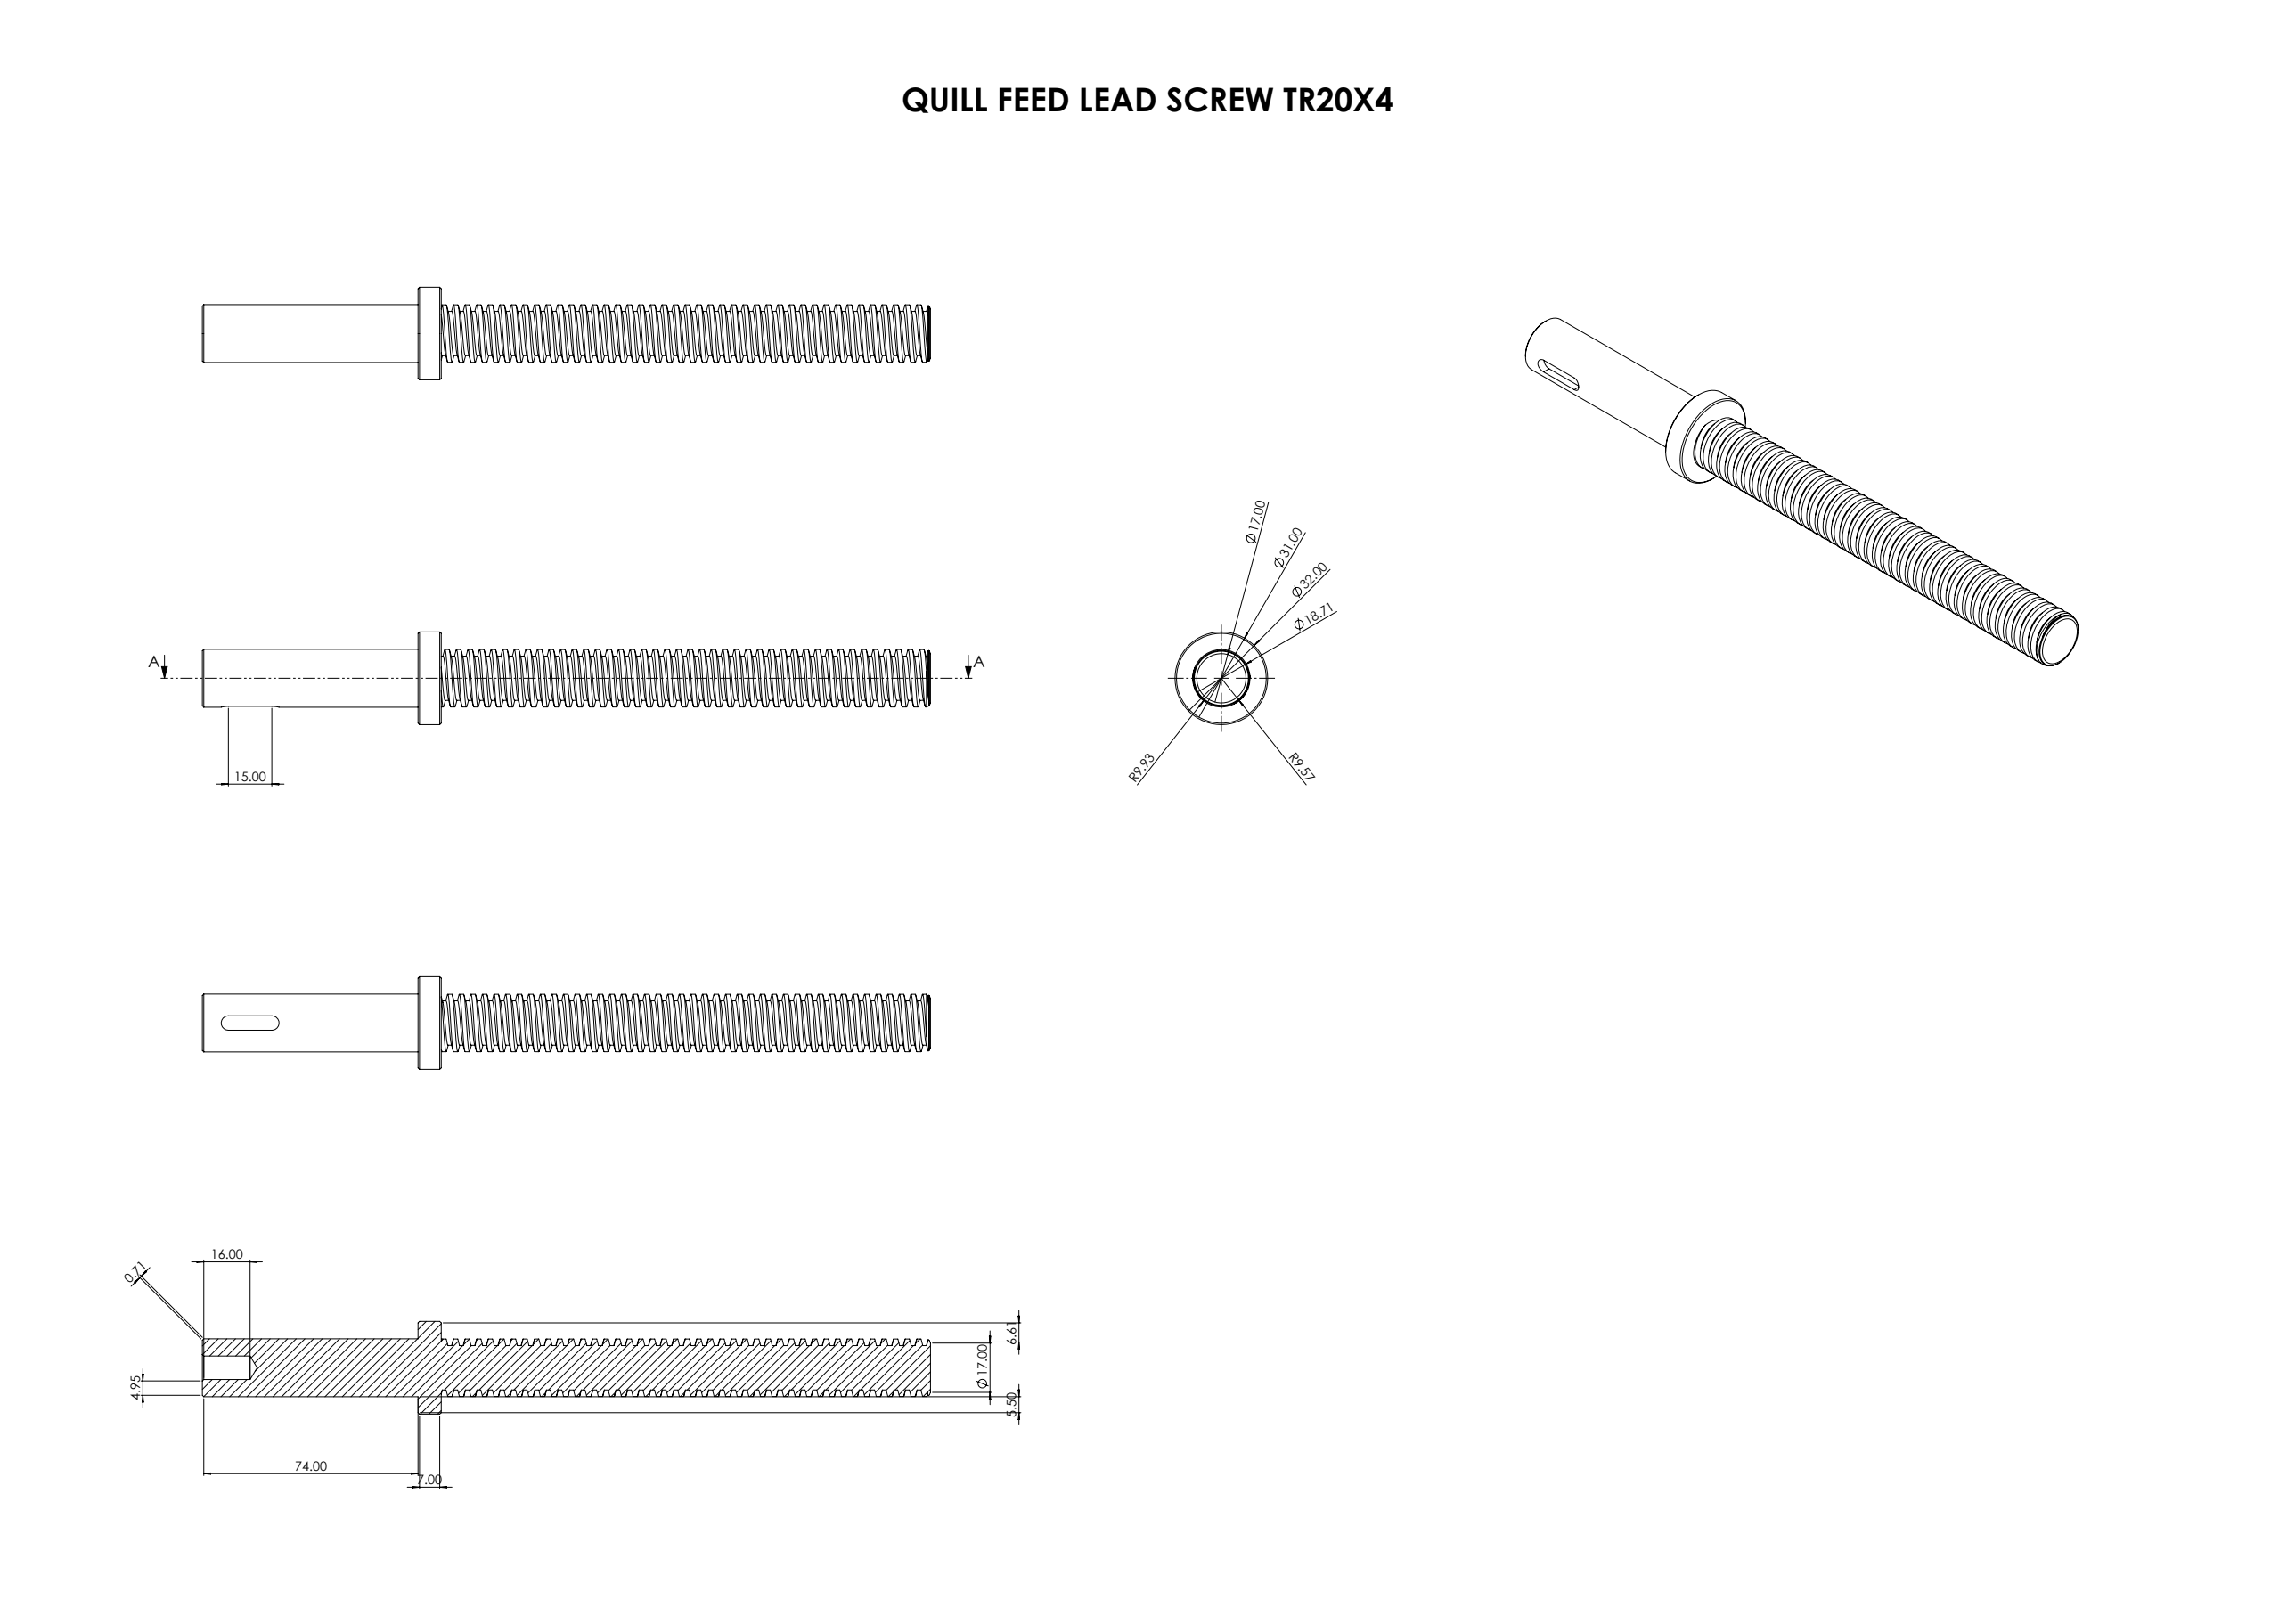
ISO-10303-21;
HEADER;
/* Generated by software containing ST-Developer
 * from STEP Tools, Inc. (www.steptools.com) 
 */

FILE_DESCRIPTION(
/* description */ (''),
/* implementation_level */ '2;1');

FILE_NAME(
/* name */ '05_Quill_Feed_Lead_Screw_Tr20x4.step',
/* time_stamp */ '2026-10-26T03:50:32-07:00',
/* author */ (''),
/* organization */ (''),
/* preprocessor_version */ 'ST-DEVELOPER v20.2',
/* originating_system */ 'Autodesk Translation Framework v15.15.0.0',
/* authorisation */ '');

FILE_SCHEMA (('AUTOMOTIVE_DESIGN { 1 0 10303 214 3 1 1 }'));
ENDSEC;

DATA;
#10=MECHANICAL_DESIGN_GEOMETRIC_PRESENTATION_REPRESENTATION('',(#1043),#76660);
#158=B_SPLINE_SURFACE_WITH_KNOTS('',3,3,((#45164,#45165,#45166,#45167,#45168,
#45169,#45170,#45171,#45172,#45173,#45174,#45175,#45176,#45177,#45178,#45179,
#45180,#45181,#45182,#45183,#45184,#45185,#45186,#45187,#45188,#45189,#45190,
#45191,#45192,#45193,#45194,#45195,#45196,#45197,#45198,#45199,#45200,#45201,
#45202,#45203,#45204,#45205,#45206,#45207,#45208,#45209,#45210,#45211,#45212,
#45213,#45214,#45215,#45216,#45217,#45218,#45219,#45220,#45221,#45222,#45223,
#45224,#45225,#45226,#45227,#45228,#45229,#45230,#45231,#45232,#45233,#45234,
#45235,#45236,#45237,#45238,#45239,#45240,#45241,#45242,#45243,#45244,#45245,
#45246,#45247,#45248,#45249,#45250,#45251,#45252,#45253,#45254,#45255,#45256,
#45257,#45258,#45259,#45260,#45261,#45262,#45263,#45264,#45265,#45266,#45267,
#45268,#45269,#45270,#45271,#45272,#45273,#45274,#45275,#45276,#45277,#45278,
#45279,#45280,#45281,#45282,#45283,#45284,#45285,#45286,#45287,#45288,#45289,
#45290,#45291,#45292,#45293,#45294,#45295,#45296,#45297,#45298,#45299,#45300,
#45301,#45302,#45303,#45304,#45305,#45306,#45307,#45308,#45309,#45310,#45311,
#45312,#45313,#45314,#45315,#45316,#45317,#45318,#45319,#45320,#45321,#45322,
#45323,#45324,#45325,#45326,#45327,#45328,#45329,#45330,#45331,#45332,#45333,
#45334,#45335,#45336,#45337,#45338,#45339,#45340,#45341,#45342,#45343,#45344,
#45345,#45346,#45347,#45348,#45349,#45350,#45351,#45352,#45353,#45354,#45355,
#45356,#45357,#45358,#45359,#45360,#45361,#45362,#45363,#45364,#45365,#45366,
#45367,#45368,#45369,#45370,#45371,#45372,#45373,#45374,#45375,#45376,#45377,
#45378,#45379,#45380,#45381,#45382,#45383,#45384,#45385,#45386,#45387,#45388,
#45389,#45390,#45391,#45392,#45393,#45394,#45395,#45396,#45397,#45398,#45399,
#45400,#45401,#45402,#45403,#45404,#45405,#45406,#45407,#45408,#45409,#45410,
#45411,#45412,#45413,#45414,#45415,#45416,#45417,#45418,#45419,#45420,#45421,
#45422,#45423,#45424,#45425,#45426,#45427,#45428,#45429,#45430,#45431,#45432,
#45433,#45434,#45435,#45436,#45437,#45438,#45439,#45440,#45441,#45442,#45443,
#45444,#45445,#45446,#45447,#45448,#45449,#45450,#45451,#45452,#45453,#45454,
#45455,#45456,#45457,#45458,#45459,#45460,#45461,#45462,#45463,#45464,#45465,
#45466,#45467,#45468,#45469,#45470,#45471,#45472,#45473,#45474,#45475,#45476,
#45477,#45478,#45479,#45480,#45481,#45482,#45483,#45484,#45485,#45486,#45487,
#45488,#45489,#45490,#45491,#45492,#45493,#45494,#45495,#45496,#45497,#45498,
#45499,#45500,#45501,#45502,#45503,#45504,#45505,#45506,#45507,#45508,#45509,
#45510,#45511,#45512,#45513,#45514,#45515,#45516,#45517,#45518,#45519,#45520,
#45521,#45522,#45523,#45524,#45525,#45526,#45527,#45528,#45529,#45530,#45531,
#45532,#45533,#45534,#45535,#45536,#45537,#45538,#45539,#45540,#45541,#45542,
#45543,#45544,#45545,#45546,#45547,#45548,#45549,#45550,#45551,#45552,#45553,
#45554,#45555,#45556,#45557,#45558,#45559,#45560,#45561,#45562,#45563,#45564,
#45565,#45566,#45567,#45568,#45569,#45570,#45571,#45572,#45573,#45574,#45575,
#45576,#45577,#45578,#45579,#45580,#45581,#45582,#45583,#45584,#45585,#45586,
#45587,#45588,#45589,#45590,#45591,#45592,#45593,#45594,#45595,#45596,#45597,
#45598,#45599,#45600,#45601,#45602,#45603,#45604,#45605,#45606,#45607,#45608,
#45609,#45610,#45611,#45612,#45613,#45614,#45615,#45616,#45617,#45618,#45619,
#45620,#45621,#45622,#45623,#45624,#45625,#45626,#45627,#45628,#45629,#45630,
#45631,#45632,#45633,#45634,#45635,#45636,#45637,#45638,#45639,#45640,#45641,
#45642,#45643,#45644,#45645,#45646,#45647,#45648,#45649,#45650,#45651,#45652,
#45653,#45654,#45655,#45656,#45657,#45658,#45659,#45660),(#45661,#45662,
#45663,#45664,#45665,#45666,#45667,#45668,#45669,#45670,#45671,#45672,#45673,
#45674,#45675,#45676,#45677,#45678,#45679,#45680,#45681,#45682,#45683,#45684,
#45685,#45686,#45687,#45688,#45689,#45690,#45691,#45692,#45693,#45694,#45695,
#45696,#45697,#45698,#45699,#45700,#45701,#45702,#45703,#45704,#45705,#45706,
#45707,#45708,#45709,#45710,#45711,#45712,#45713,#45714,#45715,#45716,#45717,
#45718,#45719,#45720,#45721,#45722,#45723,#45724,#45725,#45726,#45727,#45728,
#45729,#45730,#45731,#45732,#45733,#45734,#45735,#45736,#45737,#45738,#45739,
#45740,#45741,#45742,#45743,#45744,#45745,#45746,#45747,#45748,#45749,#45750,
#45751,#45752,#45753,#45754,#45755,#45756,#45757,#45758,#45759,#45760,#45761,
#45762,#45763,#45764,#45765,#45766,#45767,#45768,#45769,#45770,#45771,#45772,
#45773,#45774,#45775,#45776,#45777,#45778,#45779,#45780,#45781,#45782,#45783,
#45784,#45785,#45786,#45787,#45788,#45789,#45790,#45791,#45792,#45793,#45794,
#45795,#45796,#45797,#45798,#45799,#45800,#45801,#45802,#45803,#45804,#45805,
#45806,#45807,#45808,#45809,#45810,#45811,#45812,#45813,#45814,#45815,#45816,
#45817,#45818,#45819,#45820,#45821,#45822,#45823,#45824,#45825,#45826,#45827,
#45828,#45829,#45830,#45831,#45832,#45833,#45834,#45835,#45836,#45837,#45838,
#45839,#45840,#45841,#45842,#45843,#45844,#45845,#45846,#45847,#45848,#45849,
#45850,#45851,#45852,#45853,#45854,#45855,#45856,#45857,#45858,#45859,#45860,
#45861,#45862,#45863,#45864,#45865,#45866,#45867,#45868,#45869,#45870,#45871,
#45872,#45873,#45874,#45875,#45876,#45877,#45878,#45879,#45880,#45881,#45882,
#45883,#45884,#45885,#45886,#45887,#45888,#45889,#45890,#45891,#45892,#45893,
#45894,#45895,#45896,#45897,#45898,#45899,#45900,#45901,#45902,#45903,#45904,
#45905,#45906,#45907,#45908,#45909,#45910,#45911,#45912,#45913,#45914,#45915,
#45916,#45917,#45918,#45919,#45920,#45921,#45922,#45923,#45924,#45925,#45926,
#45927,#45928,#45929,#45930,#45931,#45932,#45933,#45934,#45935,#45936,#45937,
#45938,#45939,#45940,#45941,#45942,#45943,#45944,#45945,#45946,#45947,#45948,
#45949,#45950,#45951,#45952,#45953,#45954,#45955,#45956,#45957,#45958,#45959,
#45960,#45961,#45962,#45963,#45964,#45965,#45966,#45967,#45968,#45969,#45970,
#45971,#45972,#45973,#45974,#45975,#45976,#45977,#45978,#45979,#45980,#45981,
#45982,#45983,#45984,#45985,#45986,#45987,#45988,#45989,#45990,#45991,#45992,
#45993,#45994,#45995,#45996,#45997,#45998,#45999,#46000,#46001,#46002,#46003,
#46004,#46005,#46006,#46007,#46008,#46009,#46010,#46011,#46012,#46013,#46014,
#46015,#46016,#46017,#46018,#46019,#46020,#46021,#46022,#46023,#46024,#46025,
#46026,#46027,#46028,#46029,#46030,#46031,#46032,#46033,#46034,#46035,#46036,
#46037,#46038,#46039,#46040,#46041,#46042,#46043,#46044,#46045,#46046,#46047,
#46048,#46049,#46050,#46051,#46052,#46053,#46054,#46055,#46056,#46057,#46058,
#46059,#46060,#46061,#46062,#46063,#46064,#46065,#46066,#46067,#46068,#46069,
#46070,#46071,#46072,#46073,#46074,#46075,#46076,#46077,#46078,#46079,#46080,
#46081,#46082,#46083,#46084,#46085,#46086,#46087,#46088,#46089,#46090,#46091,
#46092,#46093,#46094,#46095,#46096,#46097,#46098,#46099,#46100,#46101,#46102,
#46103,#46104,#46105,#46106,#46107,#46108,#46109,#46110,#46111,#46112,#46113,
#46114,#46115,#46116,#46117,#46118,#46119,#46120,#46121,#46122,#46123,#46124,
#46125,#46126,#46127,#46128,#46129,#46130,#46131,#46132,#46133,#46134,#46135,
#46136,#46137,#46138,#46139,#46140,#46141,#46142,#46143,#46144,#46145,#46146,
#46147,#46148,#46149,#46150,#46151,#46152,#46153,#46154,#46155,#46156,#46157),
(#46158,#46159,#46160,#46161,#46162,#46163,#46164,#46165,#46166,#46167,
#46168,#46169,#46170,#46171,#46172,#46173,#46174,#46175,#46176,#46177,#46178,
#46179,#46180,#46181,#46182,#46183,#46184,#46185,#46186,#46187,#46188,#46189,
#46190,#46191,#46192,#46193,#46194,#46195,#46196,#46197,#46198,#46199,#46200,
#46201,#46202,#46203,#46204,#46205,#46206,#46207,#46208,#46209,#46210,#46211,
#46212,#46213,#46214,#46215,#46216,#46217,#46218,#46219,#46220,#46221,#46222,
#46223,#46224,#46225,#46226,#46227,#46228,#46229,#46230,#46231,#46232,#46233,
#46234,#46235,#46236,#46237,#46238,#46239,#46240,#46241,#46242,#46243,#46244,
#46245,#46246,#46247,#46248,#46249,#46250,#46251,#46252,#46253,#46254,#46255,
#46256,#46257,#46258,#46259,#46260,#46261,#46262,#46263,#46264,#46265,#46266,
#46267,#46268,#46269,#46270,#46271,#46272,#46273,#46274,#46275,#46276,#46277,
#46278,#46279,#46280,#46281,#46282,#46283,#46284,#46285,#46286,#46287,#46288,
#46289,#46290,#46291,#46292,#46293,#46294,#46295,#46296,#46297,#46298,#46299,
#46300,#46301,#46302,#46303,#46304,#46305,#46306,#46307,#46308,#46309,#46310,
#46311,#46312,#46313,#46314,#46315,#46316,#46317,#46318,#46319,#46320,#46321,
#46322,#46323,#46324,#46325,#46326,#46327,#46328,#46329,#46330,#46331,#46332,
#46333,#46334,#46335,#46336,#46337,#46338,#46339,#46340,#46341,#46342,#46343,
#46344,#46345,#46346,#46347,#46348,#46349,#46350,#46351,#46352,#46353,#46354,
#46355,#46356,#46357,#46358,#46359,#46360,#46361,#46362,#46363,#46364,#46365,
#46366,#46367,#46368,#46369,#46370,#46371,#46372,#46373,#46374,#46375,#46376,
#46377,#46378,#46379,#46380,#46381,#46382,#46383,#46384,#46385,#46386,#46387,
#46388,#46389,#46390,#46391,#46392,#46393,#46394,#46395,#46396,#46397,#46398,
#46399,#46400,#46401,#46402,#46403,#46404,#46405,#46406,#46407,#46408,#46409,
#46410,#46411,#46412,#46413,#46414,#46415,#46416,#46417,#46418,#46419,#46420,
#46421,#46422,#46423,#46424,#46425,#46426,#46427,#46428,#46429,#46430,#46431,
#46432,#46433,#46434,#46435,#46436,#46437,#46438,#46439,#46440,#46441,#46442,
#46443,#46444,#46445,#46446,#46447,#46448,#46449,#46450,#46451,#46452,#46453,
#46454,#46455,#46456,#46457,#46458,#46459,#46460,#46461,#46462,#46463,#46464,
#46465,#46466,#46467,#46468,#46469,#46470,#46471,#46472,#46473,#46474,#46475,
#46476,#46477,#46478,#46479,#46480,#46481,#46482,#46483,#46484,#46485,#46486,
#46487,#46488,#46489,#46490,#46491,#46492,#46493,#46494,#46495,#46496,#46497,
#46498,#46499,#46500,#46501,#46502,#46503,#46504,#46505,#46506,#46507,#46508,
#46509,#46510,#46511,#46512,#46513,#46514,#46515,#46516,#46517,#46518,#46519,
#46520,#46521,#46522,#46523,#46524,#46525,#46526,#46527,#46528,#46529,#46530,
#46531,#46532,#46533,#46534,#46535,#46536,#46537,#46538,#46539,#46540,#46541,
#46542,#46543,#46544,#46545,#46546,#46547,#46548,#46549,#46550,#46551,#46552,
#46553,#46554,#46555,#46556,#46557,#46558,#46559,#46560,#46561,#46562,#46563,
#46564,#46565,#46566,#46567,#46568,#46569,#46570,#46571,#46572,#46573,#46574,
#46575,#46576,#46577,#46578,#46579,#46580,#46581,#46582,#46583,#46584,#46585,
#46586,#46587,#46588,#46589,#46590,#46591,#46592,#46593,#46594,#46595,#46596,
#46597,#46598,#46599,#46600,#46601,#46602,#46603,#46604,#46605,#46606,#46607,
#46608,#46609,#46610,#46611,#46612,#46613,#46614,#46615,#46616,#46617,#46618,
#46619,#46620,#46621,#46622,#46623,#46624,#46625,#46626,#46627,#46628,#46629,
#46630,#46631,#46632,#46633,#46634,#46635,#46636,#46637,#46638,#46639,#46640,
#46641,#46642,#46643,#46644,#46645,#46646,#46647,#46648,#46649,#46650,#46651,
#46652,#46653,#46654),(#46655,#46656,#46657,#46658,#46659,#46660,#46661,
#46662,#46663,#46664,#46665,#46666,#46667,#46668,#46669,#46670,#46671,#46672,
#46673,#46674,#46675,#46676,#46677,#46678,#46679,#46680,#46681,#46682,#46683,
#46684,#46685,#46686,#46687,#46688,#46689,#46690,#46691,#46692,#46693,#46694,
#46695,#46696,#46697,#46698,#46699,#46700,#46701,#46702,#46703,#46704,#46705,
#46706,#46707,#46708,#46709,#46710,#46711,#46712,#46713,#46714,#46715,#46716,
#46717,#46718,#46719,#46720,#46721,#46722,#46723,#46724,#46725,#46726,#46727,
#46728,#46729,#46730,#46731,#46732,#46733,#46734,#46735,#46736,#46737,#46738,
#46739,#46740,#46741,#46742,#46743,#46744,#46745,#46746,#46747,#46748,#46749,
#46750,#46751,#46752,#46753,#46754,#46755,#46756,#46757,#46758,#46759,#46760,
#46761,#46762,#46763,#46764,#46765,#46766,#46767,#46768,#46769,#46770,#46771,
#46772,#46773,#46774,#46775,#46776,#46777,#46778,#46779,#46780,#46781,#46782,
#46783,#46784,#46785,#46786,#46787,#46788,#46789,#46790,#46791,#46792,#46793,
#46794,#46795,#46796,#46797,#46798,#46799,#46800,#46801,#46802,#46803,#46804,
#46805,#46806,#46807,#46808,#46809,#46810,#46811,#46812,#46813,#46814,#46815,
#46816,#46817,#46818,#46819,#46820,#46821,#46822,#46823,#46824,#46825,#46826,
#46827,#46828,#46829,#46830,#46831,#46832,#46833,#46834,#46835,#46836,#46837,
#46838,#46839,#46840,#46841,#46842,#46843,#46844,#46845,#46846,#46847,#46848,
#46849,#46850,#46851,#46852,#46853,#46854,#46855,#46856,#46857,#46858,#46859,
#46860,#46861,#46862,#46863,#46864,#46865,#46866,#46867,#46868,#46869,#46870,
#46871,#46872,#46873,#46874,#46875,#46876,#46877,#46878,#46879,#46880,#46881,
#46882,#46883,#46884,#46885,#46886,#46887,#46888,#46889,#46890,#46891,#46892,
#46893,#46894,#46895,#46896,#46897,#46898,#46899,#46900,#46901,#46902,#46903,
#46904,#46905,#46906,#46907,#46908,#46909,#46910,#46911,#46912,#46913,#46914,
#46915,#46916,#46917,#46918,#46919,#46920,#46921,#46922,#46923,#46924,#46925,
#46926,#46927,#46928,#46929,#46930,#46931,#46932,#46933,#46934,#46935,#46936,
#46937,#46938,#46939,#46940,#46941,#46942,#46943,#46944,#46945,#46946,#46947,
#46948,#46949,#46950,#46951,#46952,#46953,#46954,#46955,#46956,#46957,#46958,
#46959,#46960,#46961,#46962,#46963,#46964,#46965,#46966,#46967,#46968,#46969,
#46970,#46971,#46972,#46973,#46974,#46975,#46976,#46977,#46978,#46979,#46980,
#46981,#46982,#46983,#46984,#46985,#46986,#46987,#46988,#46989,#46990,#46991,
#46992,#46993,#46994,#46995,#46996,#46997,#46998,#46999,#47000,#47001,#47002,
#47003,#47004,#47005,#47006,#47007,#47008,#47009,#47010,#47011,#47012,#47013,
#47014,#47015,#47016,#47017,#47018,#47019,#47020,#47021,#47022,#47023,#47024,
#47025,#47026,#47027,#47028,#47029,#47030,#47031,#47032,#47033,#47034,#47035,
#47036,#47037,#47038,#47039,#47040,#47041,#47042,#47043,#47044,#47045,#47046,
#47047,#47048,#47049,#47050,#47051,#47052,#47053,#47054,#47055,#47056,#47057,
#47058,#47059,#47060,#47061,#47062,#47063,#47064,#47065,#47066,#47067,#47068,
#47069,#47070,#47071,#47072,#47073,#47074,#47075,#47076,#47077,#47078,#47079,
#47080,#47081,#47082,#47083,#47084,#47085,#47086,#47087,#47088,#47089,#47090,
#47091,#47092,#47093,#47094,#47095,#47096,#47097,#47098,#47099,#47100,#47101,
#47102,#47103,#47104,#47105,#47106,#47107,#47108,#47109,#47110,#47111,#47112,
#47113,#47114,#47115,#47116,#47117,#47118,#47119,#47120,#47121,#47122,#47123,
#47124,#47125,#47126,#47127,#47128,#47129,#47130,#47131,#47132,#47133,#47134,
#47135,#47136,#47137,#47138,#47139,#47140,#47141,#47142,#47143,#47144,#47145,
#47146,#47147,#47148,#47149,#47150,#47151)),.UNSPECIFIED.,.F.,.F.,.F.,(4,
4),(4,1,1,1,1,1,1,1,1,1,1,1,1,1,1,1,1,1,1,1,1,1,1,1,1,1,1,1,1,1,1,1,1,1,
1,1,1,1,1,1,1,1,1,1,1,1,1,1,1,1,1,1,1,1,1,1,1,1,1,1,1,1,1,1,1,1,1,1,1,1,
1,1,1,1,1,1,1,1,1,1,1,1,1,1,1,1,1,1,1,1,1,1,1,1,1,1,1,1,1,1,1,1,1,1,1,1,
1,1,1,1,1,1,1,1,1,1,1,1,1,1,1,1,1,1,1,1,1,1,1,1,1,1,1,1,1,1,1,1,1,1,1,1,
1,1,1,1,1,1,1,1,1,1,1,1,1,1,1,1,1,1,1,1,1,1,1,1,1,1,1,1,1,1,1,1,1,1,1,1,
1,1,1,1,1,1,1,1,1,1,1,1,1,1,1,1,1,1,1,1,1,1,1,1,1,1,1,1,1,1,1,1,1,1,1,1,
1,1,1,1,1,1,1,1,1,1,1,1,1,1,1,1,1,1,1,1,1,1,1,1,1,1,1,1,1,1,1,1,1,1,1,1,
1,1,1,1,1,1,1,1,1,1,1,1,1,1,1,1,1,1,1,1,1,1,1,1,1,1,1,1,1,1,1,1,1,1,1,1,
1,1,1,1,1,1,1,1,1,1,1,1,1,1,1,1,1,1,1,1,1,1,1,1,1,1,1,1,1,1,1,1,1,1,1,1,
1,1,1,1,1,1,1,1,1,1,1,1,1,1,1,1,1,1,1,1,1,1,1,1,1,1,1,1,1,1,1,1,1,1,1,1,
1,1,1,1,1,1,1,1,1,1,1,1,1,1,1,1,1,1,1,1,1,1,1,1,1,1,1,1,1,1,1,1,1,1,1,1,
1,1,1,1,1,1,1,1,1,1,1,1,1,1,1,1,1,1,1,1,1,1,1,1,1,1,1,1,1,1,1,1,1,1,1,1,
1,1,1,1,1,1,1,1,1,1,1,1,1,1,1,1,1,1,1,1,1,1,1,1,1,1,1,1,1,1,1,1,1,1,1,1,
1,1,1,1,1,1,1,1,1,1,1,1,1,1,1,1,1,1,1,1,1,1,1,1,1,1,1,1,4),(-1.54457385216123E-14,
0.236198260560645),(12.043305083964,12.5421366924057,13.0409683008475,13.5397999092893,
14.0386315177311,14.5374631261729,15.0362947346147,15.5351263430564,16.0339579514982,
17.0316211683818,17.5304527768236,18.0292843852654,18.5281159937072,19.0269476021489,
19.5257792105907,20.0246108190325,20.5234424274743,21.0222740359161,21.5211056443579,
22.0199372527997,22.5187688612414,23.0176004696832,24.0152636865668,24.5140952950086,
25.0129269034504,25.5117585118921,26.0105901203339,26.5094217287757,27.0082533372175,
27.5070849456593,28.0059165541011,28.5047481625429,29.0035797709846,29.5024113794264,
30.0012429878682,30.9989062047518,31.4977378131936,31.9965694216353,32.4954010300771,
32.9942326385189,33.4930642469607,33.9918958554025,34.4907274638443,34.9895590722861,
35.4883906807278,35.9872222891696,36.4860538976114,36.9848855060532,37.9825487229368,
38.4813803313785,38.9802119398203,39.4790435482621,39.9778751567039,40.4767067651457,
40.9755383735875,41.4743699820293,41.973201590471,42.4720331989128,42.9708648073546,
43.4696964157964,43.9685280242382,44.9661912411217,45.4650228495635,45.9638544580053,
46.4626860664471,46.9615176748889,47.4603492833307,47.9591808917725,48.4580125002142,
48.956844108656,49.4556757170978,49.9545073255396,50.4533389339814,50.9521705424232,
51.9498337593067,52.4486653677485,52.9474969761903,53.4463285846321,53.9451601930739,
54.4439918015157,54.9428234099574,55.4416550183992,55.940486626841,56.4393182352828,
56.9381498437246,57.4369814521664,57.9358130606082,58.9334762774917,59.4323078859335,
59.9311394943753,60.4299711028171,60.9288027112589,61.4276343197006,61.9264659281424,
62.4252975365842,62.924129145026,63.4229607534678,63.9217923619096,64.4206239703514,
64.9194555787931,65.9171187956767,66.4159504041185,66.9147820125603,67.4136136210021,
67.9124452294438,68.4112768378856,68.9101084463274,69.4089400547692,69.907771663211,
70.4066032716528,70.9054348800946,71.4042664885363,71.9030980969781,72.9007613138617,
73.3995929223035,73.8984245307453,74.397256139187,74.8960877476288,75.3949193560706,
75.8937509645124,76.3925825729542,76.891414181396,77.3902457898378,77.8890773982795,
78.3879090067213,78.8867406151631,79.8844038320467,80.3832354404885,80.8820670489303,
81.380898657372,81.8797302658138,82.3785618742556,82.8773934826974,83.3762250911392,
83.875056699581,84.3738883080227,84.8727199164645,85.3715515249063,85.8703831333481,
86.8680463502317,87.3668779586735,87.8657095671152,88.364541175557,88.8633727839988,
89.3622043924406,89.8610360008824,90.3598676093242,90.8586992177659,91.3575308262077,
91.8563624346495,92.3551940430913,92.8540256515331,93.8516888684167,94.3505204768584,
94.8493520853002,95.348183693742,95.8470153021838,96.3458469106256,96.8446785190674,
97.3435101275091,97.8423417359509,98.3411733443927,98.8400049528345,99.3388365612763,
99.8376681697181,100.835331386602,101.334162995043,101.832994603485,102.331826211927,
102.830657820369,103.329489428811,103.828321037252,104.327152645694,104.825984254136,
105.324815862578,105.823647471019,106.322479079461,106.821310687903,107.818973904787,
108.317805513228,108.81663712167,109.315468730112,109.814300338554,110.313131946996,
110.811963555437,111.310795163879,111.809626772321,112.308458380763,112.807289989204,
113.306121597646,113.804953206088,114.802616422972,115.301448031413,115.800279639855,
116.299111248297,116.797942856739,117.296774465181,117.795606073622,118.294437682064,
118.793269290506,119.292100898948,119.790932507389,120.289764115831,120.788595724273,
121.786258941157,122.285090549598,122.78392215804,123.282753766482,123.781585374924,
124.280416983366,124.779248591807,125.278080200249,125.776911808691,126.275743417133,
126.774575025574,127.273406634016,127.772238242458,128.769901459342,129.268733067783,
129.767564676225,130.266396284667,130.765227893109,131.26405950155,131.762891109992,
132.261722718434,132.760554326876,133.259385935318,133.758217543759,134.257049152201,
134.755880760643,135.753543977527,136.252375585968,136.75120719441,137.250038802852,
137.748870411294,138.247702019735,138.746533628177,139.245365236619,139.744196845061,
140.243028453503,140.741860061944,141.240691670386,141.739523278828,142.737186495712,
143.236018104153,143.734849712595,144.233681321037,144.732512929479,145.231344537921,
145.730176146362,146.229007754804,146.727839363246,147.725502580129,148.224334188571,
148.723165797013,149.221997405455,149.720829013897,150.219660622338,150.71849223078,
151.217323839222,151.716155447664,152.214987056105,152.713818664547,153.212650272989,
153.711481881431,154.709145098314,155.207976706756,155.706808315198,156.20563992364,
156.704471532082,157.203303140523,157.702134748965,158.200966357407,158.699797965849,
159.19862957429,159.697461182732,160.196292791174,160.695124399616,161.692787616499,
162.191619224941,162.690450833383,163.189282441825,163.688114050267,164.186945658708,
164.68577726715,165.184608875592,165.683440484034,166.182272092475,166.681103700917,
167.179935309359,167.678766917801,168.676430134684,169.175261743126,169.674093351568,
170.17292496001,170.671756568452,171.170588176893,171.669419785335,172.168251393777,
172.667083002219,173.16591461066,173.664746219102,174.163577827544,174.662409435986,
175.660072652869,176.158904261311,176.657735869753,177.156567478195,177.655399086636,
178.154230695078,178.65306230352,179.151893911962,179.650725520404,180.149557128845,
180.648388737287,181.147220345729,181.646051954171,182.643715171054,183.142546779496,
183.641378387938,184.14020999638,184.639041604821,185.137873213263,185.636704821705,
186.135536430147,186.634368038589,187.13319964703,187.632031255472,188.130862863914,
188.629694472356,189.627357689239,190.126189297681,190.625020906123,191.123852514565,
191.622684123006,192.121515731448,192.62034733989,193.119178948332,193.618010556774,
194.116842165215,194.615673773657,195.114505382099,195.613336990541,196.611000207424,
197.109831815866,197.608663424308,198.10749503275,198.606326641191,199.105158249633,
199.603989858075,200.102821466517,200.601653074959,201.1004846834,201.599316291842,
202.098147900284,202.596979508726,203.594642725609,204.093474334051,204.592305942493,
205.091137550935,205.589969159376,206.088800767818,206.58763237626,207.086463984702,
207.585295593144,208.084127201585,208.582958810027,209.081790418469,209.580622026911,
210.578285243794,211.077116852236,211.575948460678,212.07478006912,212.573611677561,
213.072443286003,213.571274894445,214.070106502887,214.568938111329,215.06776971977,
215.566601328212,216.065432936654,216.564264545096,217.561927761979,218.060759370421,
218.559590978863,219.058422587305,219.557254195746,220.056085804188,220.55491741263,
221.053749021072,221.552580629514,222.051412237955,222.550243846397,223.049075454839,
223.547907063281,224.545570280164,225.044401888606,225.543233497048,226.04206510549,
226.540896713931,227.039728322373,227.538559930815,228.037391539257,228.536223147699,
229.03505475614,229.533886364582,230.032717973024,230.531549581466,231.529212798349,
232.028044406791,232.526876015233,233.025707623675,233.524539232116,234.023370840558,
234.522202449,235.021034057442,235.519865665884,236.018697274325,236.517528882767,
237.016360491209,237.515192099651,238.512855316534,239.011686924976,239.510518533418,
240.00935014186,240.508181750301,241.007013358743,241.505844967185,242.004676575627,
242.503508184069,243.00233979251,243.501171400952,244.000003009394,244.498834617836,
245.496497834719,245.995329443161,246.494161051603,246.992992660045,247.491824268486,
247.990655876928,248.48948748537,248.988319093812,249.487150702254,249.985982310695,
250.484813919137,250.983645527579,251.482477136021,252.480140352904,252.978971961346,
253.477803569788,253.97663517823,254.475466786671,254.974298395113,255.473130003555,
255.971961611997,256.470793220438,256.96962482888,257.468456437322,257.967288045764,
258.466119654206,259.463782871089,259.962614479531,260.461446087973,260.960277696415,
261.459109304856,261.957940913298,262.45677252174,262.955604130182,263.454435738623,
263.953267347065,264.452098955507,264.950930563949,265.449762172391,266.447425389274,
266.946256997716,267.445088606158,267.9439202146,268.442751823041,268.941583431483,
269.440415039925,269.939246648367,270.438078256808,270.93690986525,271.435741473692,
271.934573082134,272.433404690576,273.431067907459,273.929899515901,274.428731124343,
274.927562732785,275.426394341226,275.925225949668,276.42405755811,276.922889166552,
277.421720774993),.UNSPECIFIED.);
#159=B_SPLINE_SURFACE_WITH_KNOTS('',3,3,((#47328,#47329,#47330,#47331,#47332,
#47333,#47334,#47335,#47336,#47337,#47338,#47339,#47340,#47341,#47342,#47343,
#47344,#47345,#47346,#47347,#47348,#47349,#47350,#47351,#47352,#47353,#47354,
#47355,#47356,#47357,#47358,#47359,#47360,#47361,#47362,#47363,#47364,#47365,
#47366,#47367,#47368,#47369,#47370,#47371,#47372,#47373,#47374,#47375,#47376,
#47377,#47378,#47379,#47380,#47381,#47382,#47383,#47384,#47385,#47386,#47387,
#47388,#47389,#47390,#47391,#47392,#47393,#47394,#47395,#47396,#47397,#47398,
#47399,#47400,#47401,#47402,#47403,#47404,#47405,#47406,#47407,#47408,#47409,
#47410,#47411,#47412,#47413,#47414,#47415,#47416,#47417,#47418,#47419,#47420,
#47421,#47422,#47423,#47424,#47425,#47426,#47427,#47428,#47429,#47430,#47431,
#47432,#47433,#47434,#47435,#47436,#47437,#47438,#47439,#47440,#47441,#47442,
#47443,#47444,#47445,#47446,#47447,#47448,#47449,#47450,#47451,#47452,#47453,
#47454,#47455,#47456,#47457,#47458,#47459,#47460,#47461,#47462,#47463,#47464,
#47465,#47466,#47467,#47468,#47469,#47470,#47471,#47472,#47473,#47474,#47475,
#47476,#47477,#47478,#47479,#47480,#47481,#47482,#47483,#47484,#47485,#47486,
#47487,#47488,#47489,#47490,#47491,#47492,#47493,#47494,#47495,#47496,#47497,
#47498,#47499,#47500,#47501,#47502,#47503,#47504,#47505,#47506,#47507,#47508,
#47509,#47510,#47511,#47512,#47513,#47514,#47515,#47516,#47517,#47518,#47519,
#47520,#47521,#47522,#47523,#47524,#47525,#47526,#47527,#47528,#47529,#47530,
#47531,#47532,#47533,#47534,#47535,#47536,#47537,#47538,#47539,#47540,#47541,
#47542,#47543,#47544,#47545,#47546,#47547,#47548,#47549,#47550,#47551,#47552,
#47553,#47554,#47555,#47556,#47557,#47558,#47559,#47560,#47561,#47562,#47563,
#47564,#47565,#47566,#47567,#47568,#47569,#47570,#47571,#47572,#47573,#47574,
#47575,#47576,#47577,#47578,#47579,#47580,#47581,#47582,#47583,#47584,#47585,
#47586,#47587,#47588,#47589,#47590,#47591,#47592,#47593,#47594,#47595,#47596,
#47597,#47598,#47599,#47600,#47601,#47602,#47603,#47604,#47605,#47606,#47607,
#47608,#47609,#47610,#47611,#47612,#47613,#47614,#47615,#47616,#47617,#47618,
#47619,#47620,#47621,#47622,#47623,#47624,#47625,#47626,#47627,#47628,#47629,
#47630,#47631,#47632,#47633,#47634,#47635,#47636,#47637,#47638,#47639,#47640,
#47641,#47642,#47643,#47644,#47645,#47646,#47647,#47648,#47649,#47650,#47651,
#47652,#47653,#47654,#47655,#47656,#47657,#47658,#47659,#47660,#47661,#47662,
#47663,#47664,#47665,#47666,#47667,#47668,#47669,#47670,#47671,#47672,#47673,
#47674,#47675,#47676,#47677,#47678,#47679,#47680,#47681,#47682,#47683,#47684,
#47685,#47686,#47687,#47688,#47689,#47690,#47691,#47692,#47693,#47694,#47695,
#47696,#47697,#47698,#47699,#47700,#47701,#47702,#47703,#47704,#47705,#47706,
#47707,#47708,#47709,#47710,#47711,#47712,#47713,#47714,#47715,#47716,#47717,
#47718,#47719,#47720,#47721,#47722,#47723,#47724,#47725,#47726,#47727,#47728,
#47729,#47730,#47731,#47732,#47733,#47734,#47735,#47736,#47737,#47738,#47739,
#47740,#47741,#47742,#47743,#47744,#47745,#47746,#47747,#47748,#47749,#47750,
#47751,#47752,#47753,#47754,#47755,#47756,#47757,#47758,#47759,#47760,#47761,
#47762,#47763,#47764,#47765,#47766,#47767,#47768,#47769,#47770,#47771,#47772,
#47773,#47774,#47775,#47776,#47777,#47778,#47779,#47780,#47781,#47782,#47783,
#47784,#47785,#47786,#47787,#47788,#47789,#47790,#47791,#47792,#47793,#47794,
#47795,#47796,#47797,#47798,#47799,#47800,#47801,#47802,#47803,#47804,#47805,
#47806,#47807,#47808,#47809,#47810,#47811,#47812,#47813,#47814,#47815,#47816,
#47817,#47818,#47819,#47820,#47821,#47822,#47823,#47824,#47825,#47826,#47827,
#47828,#47829,#47830,#47831,#47832,#47833,#47834,#47835,#47836,#47837,#47838,
#47839,#47840,#47841,#47842,#47843,#47844,#47845,#47846,#47847,#47848,#47849,
#47850,#47851,#47852,#47853,#47854,#47855,#47856,#47857,#47858),(#47859,
#47860,#47861,#47862,#47863,#47864,#47865,#47866,#47867,#47868,#47869,#47870,
#47871,#47872,#47873,#47874,#47875,#47876,#47877,#47878,#47879,#47880,#47881,
#47882,#47883,#47884,#47885,#47886,#47887,#47888,#47889,#47890,#47891,#47892,
#47893,#47894,#47895,#47896,#47897,#47898,#47899,#47900,#47901,#47902,#47903,
#47904,#47905,#47906,#47907,#47908,#47909,#47910,#47911,#47912,#47913,#47914,
#47915,#47916,#47917,#47918,#47919,#47920,#47921,#47922,#47923,#47924,#47925,
#47926,#47927,#47928,#47929,#47930,#47931,#47932,#47933,#47934,#47935,#47936,
#47937,#47938,#47939,#47940,#47941,#47942,#47943,#47944,#47945,#47946,#47947,
#47948,#47949,#47950,#47951,#47952,#47953,#47954,#47955,#47956,#47957,#47958,
#47959,#47960,#47961,#47962,#47963,#47964,#47965,#47966,#47967,#47968,#47969,
#47970,#47971,#47972,#47973,#47974,#47975,#47976,#47977,#47978,#47979,#47980,
#47981,#47982,#47983,#47984,#47985,#47986,#47987,#47988,#47989,#47990,#47991,
#47992,#47993,#47994,#47995,#47996,#47997,#47998,#47999,#48000,#48001,#48002,
#48003,#48004,#48005,#48006,#48007,#48008,#48009,#48010,#48011,#48012,#48013,
#48014,#48015,#48016,#48017,#48018,#48019,#48020,#48021,#48022,#48023,#48024,
#48025,#48026,#48027,#48028,#48029,#48030,#48031,#48032,#48033,#48034,#48035,
#48036,#48037,#48038,#48039,#48040,#48041,#48042,#48043,#48044,#48045,#48046,
#48047,#48048,#48049,#48050,#48051,#48052,#48053,#48054,#48055,#48056,#48057,
#48058,#48059,#48060,#48061,#48062,#48063,#48064,#48065,#48066,#48067,#48068,
#48069,#48070,#48071,#48072,#48073,#48074,#48075,#48076,#48077,#48078,#48079,
#48080,#48081,#48082,#48083,#48084,#48085,#48086,#48087,#48088,#48089,#48090,
#48091,#48092,#48093,#48094,#48095,#48096,#48097,#48098,#48099,#48100,#48101,
#48102,#48103,#48104,#48105,#48106,#48107,#48108,#48109,#48110,#48111,#48112,
#48113,#48114,#48115,#48116,#48117,#48118,#48119,#48120,#48121,#48122,#48123,
#48124,#48125,#48126,#48127,#48128,#48129,#48130,#48131,#48132,#48133,#48134,
#48135,#48136,#48137,#48138,#48139,#48140,#48141,#48142,#48143,#48144,#48145,
#48146,#48147,#48148,#48149,#48150,#48151,#48152,#48153,#48154,#48155,#48156,
#48157,#48158,#48159,#48160,#48161,#48162,#48163,#48164,#48165,#48166,#48167,
#48168,#48169,#48170,#48171,#48172,#48173,#48174,#48175,#48176,#48177,#48178,
#48179,#48180,#48181,#48182,#48183,#48184,#48185,#48186,#48187,#48188,#48189,
#48190,#48191,#48192,#48193,#48194,#48195,#48196,#48197,#48198,#48199,#48200,
#48201,#48202,#48203,#48204,#48205,#48206,#48207,#48208,#48209,#48210,#48211,
#48212,#48213,#48214,#48215,#48216,#48217,#48218,#48219,#48220,#48221,#48222,
#48223,#48224,#48225,#48226,#48227,#48228,#48229,#48230,#48231,#48232,#48233,
#48234,#48235,#48236,#48237,#48238,#48239,#48240,#48241,#48242,#48243,#48244,
#48245,#48246,#48247,#48248,#48249,#48250,#48251,#48252,#48253,#48254,#48255,
#48256,#48257,#48258,#48259,#48260,#48261,#48262,#48263,#48264,#48265,#48266,
#48267,#48268,#48269,#48270,#48271,#48272,#48273,#48274,#48275,#48276,#48277,
#48278,#48279,#48280,#48281,#48282,#48283,#48284,#48285,#48286,#48287,#48288,
#48289,#48290,#48291,#48292,#48293,#48294,#48295,#48296,#48297,#48298,#48299,
#48300,#48301,#48302,#48303,#48304,#48305,#48306,#48307,#48308,#48309,#48310,
#48311,#48312,#48313,#48314,#48315,#48316,#48317,#48318,#48319,#48320,#48321,
#48322,#48323,#48324,#48325,#48326,#48327,#48328,#48329,#48330,#48331,#48332,
#48333,#48334,#48335,#48336,#48337,#48338,#48339,#48340,#48341,#48342,#48343,
#48344,#48345,#48346,#48347,#48348,#48349,#48350,#48351,#48352,#48353,#48354,
#48355,#48356,#48357,#48358,#48359,#48360,#48361,#48362,#48363,#48364,#48365,
#48366,#48367,#48368,#48369,#48370,#48371,#48372,#48373,#48374,#48375,#48376,
#48377,#48378,#48379,#48380,#48381,#48382,#48383,#48384,#48385,#48386,#48387,
#48388,#48389),(#48390,#48391,#48392,#48393,#48394,#48395,#48396,#48397,
#48398,#48399,#48400,#48401,#48402,#48403,#48404,#48405,#48406,#48407,#48408,
#48409,#48410,#48411,#48412,#48413,#48414,#48415,#48416,#48417,#48418,#48419,
#48420,#48421,#48422,#48423,#48424,#48425,#48426,#48427,#48428,#48429,#48430,
#48431,#48432,#48433,#48434,#48435,#48436,#48437,#48438,#48439,#48440,#48441,
#48442,#48443,#48444,#48445,#48446,#48447,#48448,#48449,#48450,#48451,#48452,
#48453,#48454,#48455,#48456,#48457,#48458,#48459,#48460,#48461,#48462,#48463,
#48464,#48465,#48466,#48467,#48468,#48469,#48470,#48471,#48472,#48473,#48474,
#48475,#48476,#48477,#48478,#48479,#48480,#48481,#48482,#48483,#48484,#48485,
#48486,#48487,#48488,#48489,#48490,#48491,#48492,#48493,#48494,#48495,#48496,
#48497,#48498,#48499,#48500,#48501,#48502,#48503,#48504,#48505,#48506,#48507,
#48508,#48509,#48510,#48511,#48512,#48513,#48514,#48515,#48516,#48517,#48518,
#48519,#48520,#48521,#48522,#48523,#48524,#48525,#48526,#48527,#48528,#48529,
#48530,#48531,#48532,#48533,#48534,#48535,#48536,#48537,#48538,#48539,#48540,
#48541,#48542,#48543,#48544,#48545,#48546,#48547,#48548,#48549,#48550,#48551,
#48552,#48553,#48554,#48555,#48556,#48557,#48558,#48559,#48560,#48561,#48562,
#48563,#48564,#48565,#48566,#48567,#48568,#48569,#48570,#48571,#48572,#48573,
#48574,#48575,#48576,#48577,#48578,#48579,#48580,#48581,#48582,#48583,#48584,
#48585,#48586,#48587,#48588,#48589,#48590,#48591,#48592,#48593,#48594,#48595,
#48596,#48597,#48598,#48599,#48600,#48601,#48602,#48603,#48604,#48605,#48606,
#48607,#48608,#48609,#48610,#48611,#48612,#48613,#48614,#48615,#48616,#48617,
#48618,#48619,#48620,#48621,#48622,#48623,#48624,#48625,#48626,#48627,#48628,
#48629,#48630,#48631,#48632,#48633,#48634,#48635,#48636,#48637,#48638,#48639,
#48640,#48641,#48642,#48643,#48644,#48645,#48646,#48647,#48648,#48649,#48650,
#48651,#48652,#48653,#48654,#48655,#48656,#48657,#48658,#48659,#48660,#48661,
#48662,#48663,#48664,#48665,#48666,#48667,#48668,#48669,#48670,#48671,#48672,
#48673,#48674,#48675,#48676,#48677,#48678,#48679,#48680,#48681,#48682,#48683,
#48684,#48685,#48686,#48687,#48688,#48689,#48690,#48691,#48692,#48693,#48694,
#48695,#48696,#48697,#48698,#48699,#48700,#48701,#48702,#48703,#48704,#48705,
#48706,#48707,#48708,#48709,#48710,#48711,#48712,#48713,#48714,#48715,#48716,
#48717,#48718,#48719,#48720,#48721,#48722,#48723,#48724,#48725,#48726,#48727,
#48728,#48729,#48730,#48731,#48732,#48733,#48734,#48735,#48736,#48737,#48738,
#48739,#48740,#48741,#48742,#48743,#48744,#48745,#48746,#48747,#48748,#48749,
#48750,#48751,#48752,#48753,#48754,#48755,#48756,#48757,#48758,#48759,#48760,
#48761,#48762,#48763,#48764,#48765,#48766,#48767,#48768,#48769,#48770,#48771,
#48772,#48773,#48774,#48775,#48776,#48777,#48778,#48779,#48780,#48781,#48782,
#48783,#48784,#48785,#48786,#48787,#48788,#48789,#48790,#48791,#48792,#48793,
#48794,#48795,#48796,#48797,#48798,#48799,#48800,#48801,#48802,#48803,#48804,
#48805,#48806,#48807,#48808,#48809,#48810,#48811,#48812,#48813,#48814,#48815,
#48816,#48817,#48818,#48819,#48820,#48821,#48822,#48823,#48824,#48825,#48826,
#48827,#48828,#48829,#48830,#48831,#48832,#48833,#48834,#48835,#48836,#48837,
#48838,#48839,#48840,#48841,#48842,#48843,#48844,#48845,#48846,#48847,#48848,
#48849,#48850,#48851,#48852,#48853,#48854,#48855,#48856,#48857,#48858,#48859,
#48860,#48861,#48862,#48863,#48864,#48865,#48866,#48867,#48868,#48869,#48870,
#48871,#48872,#48873,#48874,#48875,#48876,#48877,#48878,#48879,#48880,#48881,
#48882,#48883,#48884,#48885,#48886,#48887,#48888,#48889,#48890,#48891,#48892,
#48893,#48894,#48895,#48896,#48897,#48898,#48899,#48900,#48901,#48902,#48903,
#48904,#48905,#48906,#48907,#48908,#48909,#48910,#48911,#48912,#48913,#48914,
#48915,#48916,#48917,#48918,#48919,#48920),(#48921,#48922,#48923,#48924,
#48925,#48926,#48927,#48928,#48929,#48930,#48931,#48932,#48933,#48934,#48935,
#48936,#48937,#48938,#48939,#48940,#48941,#48942,#48943,#48944,#48945,#48946,
#48947,#48948,#48949,#48950,#48951,#48952,#48953,#48954,#48955,#48956,#48957,
#48958,#48959,#48960,#48961,#48962,#48963,#48964,#48965,#48966,#48967,#48968,
#48969,#48970,#48971,#48972,#48973,#48974,#48975,#48976,#48977,#48978,#48979,
#48980,#48981,#48982,#48983,#48984,#48985,#48986,#48987,#48988,#48989,#48990,
#48991,#48992,#48993,#48994,#48995,#48996,#48997,#48998,#48999,#49000,#49001,
#49002,#49003,#49004,#49005,#49006,#49007,#49008,#49009,#49010,#49011,#49012,
#49013,#49014,#49015,#49016,#49017,#49018,#49019,#49020,#49021,#49022,#49023,
#49024,#49025,#49026,#49027,#49028,#49029,#49030,#49031,#49032,#49033,#49034,
#49035,#49036,#49037,#49038,#49039,#49040,#49041,#49042,#49043,#49044,#49045,
#49046,#49047,#49048,#49049,#49050,#49051,#49052,#49053,#49054,#49055,#49056,
#49057,#49058,#49059,#49060,#49061,#49062,#49063,#49064,#49065,#49066,#49067,
#49068,#49069,#49070,#49071,#49072,#49073,#49074,#49075,#49076,#49077,#49078,
#49079,#49080,#49081,#49082,#49083,#49084,#49085,#49086,#49087,#49088,#49089,
#49090,#49091,#49092,#49093,#49094,#49095,#49096,#49097,#49098,#49099,#49100,
#49101,#49102,#49103,#49104,#49105,#49106,#49107,#49108,#49109,#49110,#49111,
#49112,#49113,#49114,#49115,#49116,#49117,#49118,#49119,#49120,#49121,#49122,
#49123,#49124,#49125,#49126,#49127,#49128,#49129,#49130,#49131,#49132,#49133,
#49134,#49135,#49136,#49137,#49138,#49139,#49140,#49141,#49142,#49143,#49144,
#49145,#49146,#49147,#49148,#49149,#49150,#49151,#49152,#49153,#49154,#49155,
#49156,#49157,#49158,#49159,#49160,#49161,#49162,#49163,#49164,#49165,#49166,
#49167,#49168,#49169,#49170,#49171,#49172,#49173,#49174,#49175,#49176,#49177,
#49178,#49179,#49180,#49181,#49182,#49183,#49184,#49185,#49186,#49187,#49188,
#49189,#49190,#49191,#49192,#49193,#49194,#49195,#49196,#49197,#49198,#49199,
#49200,#49201,#49202,#49203,#49204,#49205,#49206,#49207,#49208,#49209,#49210,
#49211,#49212,#49213,#49214,#49215,#49216,#49217,#49218,#49219,#49220,#49221,
#49222,#49223,#49224,#49225,#49226,#49227,#49228,#49229,#49230,#49231,#49232,
#49233,#49234,#49235,#49236,#49237,#49238,#49239,#49240,#49241,#49242,#49243,
#49244,#49245,#49246,#49247,#49248,#49249,#49250,#49251,#49252,#49253,#49254,
#49255,#49256,#49257,#49258,#49259,#49260,#49261,#49262,#49263,#49264,#49265,
#49266,#49267,#49268,#49269,#49270,#49271,#49272,#49273,#49274,#49275,#49276,
#49277,#49278,#49279,#49280,#49281,#49282,#49283,#49284,#49285,#49286,#49287,
#49288,#49289,#49290,#49291,#49292,#49293,#49294,#49295,#49296,#49297,#49298,
#49299,#49300,#49301,#49302,#49303,#49304,#49305,#49306,#49307,#49308,#49309,
#49310,#49311,#49312,#49313,#49314,#49315,#49316,#49317,#49318,#49319,#49320,
#49321,#49322,#49323,#49324,#49325,#49326,#49327,#49328,#49329,#49330,#49331,
#49332,#49333,#49334,#49335,#49336,#49337,#49338,#49339,#49340,#49341,#49342,
#49343,#49344,#49345,#49346,#49347,#49348,#49349,#49350,#49351,#49352,#49353,
#49354,#49355,#49356,#49357,#49358,#49359,#49360,#49361,#49362,#49363,#49364,
#49365,#49366,#49367,#49368,#49369,#49370,#49371,#49372,#49373,#49374,#49375,
#49376,#49377,#49378,#49379,#49380,#49381,#49382,#49383,#49384,#49385,#49386,
#49387,#49388,#49389,#49390,#49391,#49392,#49393,#49394,#49395,#49396,#49397,
#49398,#49399,#49400,#49401,#49402,#49403,#49404,#49405,#49406,#49407,#49408,
#49409,#49410,#49411,#49412,#49413,#49414,#49415,#49416,#49417,#49418,#49419,
#49420,#49421,#49422,#49423,#49424,#49425,#49426,#49427,#49428,#49429,#49430,
#49431,#49432,#49433,#49434,#49435,#49436,#49437,#49438,#49439,#49440,#49441,
#49442,#49443,#49444,#49445,#49446,#49447,#49448,#49449,#49450,#49451)),
 .UNSPECIFIED.,.F.,.F.,.F.,(4,4),(4,1,1,1,1,1,1,1,1,1,1,1,1,1,1,1,1,1,1,
1,1,1,1,1,1,1,1,1,1,1,1,1,1,1,1,1,1,1,1,1,1,1,1,1,1,1,1,1,1,1,1,1,1,1,1,
1,1,1,1,1,1,1,1,1,1,1,1,1,1,1,1,1,1,1,1,1,1,1,1,1,1,1,1,1,1,1,1,1,1,1,1,
1,1,1,1,1,1,1,1,1,1,1,1,1,1,1,1,1,1,1,1,1,1,1,1,1,1,1,1,1,1,1,1,1,1,1,1,
1,1,1,1,1,1,1,1,1,1,1,1,1,1,1,1,1,1,1,1,1,1,1,1,1,1,1,1,1,1,1,1,1,1,1,1,
1,1,1,1,1,1,1,1,1,1,1,1,1,1,1,1,1,1,1,1,1,1,1,1,1,1,1,1,1,1,1,1,1,1,1,1,
1,1,1,1,1,1,1,1,1,1,1,1,1,1,1,1,1,1,1,1,1,1,1,1,1,1,1,1,1,1,1,1,1,1,1,1,
1,1,1,1,1,1,1,1,1,1,1,1,1,1,1,1,1,1,1,1,1,1,1,1,1,1,1,1,1,1,1,1,1,1,1,1,
1,1,1,1,1,1,1,1,1,1,1,1,1,1,1,1,1,1,1,1,1,1,1,1,1,1,1,1,1,1,1,1,1,1,1,1,
1,1,1,1,1,1,1,1,1,1,1,1,1,1,1,1,1,1,1,1,1,1,1,1,1,1,1,1,1,1,1,1,1,1,1,1,
1,1,1,1,1,1,1,1,1,1,1,1,1,1,1,1,1,1,1,1,1,1,1,1,1,1,1,1,1,1,1,1,1,1,1,1,
1,1,1,1,1,1,1,1,1,1,1,1,1,1,1,1,1,1,1,1,1,1,1,1,1,1,1,1,1,1,1,1,1,1,1,1,
1,1,1,1,1,1,1,1,1,1,1,1,1,1,1,1,1,1,1,1,1,1,1,1,1,1,1,1,1,1,1,1,1,1,1,1,
1,1,1,1,1,1,1,1,1,1,1,1,1,1,1,1,1,1,1,1,1,1,1,1,1,1,1,1,1,1,1,1,1,1,1,1,
1,1,1,1,1,1,1,1,1,1,1,1,1,1,1,1,1,1,1,1,1,1,1,1,1,1,1,1,1,1,1,1,1,1,1,1,
1,1,1,1,1,4),(-1.81545167298606E-13,0.23619887080812),(8.98757472625061,
9.48752163453545,9.98746854282029,10.4874154511051,10.98736235939,11.4873092676748,
11.9872561759597,12.4872030842445,12.9871499925294,13.4870969008142,13.987043809099,
14.4869907173839,14.9869376256687,15.4868845339536,15.9868314422384,16.4867783505233,
16.9867252588081,17.4866721670929,17.9866190753778,18.4865659836626,18.9865128919475,
19.4864598002323,19.9864067085172,20.486353616802,20.9863005250869,21.4862474333717,
21.9861943416565,22.4861412499414,22.9860881582262,23.4860350665111,23.9859819747959,
24.4859288830808,24.9858757913656,25.4858226996504,25.9857696079353,26.4857165162201,
26.985663424505,27.4856103327898,27.9855572410747,28.4855041493595,28.9854510576443,
29.4853979659292,29.985344874214,30.4852917824989,30.9852386907837,31.4851855990686,
31.9851325073534,32.4850794156383,32.9850263239231,33.4849732322079,33.9849201404928,
34.4848670487776,34.9848139570625,35.4847608653473,35.9847077736322,36.484654681917,
36.9846015902018,37.4845484984867,37.9844954067715,38.4844423150564,38.9843892233412,
39.4843361316261,39.9842830399109,40.4842299481957,40.9841768564806,41.4841237647654,
41.9840706730503,42.4840175813351,42.98396448962,43.4839113979048,43.9838583061896,
44.4838052144745,44.9837521227593,45.4836990310442,45.983645939329,46.4835928476139,
46.9835397558987,47.4834866641836,47.9834335724684,48.4833804807532,48.9833273890381,
49.4832742973229,49.9832212056078,50.4831681138926,50.9831150221775,51.4830619304623,
51.9830088387471,52.482955747032,52.9829026553168,53.4828495636017,53.9827964718865,
54.4827433801714,54.9826902884562,55.4826371967411,55.9825841050259,56.4825310133107,
56.9824779215956,57.4824248298804,57.9823717381653,58.4823186464501,58.982265554735,
59.4822124630198,59.9821593713046,60.4821062795895,60.9820531878743,61.4820000961592,
61.981947004444,62.4818939127289,62.9818408210137,63.4817877292985,63.9817346375834,
64.4816815458682,64.9816284541531,65.4815753624379,65.9815222707228,66.4814691790076,
66.9814160872924,67.4813629955773,67.9813099038621,68.481256812147,68.9812037204318,
69.4811506287167,69.9810975370015,70.4810444452864,70.9809913535712,71.480938261856,
71.9808851701409,72.4808320784257,72.9807789867106,73.4807258949954,73.9806728032802,
74.4806197115651,74.98056661985,75.4805135281348,75.9804604364196,76.4804073447045,
76.9803542529893,77.4803011612742,77.980248069559,78.4801949778438,78.9801418861287,
79.4800887944135,79.9800357026984,80.4799826109832,80.9799295192681,81.4798764275529,
81.9798233358378,82.4797702441226,82.9797171524074,83.4796640606923,83.9796109689771,
84.479557877262,84.9795047855468,85.4794516938317,85.9793986021165,86.4793455104013,
86.9792924186862,87.479239326971,87.9791862352559,88.4791331435407,88.9790800518255,
89.4790269601104,89.9789738683953,90.4789207766801,90.9788676849649,91.4788145932498,
91.9787615015346,92.4787084098195,92.9786553181043,93.4786022263891,93.978549134674,
94.4784960429588,94.9784429512437,95.4783898595285,95.9783367678134,96.4782836760982,
96.9782305843831,97.4781774926679,97.9781244009527,98.4780713092376,98.9780182175224,
99.4779651258073,99.9779120340921,100.477858942377,100.977805850662,101.477752758947,
101.977699667231,102.477646575516,102.977593483801,103.477540392086,103.977487300371,
104.477434208656,104.977381116941,105.477328025225,105.97727493351,106.477221841795,
106.97716875008,107.477115658365,107.97706256665,108.477009474934,108.976956383219,
109.476903291504,109.976850199789,110.476797108074,110.976744016359,111.476690924644,
111.976637832928,112.476584741213,112.976531649498,113.476478557783,113.976425466068,
114.476372374353,114.976319282637,115.476266190922,115.976213099207,116.476160007492,
116.976106915777,117.476053824062,117.976000732346,118.475947640631,118.975894548916,
119.475841457201,119.975788365486,120.475735273771,120.975682182056,121.47562909034,
121.975575998625,122.47552290691,122.975469815195,123.47541672348,123.975363631765,
124.475310540049,124.975257448334,125.475204356619,125.975151264904,126.475098173189,
126.975045081474,127.474991989759,127.974938898043,128.474885806328,128.974832714613,
129.474779622898,129.974726531183,130.474673439468,130.974620347752,131.474567256037,
131.974514164322,132.474461072607,132.974407980892,133.474354889177,133.974301797461,
134.474248705746,134.974195614031,135.474142522316,135.974089430601,136.474036338886,
136.973983247171,137.473930155455,137.97387706374,138.473823972025,138.97377088031,
139.97366469688,140.973558513449,141.473505421734,141.973452330019,142.473399238304,
142.973346146589,143.473293054873,143.973239963158,144.473186871443,144.973133779728,
145.473080688013,145.973027596298,146.472974504583,146.972921412867,147.472868321152,
147.972815229437,148.472762137722,148.972709046007,149.472655954292,149.972602862576,
150.472549770861,150.972496679146,151.472443587431,151.972390495716,152.472337404001,
152.972284312286,153.47223122057,153.972178128855,154.47212503714,154.972071945425,
155.47201885371,155.971965761995,156.471912670279,156.971859578564,157.471806486849,
157.971753395134,158.471700303419,158.971647211704,159.471594119988,159.971541028273,
160.471487936558,160.971434844843,161.471381753128,161.971328661413,162.471275569698,
162.971222477982,163.471169386267,163.971116294552,164.471063202837,164.971010111122,
165.470957019407,165.970903927691,166.470850835976,166.970797744261,167.470744652546,
167.970691560831,168.470638469116,168.970585377401,169.470532285685,169.97047919397,
170.470426102255,170.97037301054,171.470319918825,171.97026682711,172.470213735394,
172.970160643679,173.470107551964,173.970054460249,174.470001368534,174.969948276819,
175.469895185103,175.969842093388,176.469789001673,176.969735909958,177.469682818243,
177.969629726528,178.469576634813,178.969523543097,179.469470451382,179.969417359667,
180.469364267952,180.969311176237,181.469258084522,181.969204992806,182.469151901091,
182.969098809376,183.469045717661,183.968992625946,184.468939534231,184.968886442515,
185.4688333508,185.968780259085,186.46872716737,186.968674075655,187.46862098394,
187.968567892225,188.468514800509,188.968461708794,189.468408617079,189.968355525364,
190.468302433649,190.968249341934,191.468196250218,191.968143158503,192.468090066788,
192.968036975073,193.467983883358,193.967930791643,194.467877699928,194.967824608212,
195.467771516497,195.967718424782,196.467665333067,196.967612241352,197.467559149637,
197.967506057921,198.467452966206,198.967399874491,199.467346782776,199.967293691061,
200.467240599346,200.967187507631,201.467134415915,201.9670813242,202.467028232485,
202.96697514077,203.466922049055,203.96686895734,204.466815865624,204.966762773909,
205.466709682194,205.966656590479,206.466603498764,206.966550407049,207.466497315333,
207.966444223618,208.466391131903,208.966338040188,209.466284948473,209.966231856758,
210.466178765043,210.966125673327,211.466072581612,211.966019489897,212.465966398182,
212.965913306467,213.465860214752,213.965807123036,214.465754031321,214.965700939606,
215.465647847891,215.965594756176,216.465541664461,216.965488572745,217.46543548103,
217.965382389315,218.4653292976,218.965276205885,219.46522311417,219.965170022455,
220.465116930739,220.965063839024,221.465010747309,221.964957655594,222.464904563879,
222.964851472164,223.464798380448,223.964745288733,224.464692197018,224.964639105303,
225.464586013588,225.964532921873,226.464479830158,226.964426738442,227.464373646727,
227.964320555012,228.464267463297,228.964214371582,229.464161279867,229.964108188151,
230.464055096436,230.964002004721,231.463948913006,231.963895821291,232.463842729576,
232.96378963786,233.463736546145,233.96368345443,234.463630362715,234.963577271,
235.463524179285,235.96347108757,236.463417995854,236.963364904139,237.463311812424,
237.963258720709,238.463205628994,238.963152537279,239.463099445563,239.963046353848,
240.462993262133,240.962940170418,241.462887078703,241.962833986988,242.462780895273,
242.962727803557,243.462674711842,243.962621620127,244.462568528412,244.962515436697,
245.462462344982,245.962409253266,246.462356161551,246.962303069836,247.462249978121,
247.962196886406,248.462143794691,248.962090702975,249.46203761126,249.961984519545,
250.46193142783,250.961878336115,251.4618252444,251.961772152685,252.461719060969,
252.961665969254,253.461612877539,253.961559785824,254.461506694109,254.961453602394,
255.461400510678,255.961347418963,256.461294327248,256.961241235533,257.461188143818,
257.961135052103,258.461081960387,258.961028868672,259.460975776957,259.960922685242,
260.460869593527,260.960816501812,261.460763410097,261.960710318381,262.460657226666,
262.960604134951,263.460551043236,263.960497951521,264.460444859806,264.96039176809,
265.460338676375,265.96028558466,266.460232492945,266.96017940123,267.460126309515,
267.9600732178,268.460020126084,268.959967034369,269.459913942654,269.959860850939,
270.459807759224,270.959754667509,271.459701575793,271.959648484078,272.459595392363,
272.959542300648,273.459489208933,273.959436117218),.UNSPECIFIED.);
#239=B_SPLINE_CURVE_WITH_KNOTS('',3,(#40100,#40101,#40102,#40103,#40104,
#40105,#40106,#40107,#40108,#40109,#40110,#40111,#40112,#40113,#40114,#40115,
#40116,#40117,#40118,#40119,#40120,#40121),.UNSPECIFIED.,.F.,.F.,(4,3,3,
3,3,3,3,4),(-3.6646581839854,-3.4918212590925,-2.99298965065071,-2.49415804220892,
-1.99532643376714,-1.49649482532536,-0.99766321688357,-0.960268764914586),
 .UNSPECIFIED.);
#240=B_SPLINE_CURVE_WITH_KNOTS('',3,(#40124,#40125,#40126,#40127),
 .UNSPECIFIED.,.F.,.F.,(4,4),(0.,0.437203234519499),.UNSPECIFIED.);
#241=B_SPLINE_CURVE_WITH_KNOTS('',3,(#40132,#40133,#40134,#40135,#40136,
#40137,#40138,#40139,#40140,#40141,#40142,#40143,#40144,#40145,#40146,#40147,
#40148,#40149,#40150,#40151,#40152,#40153,#40154,#40155,#40156,#40157,#40158,
#40159,#40160,#40161,#40162,#40163,#40164,#40165,#40166,#40167,#40168),
 .UNSPECIFIED.,.F.,.F.,(4,3,3,3,3,3,3,3,3,3,3,3,4),(-9.94784349116496,-9.47780056039391,
-8.97896895195213,-8.48013734351034,-7.98130573506856,-7.48247412662677,
-6.98364251818499,-6.48481090974321,-5.98597930130142,-5.48714769285963,
-4.98831608441785,-3.99065286753428,-3.6646581839854),.UNSPECIFIED.);
#242=B_SPLINE_CURVE_WITH_KNOTS('',3,(#40169,#40170,#40171,#40172,#40173,
#40174,#40175,#40176,#40177,#40178,#40179,#40180,#40181,#40182,#40183,#40184,
#40185,#40186,#40187,#40188,#40189,#40190,#40191,#40192,#40193,#40194,#40195,
#40196,#40197,#40198,#40199,#40200,#40201,#40202,#40203,#40204,#40205,#40206,
#40207,#40208,#40209,#40210,#40211),.UNSPECIFIED.,.F.,.F.,(4,3,3,3,3,3,
3,3,3,3,3,3,3,3,4),(0.437203234519499,0.499946908284749,0.999893816569588,
1.49984072485443,1.99978763313927,2.49973454142411,2.99968144970895,3.49962835799379,
3.99957526627863,4.49952217456346,4.99946908284831,5.49941599113315,5.99936289941799,
6.49930980770282,6.72038854169909),.UNSPECIFIED.);
#243=B_SPLINE_CURVE_WITH_KNOTS('',3,(#40216,#40217,#40218,#40219,#40220,
#40221,#40222,#40223,#40224,#40225,#40226,#40227,#40228,#40229,#40230,#40231,
#40232,#40233,#40234,#40235,#40236,#40237,#40238,#40239,#40240,#40241,#40242,
#40243,#40244,#40245,#40246,#40247,#40248,#40249,#40250,#40251,#40252,#40253,
#40254,#40255),.UNSPECIFIED.,.F.,.F.,(4,3,3,3,3,3,3,3,3,3,3,3,3,4),(-16.2310287983446,
-15.9626114701371,-15.4637798616953,-14.9649482532535,-14.4661166448118,
-13.96728503637,-13.4684534279282,-12.9696218194864,-12.4707902110446,-11.9719586026028,
-10.9742953857193,-10.4754637772775,-9.9766321688357,-9.94784349116496),
 .UNSPECIFIED.);
#244=B_SPLINE_CURVE_WITH_KNOTS('',3,(#40256,#40257,#40258,#40259,#40260,
#40261,#40262,#40263,#40264,#40265,#40266,#40267,#40268,#40269,#40270,#40271,
#40272,#40273,#40274,#40275,#40276,#40277,#40278,#40279,#40280,#40281,#40282,
#40283,#40284,#40285,#40286,#40287,#40288,#40289,#40290,#40291,#40292,#40293,
#40294,#40295,#40296,#40297,#40298),.UNSPECIFIED.,.F.,.F.,(4,3,3,3,3,3,
3,3,3,3,3,3,3,3,4),(6.72038854169909,6.99925671598767,7.49920362427252,
7.99915053255736,8.49909744084221,8.99904434912705,9.4989912574119,9.99893816569675,
10.4988850739816,10.9988319822664,11.4987788905513,11.9987257988361,12.498672707121,
12.9986196154058,13.0035738488787),.UNSPECIFIED.);
#245=B_SPLINE_CURVE_WITH_KNOTS('',3,(#40303,#40304,#40305,#40306,#40307,
#40308,#40309,#40310,#40311,#40312,#40313,#40314,#40315,#40316,#40317,#40318,
#40319,#40320,#40321,#40322,#40323,#40324,#40325,#40326,#40327,#40328,#40329,
#40330,#40331,#40332,#40333,#40334,#40335,#40336,#40337,#40338,#40339,#40340,
#40341,#40342),.UNSPECIFIED.,.F.,.F.,(4,3,3,3,3,3,3,3,3,3,3,3,3,4),(-22.5142141055241,
-22.4474223798803,-21.9485907714385,-21.4497591629967,-20.950927554555,
-20.4520959461132,-19.9532643376714,-19.4544327292296,-18.9556011207878,
-17.9579379039043,-17.4591062954625,-16.9602746870207,-16.4614430785789,
-16.2310287983446),.UNSPECIFIED.);
#246=B_SPLINE_CURVE_WITH_KNOTS('',3,(#40343,#40344,#40345,#40346,#40347,
#40348,#40349,#40350,#40351,#40352,#40353,#40354,#40355,#40356,#40357,#40358,
#40359,#40360,#40361,#40362,#40363,#40364,#40365,#40366,#40367,#40368,#40369,
#40370,#40371,#40372,#40373,#40374,#40375,#40376,#40377,#40378,#40379,#40380,
#40381,#40382),.UNSPECIFIED.,.F.,.F.,(4,3,3,3,3,3,3,3,3,3,3,3,3,4),(13.0035738488787,
13.4985665236907,13.9985134319755,14.4984603402604,14.9984072485452,15.49835415683,
15.9983010651149,16.4982479733997,16.9981948816846,17.4981417899694,17.9980886982543,
18.4980356065391,18.9979825148239,19.2867591560582),.UNSPECIFIED.);
#247=B_SPLINE_CURVE_WITH_KNOTS('',3,(#40387,#40388,#40389,#40390,#40391,
#40392,#40393,#40394,#40395,#40396,#40397,#40398,#40399,#40400,#40401,#40402,
#40403,#40404,#40405,#40406,#40407,#40408,#40409,#40410,#40411),
 .UNSPECIFIED.,.F.,.F.,(4,3,3,3,3,3,3,3,4),(-28.7973994127037,-28.008505735355,
-27.2196120580062,-26.4307183806574,-25.6418247033086,-24.8529310259599,
-24.0640373486111,-23.2751436712623,-22.5142141055241),.UNSPECIFIED.);
#248=B_SPLINE_CURVE_WITH_KNOTS('',3,(#40412,#40413,#40414,#40415,#40416,
#40417,#40418,#40419,#40420,#40421,#40422,#40423,#40424,#40425,#40426,#40427,
#40428,#40429,#40430,#40431,#40432,#40433,#40434,#40435,#40436,#40437,#40438,
#40439,#40440,#40441,#40442,#40443,#40444,#40445,#40446,#40447,#40448,#40449,
#40450,#40451,#40452,#40453,#40454),.UNSPECIFIED.,.F.,.F.,(4,3,3,3,3,3,
3,3,3,3,3,3,3,3,4),(19.2867591560582,19.4979294231088,19.9978763313936,
20.4978232396785,20.9977701479633,21.4977170562482,21.997663964533,22.4976108728179,
22.9975577811027,23.4975046893875,23.9974515976724,24.4973985059572,24.9973454142421,
25.4972923225269,25.5699444632378),.UNSPECIFIED.);
#249=B_SPLINE_CURVE_WITH_KNOTS('',3,(#40459,#40460,#40461,#40462,#40463,
#40464,#40465,#40466,#40467,#40468,#40469,#40470,#40471,#40472,#40473,#40474,
#40475,#40476,#40477,#40478,#40479,#40480,#40481,#40482,#40483),
 .UNSPECIFIED.,.F.,.F.,(4,3,3,3,3,3,3,3,4),(-35.0805847198833,-34.2916910425345,
-33.5027973651858,-32.713903687837,-31.9250100104882,-31.1361163331394,
-30.3472226557907,-29.5583289784419,-28.7973994127037),.UNSPECIFIED.);
#250=B_SPLINE_CURVE_WITH_KNOTS('',3,(#40484,#40485,#40486,#40487,#40488,
#40489,#40490,#40491,#40492,#40493,#40494,#40495,#40496,#40497,#40498,#40499,
#40500,#40501,#40502,#40503,#40504,#40505,#40506,#40507,#40508,#40509,#40510,
#40511,#40512,#40513,#40514,#40515,#40516,#40517,#40518,#40519,#40520,#40521,
#40522,#40523),.UNSPECIFIED.,.F.,.F.,(4,3,3,3,3,3,3,3,3,3,3,3,3,4),(25.5699444632378,
25.9972392308118,26.4971861390966,26.9971330473814,27.4970799556663,27.9970268639511,
28.496973772236,28.9969206805208,29.4968675888057,29.9968144970905,30.4967614053753,
30.9967083136602,31.496655221945,31.8531297704174),.UNSPECIFIED.);
#251=B_SPLINE_CURVE_WITH_KNOTS('',3,(#40528,#40529,#40530,#40531,#40532,
#40533,#40534,#40535,#40536,#40537,#40538,#40539,#40540,#40541,#40542,#40543,
#40544,#40545,#40546,#40547,#40548,#40549,#40550,#40551,#40552,#40553,#40554,
#40555,#40556,#40557,#40558,#40559,#40560,#40561,#40562,#40563,#40564),
 .UNSPECIFIED.,.F.,.F.,(4,3,3,3,3,3,3,3,3,3,3,3,4),(-41.3637700270629,-40.9041918922264,
-40.4053602837846,-39.9065286753428,-38.9088654584592,-38.4100338500174,
-37.9112022415756,-37.4123706331339,-36.9135390246921,-36.4147074162503,
-35.9158758078085,-35.4170441993667,-35.0805847198833),.UNSPECIFIED.);
#252=B_SPLINE_CURVE_WITH_KNOTS('',3,(#40565,#40566,#40567,#40568,#40569,
#40570,#40571,#40572,#40573,#40574,#40575,#40576,#40577,#40578,#40579,#40580,
#40581,#40582,#40583,#40584,#40585,#40586,#40587,#40588,#40589,#40590,#40591,
#40592,#40593,#40594,#40595,#40596,#40597,#40598,#40599,#40600,#40601,#40602,
#40603,#40604,#40605,#40606,#40607),.UNSPECIFIED.,.F.,.F.,(4,3,3,3,3,3,
3,3,3,3,3,3,3,3,4),(31.8531297704174,31.9966021302299,32.4965490385147,
32.9964959467996,33.4964428550844,33.9963897633693,34.4963366716541,34.9962835799389,
35.4962304882238,35.9961773965086,36.4961243047935,36.9960712130783,37.4960181213632,
37.995965029648,38.136315077597),.UNSPECIFIED.);
#253=B_SPLINE_CURVE_WITH_KNOTS('',3,(#40612,#40613,#40614,#40615,#40616,
#40617,#40618,#40619,#40620,#40621,#40622,#40623,#40624,#40625,#40626,#40627,
#40628,#40629,#40630,#40631,#40632,#40633,#40634,#40635,#40636,#40637,#40638,
#40639,#40640,#40641,#40642,#40643,#40644,#40645,#40646,#40647,#40648,#40649,
#40650,#40651),.UNSPECIFIED.,.F.,.F.,(4,3,3,3,3,3,3,3,3,3,3,3,3,4),(-47.6469553342425,
-47.3890028019696,-46.8901711935278,-45.8925079766442,-45.3936763682024,
-44.8948447597606,-44.3960131513188,-43.8971815428771,-43.3983499344353,
-42.8995183259935,-42.4006867175517,-41.9018551091099,-41.4030235006681,
-41.3637700270629),.UNSPECIFIED.);
#254=B_SPLINE_CURVE_WITH_KNOTS('',3,(#40652,#40653,#40654,#40655,#40656,
#40657,#40658,#40659,#40660,#40661,#40662,#40663,#40664,#40665,#40666,#40667,
#40668,#40669,#40670,#40671,#40672,#40673,#40674,#40675,#40676,#40677,#40678,
#40679,#40680,#40681,#40682,#40683,#40684,#40685,#40686,#40687,#40688,#40689,
#40690,#40691),.UNSPECIFIED.,.F.,.F.,(4,3,3,3,3,3,3,3,3,3,3,3,3,4),(38.136315077597,
38.4959119379328,38.9958588462177,39.4958057545025,39.9957526627874,40.4956995710722,
40.9956464793571,41.4955933876419,41.9955402959268,42.4954872042116,42.9954341124965,
43.4953810207813,43.9953279290661,44.4195003847766),.UNSPECIFIED.);
#255=B_SPLINE_CURVE_WITH_KNOTS('',3,(#40696,#40697,#40698,#40699,#40700,
#40701,#40702,#40703,#40704,#40705,#40706,#40707,#40708,#40709,#40710,#40711,
#40712,#40713,#40714,#40715,#40716,#40717,#40718,#40719,#40720,#40721,#40722,
#40723,#40724,#40725,#40726,#40727,#40728,#40729,#40730,#40731,#40732,#40733,
#40734,#40735),.UNSPECIFIED.,.F.,.F.,(4,3,3,3,3,3,3,3,3,3,3,3,3,4),(-53.9301406414221,
-53.8738137117128,-52.8761504948292,-52.3773188863874,-51.8784872779456,
-51.3796556695038,-50.8808240610621,-50.3819924526203,-49.8831608441785,
-49.3843292357367,-48.8854976272949,-48.3866660188531,-47.8878344104113,
-47.6469553342425),.UNSPECIFIED.);
#256=B_SPLINE_CURVE_WITH_KNOTS('',3,(#40736,#40737,#40738,#40739,#40740,
#40741,#40742,#40743,#40744,#40745,#40746,#40747,#40748,#40749,#40750,#40751,
#40752,#40753,#40754,#40755,#40756,#40757,#40758,#40759,#40760,#40761,#40762,
#40763,#40764,#40765,#40766,#40767,#40768,#40769,#40770,#40771,#40772,#40773,
#40774,#40775,#40776,#40777,#40778),.UNSPECIFIED.,.F.,.F.,(4,3,3,3,3,3,
3,3,3,3,3,3,3,3,4),(44.4195003847766,44.495274837351,44.9952217456358,45.4951686539207,
45.9951155622055,46.4950624704904,46.9950093787752,47.49495628706,47.9949031953449,
48.4948501036297,48.9947970119145,49.4947439201994,49.9946908284842,50.4946377367691,
50.7026856919562),.UNSPECIFIED.);
#257=B_SPLINE_CURVE_WITH_KNOTS('',3,(#40783,#40784,#40785,#40786,#40787,
#40788,#40789,#40790,#40791,#40792,#40793,#40794,#40795,#40796,#40797,#40798,
#40799,#40800,#40801,#40802,#40803,#40804,#40805,#40806,#40807,#40808,#40809,
#40810,#40811,#40812,#40813,#40814,#40815,#40816,#40817,#40818,#40819,#40820,
#40821,#40822),.UNSPECIFIED.,.F.,.F.,(4,3,3,3,3,3,3,3,3,3,3,3,3,4),(-60.2133259486017,
-59.8597930130142,-59.3609614045724,-58.8621297961306,-58.3632981876888,
-57.864466579247,-57.3656349708053,-56.8668033623635,-56.3679717539217,
-55.8691401454799,-55.3703085370381,-54.8714769285963,-54.3726453201545,
-53.9301406414221),.UNSPECIFIED.);
#258=B_SPLINE_CURVE_WITH_KNOTS('',3,(#40823,#40824,#40825,#40826,#40827,
#40828,#40829,#40830,#40831,#40832,#40833,#40834,#40835,#40836,#40837,#40838,
#40839,#40840,#40841,#40842,#40843,#40844,#40845,#40846,#40847,#40848,#40849,
#40850,#40851,#40852,#40853,#40854,#40855,#40856,#40857,#40858,#40859,#40860,
#40861,#40862),.UNSPECIFIED.,.F.,.F.,(4,3,3,3,3,3,3,3,3,3,3,3,3,4),(50.7026856919562,
50.9945846450539,51.4945315533388,51.9944784616236,52.4944253699085,52.9943722781933,
53.4943191864781,53.994266094763,54.4942130030478,54.9941599113327,55.4941068196175,
55.9940537279024,56.4940006361872,56.9858709991358),.UNSPECIFIED.);
#259=B_SPLINE_CURVE_WITH_KNOTS('',3,(#40867,#40868,#40869,#40870,#40871,
#40872,#40873,#40874,#40875,#40876,#40877,#40878,#40879,#40880,#40881,#40882,
#40883,#40884,#40885,#40886,#40887,#40888,#40889,#40890,#40891,#40892,#40893,
#40894,#40895,#40896,#40897,#40898,#40899,#40900,#40901,#40902,#40903,#40904,
#40905,#40906),.UNSPECIFIED.,.F.,.F.,(4,3,3,3,3,3,3,3,3,3,3,3,3,4),(-66.4965112557813,
-66.3446039227574,-65.8457723143156,-65.3469407058738,-64.848109097432,
-64.3492774889902,-63.8504458805484,-63.3516142721067,-62.8527826636649,
-62.3539510552231,-61.8551194467813,-61.3562878383395,-60.8574562298977,
-60.2133259486017),.UNSPECIFIED.);
#260=B_SPLINE_CURVE_WITH_KNOTS('',3,(#40907,#40908,#40909,#40910,#40911,
#40912,#40913,#40914,#40915,#40916,#40917,#40918,#40919,#40920,#40921,#40922,
#40923,#40924,#40925,#40926,#40927,#40928,#40929,#40930,#40931,#40932,#40933,
#40934,#40935,#40936,#40937,#40938,#40939,#40940,#40941,#40942,#40943,#40944,
#40945,#40946,#40947,#40948,#40949),.UNSPECIFIED.,.F.,.F.,(4,3,3,3,3,3,
3,3,3,3,3,3,3,3,4),(56.9858709991358,56.9939475444721,57.4938944527569,
57.9938413610417,58.4937882693266,58.9937351776114,59.4936820858963,59.9936289941811,
60.493575902466,60.9935228107508,61.4934697190356,61.9934166273205,62.4933635356053,
62.9933104438902,63.2690563063154),.UNSPECIFIED.);
#261=B_SPLINE_CURVE_WITH_KNOTS('',3,(#40954,#40955,#40956,#40957,#40958,
#40959,#40960,#40961,#40962,#40963,#40964,#40965,#40966,#40967,#40968,#40969,
#40970,#40971,#40972,#40973,#40974,#40975,#40976,#40977,#40978,#40979,#40980,
#40981,#40982,#40983,#40984,#40985,#40986,#40987,#40988,#40989,#40990),
 .UNSPECIFIED.,.F.,.F.,(4,3,3,3,3,3,3,3,3,3,3,3,4),(-72.7796965629609,-72.3305832240588,
-71.831751615617,-71.3329200071752,-70.8340883987335,-70.3352567902917,
-69.8364251818499,-69.3375935734081,-68.8387619649663,-68.3399303565245,
-67.8410987480827,-66.8434355311992,-66.4965112557813),.UNSPECIFIED.);
#262=B_SPLINE_CURVE_WITH_KNOTS('',3,(#40991,#40992,#40993,#40994,#40995,
#40996,#40997,#40998,#40999,#41000,#41001,#41002,#41003,#41004,#41005,#41006,
#41007,#41008,#41009,#41010,#41011,#41012,#41013,#41014,#41015,#41016,#41017,
#41018,#41019,#41020,#41021,#41022,#41023,#41024,#41025,#41026,#41027,#41028,
#41029,#41030,#41031,#41032,#41033),.UNSPECIFIED.,.F.,.F.,(4,3,3,3,3,3,
3,3,3,3,3,3,3,3,4),(63.2690563063154,63.493257352175,63.9932042604598,64.4931511687447,
64.9930980770295,65.4930449853144,65.9929918935992,66.4929388018841,66.9928857101689,
67.4928326184538,67.9927795267386,68.4927264350235,68.9926733433083,69.4926202515931,
69.552241613495),.UNSPECIFIED.);
#263=B_SPLINE_CURVE_WITH_KNOTS('',3,(#41038,#41039,#41040,#41041,#41042,
#41043,#41044,#41045,#41046,#41047,#41048,#41049,#41050,#41051,#41052,#41053,
#41054,#41055,#41056,#41057,#41058,#41059,#41060,#41061,#41062,#41063,#41064,
#41065,#41066,#41067,#41068,#41069,#41070,#41071,#41072,#41073,#41074,#41075,
#41076,#41077),.UNSPECIFIED.,.F.,.F.,(4,3,3,3,3,3,3,3,3,3,3,3,3,4),(-79.0628818701405,
-78.815394133802,-78.3165625253602,-77.8177309169184,-77.3188993084766,
-76.8200677000349,-76.3212360915931,-75.8224044831513,-75.3235728747095,
-74.8247412662677,-73.8270780493842,-73.3282464409424,-72.8294148325006,
-72.7796965629609),.UNSPECIFIED.);
#264=B_SPLINE_CURVE_WITH_KNOTS('',3,(#41078,#41079,#41080,#41081,#41082,
#41083,#41084,#41085,#41086,#41087,#41088,#41089,#41090,#41091,#41092,#41093,
#41094,#41095,#41096,#41097,#41098,#41099,#41100,#41101,#41102,#41103,#41104,
#41105,#41106,#41107,#41108,#41109,#41110,#41111,#41112,#41113,#41114,#41115,
#41116,#41117),.UNSPECIFIED.,.F.,.F.,(4,3,3,3,3,3,3,3,3,3,3,3,3,4),(69.552241613495,
69.992567159878,70.4925140681628,70.9924609764477,71.4924078847325,71.9923547930174,
72.4923017013022,72.9922486095871,73.4921955178719,73.9921424261567,74.4920893344416,
74.9920362427264,75.4919831510113,75.8354269206746),.UNSPECIFIED.);
#265=B_SPLINE_CURVE_WITH_KNOTS('',3,(#41122,#41123,#41124,#41125,#41126,
#41127,#41128,#41129,#41130,#41131,#41132,#41133,#41134,#41135,#41136,#41137,
#41138,#41139,#41140,#41141,#41142,#41143,#41144,#41145,#41146,#41147,#41148,
#41149,#41150,#41151,#41152,#41153,#41154,#41155,#41156,#41157,#41158,#41159,
#41160,#41161),.UNSPECIFIED.,.F.,.F.,(4,3,3,3,3,3,3,3,3,3,3,3,3,4),(-85.3460671773201,
-85.3002050435452,-84.8013734351034,-84.3025418266616,-83.8037102182198,
-83.3048786097781,-82.8060470013363,-82.3072153928945,-81.8083837844527,
-80.8107205675691,-80.3118889591274,-79.8130573506856,-79.3142257422438,
-79.0628818701405),.UNSPECIFIED.);
#266=B_SPLINE_CURVE_WITH_KNOTS('',3,(#41162,#41163,#41164,#41165,#41166,
#41167,#41168,#41169,#41170,#41171,#41172,#41173,#41174,#41175,#41176,#41177,
#41178,#41179,#41180,#41181,#41182,#41183,#41184,#41185,#41186,#41187,#41188,
#41189,#41190,#41191,#41192,#41193,#41194,#41195,#41196,#41197,#41198,#41199,
#41200,#41201,#41202,#41203,#41204),.UNSPECIFIED.,.F.,.F.,(4,3,3,3,3,3,
3,3,3,3,3,3,3,3,4),(75.8354269206746,75.9919300592961,76.491876967581,76.9918238758658,
77.4917707841506,77.9917176924355,78.4916646007203,78.9916115090052,79.49155841729,
79.9915053255748,80.4914522338597,80.9913991421445,81.4913460504294,81.9912929587142,
82.1186122278542),.UNSPECIFIED.);
#267=B_SPLINE_CURVE_WITH_KNOTS('',3,(#41209,#41210,#41211,#41212,#41213,
#41214,#41215,#41216,#41217,#41218,#41219,#41220,#41221,#41222,#41223,#41224,
#41225,#41226,#41227,#41228,#41229,#41230,#41231,#41232,#41233),
 .UNSPECIFIED.,.F.,.F.,(4,3,3,3,3,3,3,3,4),(-91.6292524844997,-90.8403588071509,
-90.0514651298022,-89.2625714524534,-88.4736777751046,-87.6847840977559,
-86.8958904204071,-86.1069967430584,-85.3460671773201),.UNSPECIFIED.);
#268=B_SPLINE_CURVE_WITH_KNOTS('',3,(#41234,#41235,#41236,#41237,#41238,
#41239,#41240,#41241,#41242,#41243,#41244,#41245,#41246,#41247,#41248,#41249,
#41250,#41251,#41252,#41253,#41254,#41255,#41256,#41257,#41258,#41259,#41260,
#41261,#41262,#41263,#41264,#41265,#41266,#41267,#41268,#41269,#41270,#41271,
#41272,#41273),.UNSPECIFIED.,.F.,.F.,(4,3,3,3,3,3,3,3,3,3,3,3,3,4),(82.1186122278542,
82.4912398669991,82.9911867752839,83.4911336835687,83.9910805918536,84.4910275001384,
84.9909744084233,85.4909213167081,85.990868224993,86.4908151332778,86.9907620415627,
87.4907089498475,87.9906558581323,88.4017975350338),.UNSPECIFIED.);
#269=B_SPLINE_CURVE_WITH_KNOTS('',3,(#41278,#41279,#41280,#41281,#41282,
#41283,#41284,#41285,#41286,#41287,#41288,#41289,#41290,#41291,#41292,#41293,
#41294,#41295,#41296,#41297,#41298,#41299,#41300,#41301,#41302),
 .UNSPECIFIED.,.F.,.F.,(4,3,3,3,3,3,3,3,4),(-97.9124377916793,-97.1235441143305,
-96.3346504369817,-95.545756759633,-94.7568630822842,-93.9679694049355,
-93.1790757275867,-92.390182050238,-91.6292524844997),.UNSPECIFIED.);
#270=B_SPLINE_CURVE_WITH_KNOTS('',3,(#41303,#41304,#41305,#41306,#41307,
#41308,#41309,#41310,#41311,#41312,#41313,#41314,#41315,#41316,#41317,#41318,
#41319,#41320,#41321,#41322,#41323,#41324,#41325,#41326,#41327,#41328,#41329,
#41330,#41331,#41332,#41333,#41334,#41335,#41336,#41337,#41338,#41339,#41340,
#41341,#41342,#41343,#41344,#41345),.UNSPECIFIED.,.F.,.F.,(4,3,3,3,3,3,
3,3,3,3,3,3,3,3,4),(88.4017975350338,88.4906027664172,88.990549674702,89.4904965829869,
89.9904434912717,90.4903903995565,90.9903373078414,91.4902842161263,91.9902311244111,
92.4901780326959,92.9901249409808,93.4900718492656,93.9900187575504,94.4899656658353,
94.6849828422133),.UNSPECIFIED.);
#271=B_SPLINE_CURVE_WITH_KNOTS('',3,(#41350,#41351,#41352,#41353,#41354,
#41355,#41356,#41357,#41358,#41359,#41360,#41361,#41362,#41363,#41364,#41365,
#41366,#41367,#41368,#41369,#41370,#41371,#41372,#41373,#41374,#41375,#41376,
#41377,#41378,#41379,#41380,#41381,#41382,#41383,#41384,#41385,#41386),
 .UNSPECIFIED.,.F.,.F.,(4,3,3,3,3,3,3,3,3,3,3,3,4),(-104.195623098859,-103.756974555891,
-103.258142947449,-102.759311339008,-101.761648122124,-101.262816513682,
-100.763984905241,-100.265153296799,-99.766321688357,-99.2674900799152,
-98.7686584714734,-98.2698268630316,-97.9124377916793),.UNSPECIFIED.);
#272=B_SPLINE_CURVE_WITH_KNOTS('',3,(#41387,#41388,#41389,#41390,#41391,
#41392,#41393,#41394,#41395,#41396,#41397,#41398,#41399,#41400,#41401,#41402,
#41403,#41404,#41405,#41406,#41407,#41408,#41409,#41410,#41411,#41412,#41413,
#41414,#41415,#41416,#41417,#41418,#41419,#41420,#41421,#41422,#41423,#41424,
#41425,#41426),.UNSPECIFIED.,.F.,.F.,(4,3,3,3,3,3,3,3,3,3,3,3,3,4),(94.6849828422133,
94.9899125741201,95.489859482405,95.9898063906898,96.4897532989747,96.9897002072595,
97.4896471155444,97.9895940238292,98.4895409321141,98.9894878403989,99.4894347486837,
99.9893816569686,100.489328565253,100.968168149393),.UNSPECIFIED.);
#273=B_SPLINE_CURVE_WITH_KNOTS('',3,(#41431,#41432,#41433,#41434,#41435,
#41436,#41437,#41438,#41439,#41440,#41441,#41442,#41443,#41444,#41445,#41446,
#41447,#41448,#41449,#41450,#41451,#41452,#41453,#41454,#41455,#41456,#41457,
#41458,#41459,#41460,#41461,#41462,#41463,#41464,#41465,#41466,#41467,#41468,
#41469,#41470),.UNSPECIFIED.,.F.,.F.,(4,3,3,3,3,3,3,3,3,3,3,3,3,4),(-110.478808406038,
-110.241785465634,-109.742953857193,-108.745290640309,-108.246459031867,
-107.747627423426,-107.248795814984,-106.749964206542,-106.2511325981,-105.752300989658,
-105.253469381217,-104.754637772775,-104.255806164333,-104.195623098859),
 .UNSPECIFIED.);
#274=B_SPLINE_CURVE_WITH_KNOTS('',3,(#41471,#41472,#41473,#41474,#41475,
#41476,#41477,#41478,#41479,#41480,#41481,#41482,#41483,#41484,#41485,#41486,
#41487,#41488,#41489,#41490,#41491,#41492,#41493,#41494,#41495,#41496,#41497,
#41498,#41499,#41500,#41501,#41502,#41503,#41504,#41505,#41506,#41507,#41508,
#41509,#41510,#41511,#41512,#41513),.UNSPECIFIED.,.F.,.F.,(4,3,3,3,3,3,
3,3,3,3,3,3,3,3,4),(100.968168149393,100.989275473538,101.489222381823,
101.989169290108,102.489116198393,102.989063106678,103.489010014963,103.988956923247,
104.488903831532,104.988850739817,105.488797648102,105.988744556387,106.488691464672,
106.988638372956,107.251353456573),.UNSPECIFIED.);
#275=B_SPLINE_CURVE_WITH_KNOTS('',3,(#41518,#41519,#41520,#41521,#41522,
#41523,#41524,#41525,#41526,#41527,#41528,#41529,#41530,#41531,#41532,#41533,
#41534,#41535,#41536,#41537,#41538,#41539,#41540,#41541,#41542,#41543,#41544,
#41545,#41546,#41547,#41548,#41549,#41550,#41551,#41552,#41553,#41554,#41555,
#41556,#41557),.UNSPECIFIED.,.F.,.F.,(4,3,3,3,3,3,3,3,3,3,3,3,3,4),(-116.761993713218,
-116.726596375378,-115.728933158494,-115.230101550052,-114.731269941611,
-114.232438333169,-113.733606724727,-113.234775116285,-112.735943507843,
-112.237111899402,-111.73828029096,-111.239448682518,-110.740617074076,
-110.478808406038),.UNSPECIFIED.);
#276=B_SPLINE_CURVE_WITH_KNOTS('',3,(#41558,#41559,#41560,#41561,#41562,
#41563,#41564,#41565,#41566,#41567,#41568,#41569,#41570,#41571,#41572,#41573,
#41574,#41575,#41576,#41577,#41578,#41579,#41580,#41581,#41582,#41583,#41584,
#41585,#41586,#41587,#41588,#41589,#41590,#41591,#41592,#41593,#41594,#41595,
#41596,#41597,#41598,#41599,#41600),.UNSPECIFIED.,.F.,.F.,(4,3,3,3,3,3,
3,3,3,3,3,3,3,3,4),(107.251353456573,107.488585281241,107.988532189526,
108.488479097811,108.988426006096,109.488372914381,109.988319822665,110.48826673095,
110.988213639235,111.48816054752,111.988107455805,112.48805436409,112.988001272375,
113.487948180659,113.534538763752),.UNSPECIFIED.);
#277=B_SPLINE_CURVE_WITH_KNOTS('',3,(#41605,#41606,#41607,#41608,#41609,
#41610,#41611,#41612,#41613,#41614,#41615,#41616,#41617,#41618,#41619,#41620,
#41621,#41622,#41623,#41624,#41625,#41626,#41627,#41628,#41629,#41630,#41631,
#41632,#41633,#41634,#41635,#41636,#41637,#41638,#41639,#41640,#41641,#41642,
#41643,#41644),.UNSPECIFIED.,.F.,.F.,(4,3,3,3,3,3,3,3,3,3,3,3,3,4),(-123.045179020398,
-122.712575676679,-122.213744068237,-121.714912459795,-121.216080851354,
-120.717249242912,-120.21841763447,-119.719586026028,-119.220754417587,
-118.721922809145,-118.223091200703,-117.724259592261,-117.225427983819,
-116.761993713218),.UNSPECIFIED.);
#278=B_SPLINE_CURVE_WITH_KNOTS('',3,(#41645,#41646,#41647,#41648,#41649,
#41650,#41651,#41652,#41653,#41654,#41655,#41656,#41657,#41658,#41659,#41660,
#41661,#41662,#41663,#41664,#41665,#41666,#41667,#41668,#41669,#41670,#41671,
#41672,#41673,#41674,#41675,#41676,#41677,#41678,#41679,#41680,#41681,#41682,
#41683,#41684),.UNSPECIFIED.,.F.,.F.,(4,3,3,3,3,3,3,3,3,3,3,3,3,4),(113.534538763752,
113.987895088944,114.487841997229,114.987788905514,115.487735813799,115.987682722084,
116.487629630368,116.987576538653,117.487523446938,117.987470355223,118.487417263508,
118.987364171793,119.487311080077,119.817724070932),.UNSPECIFIED.);
#279=B_SPLINE_CURVE_WITH_KNOTS('',3,(#41689,#41690,#41691,#41692,#41693,
#41694,#41695,#41696,#41697,#41698,#41699,#41700,#41701,#41702,#41703,#41704,
#41705,#41706,#41707,#41708,#41709,#41710,#41711,#41712,#41713,#41714,#41715,
#41716,#41717,#41718,#41719,#41720,#41721,#41722,#41723,#41724,#41725,#41726,
#41727,#41728),.UNSPECIFIED.,.F.,.F.,(4,3,3,3,3,3,3,3,3,3,3,3,3,4),(-129.328364327577,
-129.197386586422,-128.698554977981,-128.199723369539,-127.700891761097,
-127.202060152655,-126.703228544213,-126.204396935772,-125.70556532733,
-125.206733718888,-124.707902110446,-124.209070502004,-123.710238893563,
-123.045179020398),.UNSPECIFIED.);
#280=B_SPLINE_CURVE_WITH_KNOTS('',3,(#41729,#41730,#41731,#41732,#41733,
#41734,#41735,#41736,#41737,#41738,#41739,#41740,#41741,#41742,#41743,#41744,
#41745,#41746,#41747,#41748,#41749,#41750,#41751,#41752,#41753,#41754,#41755,
#41756,#41757,#41758,#41759,#41760,#41761,#41762,#41763,#41764,#41765,#41766,
#41767,#41768,#41769,#41770,#41771),.UNSPECIFIED.,.F.,.F.,(4,3,3,3,3,3,
3,3,3,3,3,3,3,3,4),(119.817724070932,119.987257988362,120.487204896647,
120.987151804932,121.487098713217,121.987045621502,122.486992529787,122.986939438071,
123.486886346356,123.986833254641,124.486780162926,124.986727071211,125.486673979496,
125.98662088778,126.100909378111),.UNSPECIFIED.);
#281=B_SPLINE_CURVE_WITH_KNOTS('',3,(#41776,#41777,#41778,#41779,#41780,
#41781,#41782,#41783,#41784,#41785,#41786,#41787,#41788,#41789,#41790,#41791,
#41792,#41793,#41794,#41795,#41796,#41797,#41798,#41799,#41800,#41801,#41802,
#41803,#41804,#41805,#41806,#41807,#41808,#41809),.UNSPECIFIED.,.F.,.F.,
(4,3,3,3,3,3,3,3,3,3,3,4),(-135.611549634757,-134.684534279282,-134.18570267084,
-133.686871062398,-133.188039453957,-132.689207845515,-132.190376237073,
-131.691544628631,-131.192713020189,-130.693881411748,-129.696218194864,
-129.328364327577),.UNSPECIFIED.);
#282=B_SPLINE_CURVE_WITH_KNOTS('',3,(#41810,#41811,#41812,#41813,#41814,
#41815,#41816,#41817,#41818,#41819,#41820,#41821,#41822,#41823,#41824,#41825,
#41826,#41827,#41828,#41829,#41830,#41831,#41832,#41833,#41834,#41835,#41836,
#41837,#41838,#41839,#41840,#41841,#41842,#41843),.UNSPECIFIED.,.F.,.F.,
(4,3,3,3,3,3,3,3,3,3,3,4),(126.100909378111,126.486567796065,126.98651470435,
127.486461612635,127.98640852092,128.486355429205,128.98630233749,129.486249245774,
129.986196154059,130.986089970629,131.985983787199,132.384094685291),
 .UNSPECIFIED.);
#283=B_SPLINE_CURVE_WITH_KNOTS('',3,(#41848,#41849,#41850,#41851,#41852,
#41853,#41854,#41855,#41856,#41857,#41858,#41859,#41860,#41861,#41862,#41863,
#41864,#41865,#41866,#41867,#41868,#41869,#41870,#41871,#41872,#41873,#41874,
#41875,#41876,#41877,#41878,#41879,#41880,#41881,#41882,#41883,#41884,#41885,
#41886,#41887,#41888,#41889,#41890),.UNSPECIFIED.,.F.,.F.,(4,3,3,3,3,3,
3,3,3,3,3,3,3,3,4),(-141.894734941936,-141.668176797467,-141.169345189025,
-140.670513580583,-140.171681972142,-139.6728503637,-139.174018755258,-138.675187146816,
-138.176355538374,-137.677523929933,-137.178692321491,-136.679860713049,
-136.181029104607,-135.682197496165,-135.611549634757),.UNSPECIFIED.);
#284=B_SPLINE_CURVE_WITH_KNOTS('',3,(#41891,#41892,#41893,#41894,#41895,
#41896,#41897,#41898,#41899,#41900,#41901,#41902,#41903,#41904,#41905,#41906,
#41907,#41908,#41909,#41910,#41911,#41912,#41913,#41914,#41915,#41916,#41917,
#41918,#41919,#41920,#41921,#41922,#41923,#41924,#41925,#41926,#41927,#41928,
#41929,#41930,#41931,#41932,#41933),.UNSPECIFIED.,.F.,.F.,(4,3,3,3,3,3,
3,3,3,3,3,3,3,3,4),(132.384094685291,132.485930695483,132.985877603768,
133.485824512053,133.985771420338,134.485718328623,134.985665236908,135.485612145193,
135.985559053477,136.485505961762,136.985452870047,137.485399778332,137.985346686617,
138.485293594902,138.66727999247),.UNSPECIFIED.);
#285=B_SPLINE_CURVE_WITH_KNOTS('',3,(#41938,#41939,#41940,#41941,#41942,
#41943,#41944,#41945,#41946,#41947,#41948,#41949,#41950,#41951,#41952,#41953,
#41954,#41955,#41956,#41957,#41958,#41959,#41960,#41961,#41962,#41963,#41964,
#41965,#41966,#41967,#41968,#41969,#41970,#41971,#41972,#41973,#41974,#41975,
#41976,#41977),.UNSPECIFIED.,.F.,.F.,(4,3,3,3,3,3,3,3,3,3,3,3,3,4),(-148.177920249116,
-148.15298770721,-147.654156098768,-147.155324490327,-146.656492881885,
-146.157661273443,-145.658829665001,-145.159998056559,-144.661166448118,
-144.162334839676,-143.663503231234,-143.164671622792,-142.66584001435,
-141.894734941936),.UNSPECIFIED.);
#286=B_SPLINE_CURVE_WITH_KNOTS('',3,(#41978,#41979,#41980,#41981,#41982,
#41983,#41984,#41985,#41986,#41987,#41988,#41989,#41990,#41991,#41992,#41993,
#41994,#41995,#41996,#41997,#41998,#41999,#42000,#42001,#42002,#42003,#42004,
#42005,#42006,#42007,#42008,#42009,#42010,#42011,#42012,#42013,#42014,#42015,
#42016,#42017),.UNSPECIFIED.,.F.,.F.,(4,3,3,3,3,3,3,3,3,3,3,3,3,4),(138.66727999247,
138.985240503186,139.485187411471,139.985134319756,140.485081228041,140.985028136326,
141.484975044611,141.984921952895,142.48486886118,142.984815769465,143.48476267775,
143.984709586035,144.48465649432,144.95046529965),.UNSPECIFIED.);
#287=B_SPLINE_CURVE_WITH_KNOTS('',3,(#42022,#42023,#42024,#42025,#42026,
#42027,#42028,#42029,#42030,#42031,#42032,#42033,#42034,#42035,#42036,#42037,
#42038,#42039,#42040,#42041,#42042,#42043,#42044,#42045,#42046,#42047,#42048,
#42049,#42050,#42051,#42052,#42053,#42054,#42055,#42056,#42057,#42058),
 .UNSPECIFIED.,.F.,.F.,(4,3,3,3,3,3,3,3,3,3,3,3,4),(-154.461105556295,-154.138967008512,
-153.64013540007,-153.141303791628,-152.642472183186,-152.143640574744,
-151.644808966303,-151.145977357861,-150.647145749419,-150.148314140977,
-149.649482532535,-148.651819315652,-148.177920249116),.UNSPECIFIED.);
#288=B_SPLINE_CURVE_WITH_KNOTS('',3,(#42059,#42060,#42061,#42062,#42063,
#42064,#42065,#42066,#42067,#42068,#42069,#42070,#42071,#42072,#42073,#42074,
#42075,#42076,#42077,#42078,#42079,#42080,#42081,#42082,#42083,#42084,#42085,
#42086,#42087,#42088,#42089,#42090,#42091,#42092,#42093,#42094,#42095,#42096,
#42097,#42098,#42099,#42100,#42101),.UNSPECIFIED.,.F.,.F.,(4,3,3,3,3,3,
3,3,3,3,3,3,3,3,4),(144.95046529965,144.984603402604,145.484550310889,145.984497219174,
146.484444127459,146.984391035744,147.484337944029,147.984284852314,148.484231760598,
148.984178668883,149.484125577168,149.984072485453,150.484019393738,150.983966302023,
151.23365060683),.UNSPECIFIED.);
#289=B_SPLINE_CURVE_WITH_KNOTS('',3,(#42106,#42107,#42108,#42109,#42110,
#42111,#42112,#42113,#42114,#42115,#42116,#42117,#42118,#42119,#42120,#42121,
#42122,#42123,#42124,#42125,#42126,#42127,#42128,#42129,#42130,#42131,#42132,
#42133,#42134,#42135,#42136,#42137,#42138,#42139,#42140,#42141,#42142,#42143,
#42144,#42145),.UNSPECIFIED.,.F.,.F.,(4,3,3,3,3,3,3,3,3,3,3,3,3,4),(-160.744290863475,
-160.623777918255,-160.124946309813,-159.626114701371,-159.127283092929,
-158.628451484488,-158.129619876046,-157.630788267604,-157.131956659162,
-156.63312505072,-155.635461833837,-155.136630225395,-154.637798616953,
-154.461105556295),.UNSPECIFIED.);
#290=B_SPLINE_CURVE_WITH_KNOTS('',3,(#42146,#42147,#42148,#42149,#42150,
#42151,#42152,#42153,#42154,#42155,#42156,#42157,#42158,#42159,#42160,#42161,
#42162,#42163,#42164,#42165,#42166,#42167,#42168,#42169,#42170,#42171,#42172,
#42173,#42174,#42175,#42176,#42177,#42178,#42179,#42180,#42181,#42182,#42183,
#42184,#42185,#42186,#42187,#42188),.UNSPECIFIED.,.F.,.F.,(4,3,3,3,3,3,
3,3,3,3,3,3,3,3,4),(151.23365060683,151.483913210307,151.983860118592,152.483807026877,
152.983753935162,153.483700843447,153.983647751732,154.483594660017,154.983541568301,
155.483488476586,155.983435384871,156.483382293156,156.983329201441,157.483276109726,
157.516835914009),.UNSPECIFIED.);
#291=B_SPLINE_CURVE_WITH_KNOTS('',3,(#42193,#42194,#42195,#42196,#42197,
#42198,#42199,#42200,#42201,#42202,#42203,#42204,#42205,#42206,#42207,#42208,
#42209,#42210,#42211,#42212,#42213,#42214,#42215,#42216,#42217,#42218,#42219,
#42220,#42221,#42222,#42223,#42224,#42225,#42226,#42227,#42228,#42229),
 .UNSPECIFIED.,.F.,.F.,(4,3,3,3,3,3,3,3,3,3,3,3,4),(-167.027476170655,-166.609757219556,
-166.110925611114,-165.612094002673,-165.113262394231,-164.614430785789,
-164.115599177347,-163.616767568905,-162.619104352022,-162.12027274358,
-161.621441135138,-161.122609526696,-160.744290863475),.UNSPECIFIED.);
#292=B_SPLINE_CURVE_WITH_KNOTS('',3,(#42230,#42231,#42232,#42233,#42234,
#42235,#42236,#42237,#42238,#42239,#42240,#42241,#42242,#42243,#42244,#42245,
#42246,#42247,#42248,#42249,#42250,#42251,#42252,#42253,#42254,#42255,#42256,
#42257,#42258,#42259,#42260,#42261,#42262,#42263,#42264,#42265,#42266,#42267,
#42268,#42269),.UNSPECIFIED.,.F.,.F.,(4,3,3,3,3,3,3,3,3,3,3,3,3,4),(157.516835914009,
157.98322301801,158.483169926295,158.98311683458,159.483063742865,159.98301065115,
160.482957559435,160.98290446772,161.482851376004,161.982798284289,162.482745192574,
162.982692100859,163.482639009144,163.800021221189),.UNSPECIFIED.);
#293=B_SPLINE_CURVE_WITH_KNOTS('',3,(#42274,#42275,#42276,#42277,#42278,
#42279,#42280,#42281,#42282,#42283,#42284,#42285,#42286,#42287,#42288,#42289,
#42290,#42291,#42292,#42293,#42294,#42295,#42296,#42297,#42298),
 .UNSPECIFIED.,.F.,.F.,(4,3,3,3,3,3,3,3,4),(-173.310661477834,-172.521767800485,
-171.732874123137,-170.943980445788,-170.155086768439,-169.36619309109,
-168.577299413742,-167.788405736393,-167.027476170655),.UNSPECIFIED.);
#294=B_SPLINE_CURVE_WITH_KNOTS('',3,(#42299,#42300,#42301,#42302,#42303,
#42304,#42305,#42306,#42307,#42308,#42309,#42310,#42311,#42312,#42313,#42314,
#42315,#42316,#42317,#42318,#42319,#42320,#42321,#42322,#42323,#42324,#42325,
#42326,#42327,#42328,#42329,#42330,#42331,#42332,#42333,#42334,#42335,#42336,
#42337,#42338,#42339,#42340,#42341),.UNSPECIFIED.,.F.,.F.,(4,3,3,3,3,3,
3,3,3,3,3,3,3,3,4),(163.800021221189,163.982585917429,164.482532825713,
164.982479733998,165.482426642283,165.982373550568,166.482320458853,166.982267367138,
167.482214275422,167.982161183707,168.482108091992,168.982055000277,169.482001908562,
169.981948816847,170.083206528368),.UNSPECIFIED.);
#295=B_SPLINE_CURVE_WITH_KNOTS('',3,(#42346,#42347,#42348,#42349,#42350,
#42351,#42352,#42353,#42354,#42355,#42356,#42357,#42358,#42359,#42360,#42361,
#42362,#42363,#42364,#42365,#42366,#42367,#42368,#42369,#42370),
 .UNSPECIFIED.,.F.,.F.,(4,3,3,3,3,3,3,3,4),(-179.593846785014,-178.804953107665,
-178.016059430316,-177.227165752967,-176.438272075619,-175.64937839827,
-174.860484720921,-174.071591043572,-173.310661477834),.UNSPECIFIED.);
#296=B_SPLINE_CURVE_WITH_KNOTS('',3,(#42371,#42372,#42373,#42374,#42375,
#42376,#42377,#42378,#42379,#42380,#42381,#42382,#42383,#42384,#42385,#42386,
#42387,#42388,#42389,#42390,#42391,#42392,#42393,#42394,#42395,#42396,#42397,
#42398,#42399,#42400,#42401,#42402,#42403,#42404,#42405,#42406,#42407,#42408,
#42409,#42410),.UNSPECIFIED.,.F.,.F.,(4,3,3,3,3,3,3,3,3,3,3,3,3,4),(170.083206528368,
170.481895725131,170.981842633416,171.481789541701,171.981736449986,172.481683358271,
172.981630266556,173.481577174841,173.981524083125,174.48147099141,174.981417899695,
175.48136480798,175.981311716265,176.366391835548),.UNSPECIFIED.);
#297=B_SPLINE_CURVE_WITH_KNOTS('',3,(#42415,#42416,#42417,#42418,#42419,
#42420,#42421,#42422,#42423,#42424,#42425,#42426,#42427,#42428,#42429,#42430,
#42431,#42432,#42433,#42434,#42435,#42436,#42437,#42438,#42439,#42440,#42441,
#42442,#42443,#42444,#42445,#42446,#42447,#42448,#42449,#42450,#42451),
 .UNSPECIFIED.,.F.,.F.,(4,3,3,3,3,3,3,3,3,3,3,3,4),(-185.877032092193,-185.565358340344,
-185.066526731902,-184.56769512346,-183.570031906577,-183.071200298135,
-182.572368689693,-182.073537081251,-181.57470547281,-181.075873864368,
-180.577042255926,-180.078210647484,-179.593846785014),.UNSPECIFIED.);
#298=B_SPLINE_CURVE_WITH_KNOTS('',3,(#42452,#42453,#42454,#42455,#42456,
#42457,#42458,#42459,#42460,#42461,#42462,#42463,#42464,#42465,#42466,#42467,
#42468,#42469,#42470,#42471,#42472,#42473,#42474,#42475,#42476,#42477,#42478,
#42479,#42480,#42481,#42482,#42483,#42484,#42485,#42486,#42487,#42488,#42489,
#42490,#42491,#42492,#42493,#42494),.UNSPECIFIED.,.F.,.F.,(4,3,3,3,3,3,
3,3,3,3,3,3,3,3,4),(176.366391835548,176.48125862455,176.981205532834,177.481152441119,
177.981099349404,178.481046257689,178.980993165974,179.480940074259,179.980886982544,
180.480833890828,180.980780799113,181.480727707398,181.980674615683,182.480621523968,
182.649577142727),.UNSPECIFIED.);
#299=B_SPLINE_CURVE_WITH_KNOTS('',3,(#42499,#42500,#42501,#42502,#42503,
#42504,#42505,#42506,#42507,#42508,#42509,#42510,#42511,#42512,#42513,#42514,
#42515,#42516,#42517,#42518,#42519,#42520,#42521,#42522,#42523,#42524,#42525,
#42526,#42527,#42528,#42529,#42530,#42531,#42532,#42533,#42534,#42535,#42536,
#42537,#42538),.UNSPECIFIED.,.F.,.F.,(4,3,3,3,3,3,3,3,3,3,3,3,3,4),(-192.160217399373,
-192.050169250087,-191.551337641645,-190.553674424762,-190.05484281632,
-189.556011207878,-189.057179599436,-188.558347990995,-188.059516382553,
-187.560684774111,-187.061853165669,-186.563021557228,-186.064189948786,
-185.877032092193),.UNSPECIFIED.);
#300=B_SPLINE_CURVE_WITH_KNOTS('',3,(#42539,#42540,#42541,#42542,#42543,
#42544,#42545,#42546,#42547,#42548,#42549,#42550,#42551,#42552,#42553,#42554,
#42555,#42556,#42557,#42558,#42559,#42560,#42561,#42562,#42563,#42564,#42565,
#42566,#42567,#42568,#42569,#42570,#42571,#42572,#42573,#42574,#42575,#42576,
#42577,#42578),.UNSPECIFIED.,.F.,.F.,(4,3,3,3,3,3,3,3,3,3,3,3,3,4),(182.649577142727,
182.980568432253,183.480515340537,183.980462248822,184.480409157107,184.980356065392,
185.480302973677,185.980249881962,186.480196790247,186.980143698531,187.480090606816,
187.980037515101,188.479984423386,188.932762449907),.UNSPECIFIED.);
#301=B_SPLINE_CURVE_WITH_KNOTS('',3,(#42583,#42584,#42585,#42586,#42587,
#42588,#42589,#42590,#42591,#42592,#42593,#42594,#42595,#42596,#42597,#42598,
#42599,#42600,#42601,#42602,#42603,#42604,#42605,#42606,#42607,#42608,#42609,
#42610,#42611,#42612,#42613,#42614,#42615,#42616,#42617,#42618,#42619),
 .UNSPECIFIED.,.F.,.F.,(4,3,3,3,3,3,3,3,3,3,3,3,4),(-198.443402706552,-197.537316942947,
-197.038485334505,-196.539653726063,-196.040822117621,-195.54199050918,
-195.043158900738,-194.544327292296,-194.045495683854,-193.546664075412,
-193.047832466971,-192.549000858529,-192.160217399373),.UNSPECIFIED.);
#302=B_SPLINE_CURVE_WITH_KNOTS('',3,(#42620,#42621,#42622,#42623,#42624,
#42625,#42626,#42627,#42628,#42629,#42630,#42631,#42632,#42633,#42634,#42635,
#42636,#42637,#42638,#42639,#42640,#42641,#42642,#42643,#42644,#42645,#42646,
#42647,#42648,#42649,#42650,#42651,#42652,#42653,#42654,#42655,#42656,#42657,
#42658,#42659,#42660,#42661,#42662),.UNSPECIFIED.,.F.,.F.,(4,3,3,3,3,3,
3,3,3,3,3,3,3,3,4),(188.932762449907,188.979931331671,189.479878239956,
189.97982514824,190.479772056525,190.97971896481,191.479665873095,191.97961278138,
192.479559689665,192.979506597949,193.479453506234,193.979400414519,194.479347322804,
194.979294231089,195.215947757087),.UNSPECIFIED.);
#303=B_SPLINE_CURVE_WITH_KNOTS('',3,(#42667,#42668,#42669,#42670,#42671,
#42672,#42673,#42674,#42675,#42676,#42677,#42678,#42679,#42680,#42681,#42682,
#42683,#42684,#42685,#42686,#42687,#42688,#42689,#42690,#42691,#42692,#42693,
#42694,#42695,#42696,#42697,#42698,#42699,#42700,#42701,#42702,#42703,#42704,
#42705,#42706,#42707,#42708,#42709),.UNSPECIFIED.,.F.,.F.,(4,3,3,3,3,3,
3,3,3,3,3,3,3,3,4),(-204.726588013732,-204.520959461132,-204.02212785269,
-203.523296244248,-203.024464635806,-202.525633027365,-202.026801418923,
-201.527969810481,-201.029138202039,-200.530306593597,-200.031474985156,
-199.532643376714,-199.033811768272,-198.53498015983,-198.443402706552),
 .UNSPECIFIED.);
#304=B_SPLINE_CURVE_WITH_KNOTS('',3,(#42710,#42711,#42712,#42713,#42714,
#42715,#42716,#42717,#42718,#42719,#42720,#42721,#42722,#42723,#42724,#42725,
#42726,#42727,#42728,#42729,#42730,#42731,#42732,#42733,#42734,#42735,#42736,
#42737,#42738,#42739,#42740,#42741,#42742,#42743,#42744,#42745,#42746,#42747,
#42748,#42749,#42750,#42751,#42752),.UNSPECIFIED.,.F.,.F.,(4,3,3,3,3,3,
3,3,3,3,3,3,3,3,4),(195.215947757087,195.479241139374,195.979188047659,
196.479134955943,196.979081864228,197.479028772513,197.978975680798,198.478922589083,
198.978869497368,199.478816405652,199.978763313937,200.478710222222,200.978657130507,
201.478604038792,201.499133064266),.UNSPECIFIED.);
#305=B_SPLINE_CURVE_WITH_KNOTS('',3,(#42757,#42758,#42759,#42760,#42761,
#42762,#42763,#42764,#42765,#42766,#42767,#42768,#42769,#42770,#42771,#42772,
#42773,#42774,#42775,#42776,#42777,#42778,#42779,#42780,#42781,#42782,#42783,
#42784,#42785,#42786,#42787,#42788,#42789,#42790,#42791,#42792,#42793,#42794,
#42795,#42796),.UNSPECIFIED.,.F.,.F.,(4,3,3,3,3,3,3,3,3,3,3,3,3,4),(-211.009773320912,
-211.005770370875,-210.506938762433,-210.008107153991,-209.50927554555,
-209.010443937108,-208.511612328666,-208.012780720224,-207.513949111782,
-207.015117503341,-206.516285894899,-206.017454286457,-205.518622678015,
-204.726588013732),.UNSPECIFIED.);
#306=B_SPLINE_CURVE_WITH_KNOTS('',3,(#42797,#42798,#42799,#42800,#42801,
#42802,#42803,#42804,#42805,#42806,#42807,#42808,#42809,#42810,#42811,#42812,
#42813,#42814,#42815,#42816,#42817,#42818,#42819,#42820,#42821,#42822,#42823,
#42824,#42825,#42826,#42827,#42828,#42829,#42830,#42831,#42832,#42833,#42834,
#42835,#42836),.UNSPECIFIED.,.F.,.F.,(4,3,3,3,3,3,3,3,3,3,3,3,3,4),(201.499133064266,
201.978550947077,202.478497855361,202.978444763646,203.478391671931,203.978338580216,
204.478285488501,204.978232396786,205.478179305071,205.978126213355,206.47807312164,
206.978020029925,207.47796693821,207.782318371446),.UNSPECIFIED.);
#307=B_SPLINE_CURVE_WITH_KNOTS('',3,(#42841,#42842,#42843,#42844,#42845,
#42846,#42847,#42848,#42849,#42850,#42851,#42852,#42853,#42854,#42855,#42856,
#42857,#42858,#42859,#42860,#42861,#42862,#42863,#42864,#42865,#42866,#42867,
#42868,#42869,#42870,#42871,#42872,#42873,#42874,#42875,#42876,#42877),
 .UNSPECIFIED.,.F.,.F.,(4,3,3,3,3,3,3,3,3,3,3,3,4),(-217.292958628091,-216.991749672176,
-216.492918063735,-215.994086455293,-215.495254846851,-214.996423238409,
-214.497591629967,-213.998760021526,-213.499928413084,-213.001096804642,
-212.5022651962,-211.504601979317,-211.009773320912),.UNSPECIFIED.);
#308=B_SPLINE_CURVE_WITH_KNOTS('',3,(#42878,#42879,#42880,#42881,#42882,
#42883,#42884,#42885,#42886,#42887,#42888,#42889,#42890,#42891,#42892,#42893,
#42894,#42895,#42896,#42897,#42898,#42899,#42900,#42901,#42902,#42903,#42904,
#42905,#42906,#42907,#42908,#42909,#42910,#42911,#42912,#42913,#42914,#42915,
#42916,#42917,#42918,#42919,#42920),.UNSPECIFIED.,.F.,.F.,(4,3,3,3,3,3,
3,3,3,3,3,3,3,3,4),(207.782318371446,207.977913846495,208.47786075478,208.977807663065,
209.477754571349,209.977701479634,210.477648387919,210.977595296204,211.477542204489,
211.977489112774,212.477436021058,212.977382929343,213.477329837628,213.977276745913,
214.065503678625),.UNSPECIFIED.);
#309=B_SPLINE_CURVE_WITH_KNOTS('',3,(#42925,#42926,#42927,#42928,#42929,
#42930,#42931,#42932,#42933,#42934,#42935,#42936,#42937,#42938,#42939,#42940,
#42941,#42942,#42943,#42944,#42945,#42946,#42947,#42948,#42949,#42950,#42951,
#42952,#42953,#42954,#42955,#42956,#42957,#42958,#42959,#42960,#42961,#42962,
#42963,#42964),.UNSPECIFIED.,.F.,.F.,(4,3,3,3,3,3,3,3,3,3,3,3,3,4),(-223.576143935271,
-223.47656058192,-222.977728973478,-222.478897365036,-221.980065756594,
-221.481234148152,-220.982402539711,-220.483570931269,-219.984739322827,
-219.485907714385,-218.488244497502,-217.98941288906,-217.490581280618,
-217.292958628091),.UNSPECIFIED.);
#310=B_SPLINE_CURVE_WITH_KNOTS('',3,(#42965,#42966,#42967,#42968,#42969,
#42970,#42971,#42972,#42973,#42974,#42975,#42976,#42977,#42978,#42979,#42980,
#42981,#42982,#42983,#42984,#42985,#42986,#42987,#42988,#42989,#42990,#42991,
#42992,#42993,#42994,#42995,#42996,#42997,#42998,#42999,#43000,#43001,#43002,
#43003,#43004),.UNSPECIFIED.,.F.,.F.,(4,3,3,3,3,3,3,3,3,3,3,3,3,4),(214.065503678625,
214.477223654198,214.977170562483,215.477117470767,215.977064379052,216.477011287337,
216.976958195622,217.476905103907,217.976852012192,218.476798920477,218.976745828761,
219.476692737046,219.976639645331,220.348688985805),.UNSPECIFIED.);
#311=B_SPLINE_CURVE_WITH_KNOTS('',3,(#43009,#43010,#43011,#43012,#43013,
#43014,#43015,#43016,#43017,#43018,#43019,#43020,#43021,#43022,#43023,#43024,
#43025,#43026,#43027,#43028,#43029,#43030,#43031,#43032,#43033,#43034,#43035,
#43036,#43037,#43038,#43039,#43040,#43041,#43042,#43043,#43044,#43045),
 .UNSPECIFIED.,.F.,.F.,(4,3,3,3,3,3,3,3,3,3,3,3,4),(-229.85932924245,-229.462539883221,
-228.963708274779,-228.464876666337,-227.966045057896,-227.467213449454,
-226.968381841012,-226.46955023257,-225.471887015687,-224.973055407245,
-224.474223798803,-223.975392190361,-223.576143935271),.UNSPECIFIED.);
#312=B_SPLINE_CURVE_WITH_KNOTS('',3,(#43046,#43047,#43048,#43049,#43050,
#43051,#43052,#43053,#43054,#43055,#43056,#43057,#43058,#43059,#43060,#43061,
#43062,#43063,#43064,#43065,#43066,#43067,#43068,#43069,#43070,#43071,#43072,
#43073,#43074,#43075,#43076,#43077,#43078,#43079,#43080,#43081,#43082,#43083,
#43084,#43085,#43086,#43087,#43088),.UNSPECIFIED.,.F.,.F.,(4,3,3,3,3,3,
3,3,3,3,3,3,3,3,4),(220.348688985805,220.476586553616,220.976533461901,
221.476480370186,221.97642727847,222.476374186755,222.97632109504,223.476268003325,
223.97621491161,224.476161819895,224.976108728179,225.476055636464,225.976002544749,
226.475949453034,226.631874292984),.UNSPECIFIED.);
#313=B_SPLINE_CURVE_WITH_KNOTS('',3,(#43093,#43094,#43095,#43096,#43097,
#43098,#43099,#43100,#43101,#43102,#43103,#43104,#43105,#43106,#43107,#43108,
#43109,#43110,#43111,#43112,#43113,#43114,#43115,#43116,#43117),
 .UNSPECIFIED.,.F.,.F.,(4,3,3,3,3,3,3,3,4),(-236.14251454963,-235.353620872281,
-234.564727194932,-233.775833517583,-232.986939840235,-232.198046162886,
-231.409152485537,-230.620258808188,-229.85932924245),.UNSPECIFIED.);
#314=B_SPLINE_CURVE_WITH_KNOTS('',3,(#43118,#43119,#43120,#43121,#43122,
#43123,#43124,#43125,#43126,#43127,#43128,#43129,#43130,#43131,#43132,#43133,
#43134,#43135,#43136,#43137,#43138,#43139,#43140,#43141,#43142,#43143,#43144,
#43145,#43146,#43147,#43148,#43149,#43150,#43151,#43152,#43153,#43154,#43155,
#43156,#43157),.UNSPECIFIED.,.F.,.F.,(4,3,3,3,3,3,3,3,3,3,3,3,3,4),(226.631874292984,
226.975896361319,227.475843269604,227.975790177889,228.475737086173,228.975683994458,
229.475630902743,229.975577811028,230.475524719313,230.975471627598,231.475418535882,
231.975365444167,232.475312352452,232.915059600164),.UNSPECIFIED.);
#315=B_SPLINE_CURVE_WITH_KNOTS('',3,(#43162,#43163,#43164,#43165,#43166,
#43167,#43168,#43169,#43170,#43171,#43172,#43173,#43174,#43175,#43176,#43177,
#43178,#43179,#43180,#43181,#43182,#43183,#43184,#43185,#43186,#43187,#43188,
#43189,#43190,#43191,#43192,#43193,#43194,#43195,#43196,#43197,#43198),
 .UNSPECIFIED.,.F.,.F.,(4,3,3,3,3,3,3,3,3,3,3,3,4),(-242.425699856809,-241.933330094266,
-241.434498485824,-240.935666877382,-240.43683526894,-239.439172052057,
-238.940340443615,-238.441508835173,-237.942677226731,-237.44384561829,
-236.945014009848,-236.446182401406,-236.14251454963),.UNSPECIFIED.);
#316=B_SPLINE_CURVE_WITH_KNOTS('',3,(#43199,#43200,#43201,#43202,#43203,
#43204,#43205,#43206,#43207,#43208,#43209,#43210,#43211,#43212,#43213,#43214,
#43215,#43216,#43217,#43218,#43219,#43220,#43221,#43222,#43223,#43224,#43225,
#43226,#43227,#43228,#43229,#43230,#43231,#43232,#43233,#43234,#43235,#43236,
#43237,#43238,#43239,#43240,#43241),.UNSPECIFIED.,.F.,.F.,(4,3,3,3,3,3,
3,3,3,3,3,3,3,3,4),(232.915059600164,232.975259260737,233.475206169022,
233.975153077307,234.475099985591,234.975046893876,235.474993802161,235.974940710446,
236.474887618731,236.974834527016,237.474781435301,237.974728343585,238.47467525187,
238.974622160155,239.198244907343),.UNSPECIFIED.);
#317=B_SPLINE_CURVE_WITH_KNOTS('',3,(#43246,#43247,#43248,#43249,#43250,
#43251,#43252,#43253,#43254,#43255,#43256,#43257,#43258,#43259,#43260,#43261,
#43262,#43263,#43264,#43265,#43266,#43267,#43268,#43269,#43270,#43271,#43272,
#43273,#43274,#43275,#43276,#43277,#43278,#43279,#43280,#43281,#43282,#43283,
#43284,#43285),.UNSPECIFIED.,.F.,.F.,(4,3,3,3,3,3,3,3,3,3,3,3,3,4),(-248.708885163989,
-248.418141004009,-247.919309395567,-247.420477787125,-246.422814570242,
-245.9239829618,-245.425151353358,-244.926319744916,-244.427488136475,-243.928656528033,
-243.429824919591,-242.930993311149,-242.432161702707,-242.425699856809),
 .UNSPECIFIED.);
#318=B_SPLINE_CURVE_WITH_KNOTS('',3,(#43286,#43287,#43288,#43289,#43290,
#43291,#43292,#43293,#43294,#43295,#43296,#43297,#43298,#43299,#43300,#43301,
#43302,#43303,#43304,#43305,#43306,#43307,#43308,#43309,#43310,#43311,#43312,
#43313,#43314,#43315,#43316,#43317,#43318,#43319,#43320,#43321,#43322,#43323,
#43324,#43325,#43326,#43327,#43328),.UNSPECIFIED.,.F.,.F.,(4,3,3,3,3,3,
3,3,3,3,3,3,3,3,4),(239.198244907343,239.47456906844,239.974515976725,240.47446288501,
240.974409793294,241.474356701579,241.974303609864,242.474250518149,242.974197426434,
243.474144334719,243.974091243004,244.474038151288,244.973985059573,245.473931967858,
245.481430214523),.UNSPECIFIED.);
#319=B_SPLINE_CURVE_WITH_KNOTS('',3,(#43333,#43334,#43335,#43336,#43337,
#43338,#43339,#43340,#43341,#43342,#43343,#43344,#43345,#43346,#43347,#43348,
#43349,#43350,#43351,#43352,#43353,#43354,#43355,#43356,#43357,#43358,#43359,
#43360,#43361,#43362,#43363,#43364,#43365,#43366,#43367,#43368,#43369,#43370,
#43371,#43372),.UNSPECIFIED.,.F.,.F.,(4,3,3,3,3,3,3,3,3,3,3,3,3,4),(-254.992070471168,
-254.902951913752,-254.40412030531,-253.406457088427,-252.907625479985,
-252.408793871543,-251.909962263101,-251.41113065466,-250.912299046218,
-250.413467437776,-249.914635829334,-249.415804220892,-248.916972612451,
-248.708885163989),.UNSPECIFIED.);
#320=B_SPLINE_CURVE_WITH_KNOTS('',3,(#43373,#43374,#43375,#43376,#43377,
#43378,#43379,#43380,#43381,#43382,#43383,#43384,#43385,#43386,#43387,#43388,
#43389,#43390,#43391,#43392,#43393,#43394,#43395,#43396,#43397,#43398,#43399,
#43400,#43401,#43402,#43403,#43404,#43405,#43406,#43407,#43408,#43409,#43410,
#43411,#43412),.UNSPECIFIED.,.F.,.F.,(4,3,3,3,3,3,3,3,3,3,3,3,3,4),(245.481430214523,
245.973878876143,246.473825784428,246.973772692713,247.473719600997,247.973666509282,
248.473613417567,248.973560325852,249.473507234137,249.973454142422,250.473401050706,
250.973347958991,251.473294867276,251.764615521703),.UNSPECIFIED.);
#321=B_SPLINE_CURVE_WITH_KNOTS('',3,(#43417,#43418,#43419,#43420,#43421,
#43422,#43423,#43424,#43425,#43426,#43427,#43428,#43429,#43430,#43431,#43432,
#43433,#43434,#43435,#43436,#43437,#43438,#43439,#43440,#43441,#43442,#43443,
#43444,#43445,#43446,#43447,#43448,#43449,#43450,#43451,#43452,#43453),
 .UNSPECIFIED.,.F.,.F.,(4,3,3,3,3,3,3,3,3,3,3,3,4),(-261.275255778348,-260.390099606612,
-259.89126799817,-259.392436389728,-258.893604781286,-258.394773172845,
-257.895941564403,-257.397109955961,-256.898278347519,-256.399446739077,
-255.900615130636,-255.401783522194,-254.992070471168),.UNSPECIFIED.);
#322=B_SPLINE_CURVE_WITH_KNOTS('',3,(#43454,#43455,#43456,#43457,#43458,
#43459,#43460,#43461,#43462,#43463,#43464,#43465,#43466,#43467,#43468,#43469,
#43470,#43471,#43472,#43473,#43474,#43475,#43476,#43477,#43478,#43479,#43480,
#43481,#43482,#43483,#43484,#43485,#43486,#43487,#43488,#43489,#43490,#43491,
#43492,#43493,#43494,#43495,#43496),.UNSPECIFIED.,.F.,.F.,(4,3,3,3,3,3,
3,3,3,3,3,3,3,3,4),(251.764615521703,251.973241775561,252.473188683846,
252.973135592131,253.473082500416,253.9730294087,254.472976316985,254.97292322527,
255.472870133555,255.97281704184,256.472763950125,256.972710858409,257.472657766694,
257.972604674979,258.047800828882),.UNSPECIFIED.);
#323=B_SPLINE_CURVE_WITH_KNOTS('',3,(#43502,#43503,#43504,#43505,#43506,
#43507,#43508,#43509,#43510,#43511),.UNSPECIFIED.,.F.,.F.,(4,1,1,1,1,1,
1,4),(273.318560862312,273.431067907459,273.929899515901,274.428731124343,
274.927562732785,275.426394341226,275.925225949668,276.054897710016),
 .UNSPECIFIED.);
#324=B_SPLINE_CURVE_WITH_KNOTS('',3,(#43514,#43515,#43516,#43517,#43518),
 .UNSPECIFIED.,.F.,.F.,(4,1,4),(273.318560862312,273.459489208933,273.959436117218),
 .UNSPECIFIED.);
#325=B_SPLINE_CURVE_WITH_KNOTS('',3,(#43523,#43524,#43525,#43526,#43527,
#43528,#43529,#43530,#43531,#43532,#43533,#43534,#43535,#43536,#43537),
 .UNSPECIFIED.,.F.,.F.,(4,1,1,1,1,1,1,1,1,1,1,1,4),(267.035375555132,267.445088606158,
267.9439202146,268.442751823041,268.941583431483,269.440415039925,269.939246648367,
270.438078256808,270.93690986525,271.435741473692,271.934573082134,272.433404690576,
273.318560862312),.UNSPECIFIED.);
#326=B_SPLINE_CURVE_WITH_KNOTS('',3,(#43538,#43539,#43540,#43541,#43542,
#43543,#43544,#43545,#43546,#43547,#43548,#43549,#43550,#43551,#43552,#43553),
 .UNSPECIFIED.,.F.,.F.,(4,1,1,1,1,1,1,1,1,1,1,1,1,4),(267.035375555132,
267.460126309515,267.9600732178,268.460020126084,268.959967034369,269.459913942654,
269.959860850939,270.459807759224,270.959754667509,271.459701575793,271.959648484078,
272.459595392363,272.959542300648,273.318560862312),.UNSPECIFIED.);
#327=B_SPLINE_CURVE_WITH_KNOTS('',3,(#43558,#43559,#43560,#43561,#43562,
#43563,#43564,#43565,#43566,#43567,#43568,#43569,#43570,#43571,#43572,#43573),
 .UNSPECIFIED.,.F.,.F.,(4,1,1,1,1,1,1,1,1,1,1,1,1,4),(260.752190247953,
260.960277696415,261.459109304856,261.957940913298,262.45677252174,262.955604130182,
263.454435738623,263.953267347065,264.452098955507,264.950930563949,265.449762172391,
266.447425389274,266.946256997716,267.035375555132),.UNSPECIFIED.);
#328=B_SPLINE_CURVE_WITH_KNOTS('',3,(#43574,#43575,#43576,#43577,#43578,
#43579,#43580,#43581,#43582,#43583,#43584,#43585,#43586,#43587,#43588,#43589,
#43590),.UNSPECIFIED.,.F.,.F.,(4,1,1,1,1,1,1,1,1,1,1,1,1,1,4),(260.752190247953,
260.960816501812,261.460763410097,261.960710318381,262.460657226666,262.960604134951,
263.460551043236,263.960497951521,264.460444859806,264.96039176809,265.460338676375,
265.96028558466,266.460232492945,266.96017940123,267.035375555132),
 .UNSPECIFIED.);
#329=B_SPLINE_CURVE_WITH_KNOTS('',3,(#43595,#43596,#43597,#43598,#43599,
#43600,#43601,#43602,#43603,#43604,#43605,#43606,#43607,#43608,#43609,#43610),
 .UNSPECIFIED.,.F.,.F.,(4,1,1,1,1,1,1,1,1,1,1,1,1,4),(254.469004940773,
254.475466786671,254.974298395113,255.473130003555,255.971961611997,256.470793220438,
256.96962482888,257.468456437322,257.967288045764,258.466119654206,259.463782871089,
259.962614479531,260.461446087973,260.752190247953),.UNSPECIFIED.);
#330=B_SPLINE_CURVE_WITH_KNOTS('',3,(#43611,#43612,#43613,#43614,#43615,
#43616,#43617,#43618,#43619,#43620,#43621,#43622,#43623,#43624,#43625,#43626),
 .UNSPECIFIED.,.F.,.F.,(4,1,1,1,1,1,1,1,1,1,1,1,1,4),(254.469004940773,
254.961453602394,255.461400510678,255.961347418963,256.461294327248,256.961241235533,
257.461188143818,257.961135052103,258.461081960387,258.961028868672,259.460975776957,
259.960922685242,260.460869593527,260.752190247953),.UNSPECIFIED.);
#331=B_SPLINE_CURVE_WITH_KNOTS('',3,(#43631,#43632,#43633,#43634,#43635,
#43636,#43637,#43638,#43639,#43640,#43641,#43642,#43643,#43644,#43645),
 .UNSPECIFIED.,.F.,.F.,(4,1,1,1,1,1,1,1,1,1,1,1,4),(248.185819633594,248.48948748537,
248.988319093812,249.487150702254,249.985982310695,250.484813919137,250.983645527579,
251.482477136021,252.480140352904,252.978971961346,253.477803569788,253.97663517823,
254.469004940773),.UNSPECIFIED.);
#332=B_SPLINE_CURVE_WITH_KNOTS('',3,(#43646,#43647,#43648,#43649,#43650,
#43651,#43652,#43653,#43654,#43655,#43656,#43657,#43658,#43659,#43660,#43661,
#43662),.UNSPECIFIED.,.F.,.F.,(4,1,1,1,1,1,1,1,1,1,1,1,1,1,4),(248.185819633594,
248.462143794691,248.962090702975,249.46203761126,249.961984519545,250.46193142783,
250.961878336115,251.4618252444,251.961772152685,252.461719060969,252.961665969254,
253.461612877539,253.961559785824,254.461506694109,254.469004940773),
 .UNSPECIFIED.);
#333=B_SPLINE_CURVE_WITH_KNOTS('',3,(#43667,#43668,#43669,#43670,#43671,
#43672,#43673,#43674,#43675,#43676,#43677,#43678,#43679,#43680,#43681,#43682,
#43683,#43684,#43685,#43686,#43687,#43688,#43689,#43690,#43691),
 .UNSPECIFIED.,.F.,.F.,(4,3,3,3,3,3,3,3,4),(241.902634326414,242.744762189266,
243.586890052118,244.42901791497,245.271145777822,246.113273640674,246.955401503526,
247.797529366378,248.185819633594),.UNSPECIFIED.);
#334=B_SPLINE_CURVE_WITH_KNOTS('',3,(#43692,#43693,#43694,#43695,#43696,
#43697,#43698,#43699,#43700,#43701,#43702,#43703,#43704,#43705,#43706,#43707,
#43708),.UNSPECIFIED.,.F.,.F.,(4,1,1,1,1,1,1,1,1,1,1,1,1,1,4),(241.902634326414,
241.962833986988,242.462780895273,242.962727803557,243.462674711842,243.962621620127,
244.462568528412,244.962515436697,245.462462344982,245.962409253266,246.462356161551,
246.962303069836,247.462249978121,247.962196886406,248.185819633594),
 .UNSPECIFIED.);
#335=B_SPLINE_CURVE_WITH_KNOTS('',3,(#43713,#43714,#43715,#43716,#43717,
#43718,#43719,#43720,#43721,#43722,#43723,#43724,#43725,#43726,#43727),
 .UNSPECIFIED.,.F.,.F.,(4,1,1,1,1,1,1,1,1,1,1,1,4),(235.619449019234,236.018697274325,
236.517528882767,237.016360491209,237.515192099651,238.512855316534,239.011686924976,
239.510518533418,240.00935014186,240.508181750301,241.007013358743,241.505844967185,
241.902634326414),.UNSPECIFIED.);
#336=B_SPLINE_CURVE_WITH_KNOTS('',3,(#43728,#43729,#43730,#43731,#43732,
#43733,#43734,#43735,#43736,#43737,#43738,#43739,#43740,#43741,#43742,#43743),
 .UNSPECIFIED.,.F.,.F.,(4,1,1,1,1,1,1,1,1,1,1,1,1,4),(235.619449019235,
235.96347108757,236.463417995854,236.963364904139,237.463311812424,237.963258720709,
238.463205628994,238.963152537279,239.463099445563,239.963046353848,240.462993262133,
240.962940170418,241.462887078703,241.902634326414),.UNSPECIFIED.);
#337=B_SPLINE_CURVE_WITH_KNOTS('',3,(#43748,#43749,#43750,#43751,#43752,
#43753,#43754,#43755,#43756,#43757,#43758,#43759,#43760,#43761,#43762,#43763),
 .UNSPECIFIED.,.F.,.F.,(4,1,1,1,1,1,1,1,1,1,1,1,1,4),(229.336263712055,
229.533886364582,230.032717973024,230.531549581466,231.529212798349,232.028044406791,
232.526876015233,233.025707623675,233.524539232116,234.023370840558,234.522202449,
235.021034057442,235.519865665884,235.619449019234),.UNSPECIFIED.);
#338=B_SPLINE_CURVE_WITH_KNOTS('',3,(#43764,#43765,#43766,#43767,#43768,
#43769,#43770,#43771,#43772,#43773,#43774,#43775,#43776,#43777,#43778,#43779,
#43780),.UNSPECIFIED.,.F.,.F.,(4,1,1,1,1,1,1,1,1,1,1,1,1,1,4),(229.336263712055,
229.464161279867,229.964108188151,230.464055096436,230.964002004721,231.463948913006,
231.963895821291,232.463842729576,232.96378963786,233.463736546145,233.96368345443,
234.463630362715,234.963577271,235.463524179285,235.619449019235),
 .UNSPECIFIED.);
#339=B_SPLINE_CURVE_WITH_KNOTS('',3,(#43785,#43786,#43787,#43788,#43789,
#43790,#43791,#43792,#43793,#43794,#43795,#43796,#43797,#43798,#43799),
 .UNSPECIFIED.,.F.,.F.,(4,1,1,1,1,1,1,1,1,1,1,1,4),(223.053078404875,223.547907063281,
224.545570280164,225.044401888606,225.543233497048,226.04206510549,226.540896713931,
227.039728322373,227.538559930815,228.037391539257,228.536223147699,229.03505475614,
229.336263712055),.UNSPECIFIED.);
#340=B_SPLINE_CURVE_WITH_KNOTS('',3,(#43800,#43801,#43802,#43803,#43804,
#43805,#43806,#43807,#43808,#43809,#43810,#43811,#43812,#43813,#43814,#43815),
 .UNSPECIFIED.,.F.,.F.,(4,1,1,1,1,1,1,1,1,1,1,1,1,4),(223.053078404875,
223.464798380448,223.964745288733,224.464692197018,224.964639105303,225.464586013588,
225.964532921873,226.464479830158,226.964426738442,227.464373646727,227.964320555012,
228.464267463297,228.964214371582,229.336263712055),.UNSPECIFIED.);
#341=B_SPLINE_CURVE_WITH_KNOTS('',3,(#43820,#43821,#43822,#43823,#43824,
#43825,#43826,#43827,#43828,#43829,#43830,#43831,#43832,#43833,#43834,#43835),
 .UNSPECIFIED.,.F.,.F.,(4,1,1,1,1,1,1,1,1,1,1,1,1,4),(216.769893097696,
217.561927761979,218.060759370421,218.559590978863,219.058422587305,219.557254195746,
220.056085804188,220.55491741263,221.053749021072,221.552580629514,222.051412237955,
222.550243846397,223.049075454839,223.053078404875),.UNSPECIFIED.);
#342=B_SPLINE_CURVE_WITH_KNOTS('',3,(#43836,#43837,#43838,#43839,#43840,
#43841,#43842,#43843,#43844,#43845,#43846,#43847,#43848,#43849,#43850,#43851,
#43852),.UNSPECIFIED.,.F.,.F.,(4,1,1,1,1,1,1,1,1,1,1,1,1,1,4),(216.769893097696,
216.965488572745,217.46543548103,217.965382389315,218.4653292976,218.965276205885,
219.46522311417,219.965170022455,220.465116930739,220.965063839024,221.465010747309,
221.964957655594,222.464904563879,222.964851472164,223.053078404875),
 .UNSPECIFIED.);
#343=B_SPLINE_CURVE_WITH_KNOTS('',3,(#43857,#43858,#43859,#43860,#43861,
#43862,#43863,#43864,#43865,#43866,#43867,#43868,#43869,#43870,#43871,#43872,
#43873),.UNSPECIFIED.,.F.,.F.,(4,1,1,1,1,1,1,1,1,1,1,1,1,1,4),(210.486707790516,
210.578285243794,211.077116852236,211.575948460678,212.07478006912,212.573611677561,
213.072443286003,213.571274894445,214.070106502887,214.568938111329,215.06776971977,
215.566601328212,216.065432936654,216.564264545096,216.769893097696),
 .UNSPECIFIED.);
#344=B_SPLINE_CURVE_WITH_KNOTS('',3,(#43874,#43875,#43876,#43877,#43878,
#43879,#43880,#43881,#43882,#43883,#43884,#43885,#43886,#43887,#43888,#43889),
 .UNSPECIFIED.,.F.,.F.,(4,1,1,1,1,1,1,1,1,1,1,1,1,4),(210.486707790516,
210.966125673327,211.466072581612,211.966019489897,212.465966398182,212.965913306467,
213.465860214752,213.965807123036,214.465754031321,214.965700939606,215.465647847891,
215.965594756176,216.465541664461,216.769893097696),.UNSPECIFIED.);
#345=B_SPLINE_CURVE_WITH_KNOTS('',3,(#43894,#43895,#43896,#43897,#43898,
#43899,#43900,#43901,#43902,#43903,#43904,#43905,#43906,#43907,#43908),
 .UNSPECIFIED.,.F.,.F.,(4,1,1,1,1,1,1,1,1,1,1,1,4),(204.203522483337,204.592305942493,
205.091137550935,205.589969159376,206.088800767818,206.58763237626,207.086463984702,
207.585295593144,208.084127201585,208.582958810027,209.081790418469,209.580622026911,
210.486707790516),.UNSPECIFIED.);
#346=B_SPLINE_CURVE_WITH_KNOTS('',3,(#43909,#43910,#43911,#43912,#43913,
#43914,#43915,#43916,#43917,#43918,#43919,#43920,#43921,#43922,#43923,#43924,
#43925),.UNSPECIFIED.,.F.,.F.,(4,1,1,1,1,1,1,1,1,1,1,1,1,1,4),(204.203522483337,
204.466815865624,204.966762773909,205.466709682194,205.966656590479,206.466603498764,
206.966550407049,207.466497315333,207.966444223618,208.466391131903,208.966338040188,
209.466284948473,209.966231856758,210.466178765043,210.486707790516),
 .UNSPECIFIED.);
#347=B_SPLINE_CURVE_WITH_KNOTS('',3,(#43930,#43931,#43932,#43933,#43934,
#43935,#43936,#43937,#43938,#43939,#43940,#43941,#43942,#43943,#43944,#43945),
 .UNSPECIFIED.,.F.,.F.,(4,1,1,1,1,1,1,1,1,1,1,1,1,4),(197.920337176157,
198.10749503275,198.606326641191,199.105158249633,199.603989858075,200.102821466517,
200.601653074959,201.1004846834,201.599316291842,202.098147900284,202.596979508726,
203.594642725609,204.093474334051,204.203522483337),.UNSPECIFIED.);
#348=B_SPLINE_CURVE_WITH_KNOTS('',3,(#43946,#43947,#43948,#43949,#43950,
#43951,#43952,#43953,#43954,#43955,#43956,#43957,#43958,#43959,#43960,#43961,
#43962),.UNSPECIFIED.,.F.,.F.,(4,1,1,1,1,1,1,1,1,1,1,1,1,1,4),(197.920337176157,
197.967506057921,198.467452966206,198.967399874491,199.467346782776,199.967293691061,
200.467240599346,200.967187507631,201.467134415915,201.9670813242,202.467028232485,
202.96697514077,203.466922049055,203.96686895734,204.203522483337),
 .UNSPECIFIED.);
#349=B_SPLINE_CURVE_WITH_KNOTS('',3,(#43967,#43968,#43969,#43970,#43971,
#43972,#43973,#43974,#43975,#43976,#43977,#43978,#43979,#43980,#43981),
 .UNSPECIFIED.,.F.,.F.,(4,1,1,1,1,1,1,1,1,1,1,1,4),(191.637151868978,192.121515731448,
192.62034733989,193.119178948332,193.618010556774,194.116842165215,194.615673773657,
195.114505382099,195.613336990541,196.611000207424,197.109831815866,197.608663424308,
197.920337176157),.UNSPECIFIED.);
#350=B_SPLINE_CURVE_WITH_KNOTS('',3,(#43982,#43983,#43984,#43985,#43986,
#43987,#43988,#43989,#43990,#43991,#43992,#43993,#43994,#43995,#43996,#43997),
 .UNSPECIFIED.,.F.,.F.,(4,1,1,1,1,1,1,1,1,1,1,1,1,4),(191.637151868978,
191.968143158503,192.468090066788,192.968036975073,193.467983883358,193.967930791643,
194.467877699928,194.967824608212,195.467771516497,195.967718424782,196.467665333067,
196.967612241352,197.467559149637,197.920337176157),.UNSPECIFIED.);
#351=B_SPLINE_CURVE_WITH_KNOTS('',3,(#44002,#44003,#44004,#44005,#44006,
#44007,#44008,#44009,#44010,#44011,#44012,#44013,#44014,#44015,#44016,#44017),
 .UNSPECIFIED.,.F.,.F.,(4,1,1,1,1,1,1,1,1,1,1,1,1,4),(185.353966561798,
185.636704821705,186.135536430147,186.634368038589,187.13319964703,187.632031255472,
188.130862863914,188.629694472356,189.627357689239,190.126189297681,190.625020906123,
191.123852514565,191.622684123006,191.637151868978),.UNSPECIFIED.);
#352=B_SPLINE_CURVE_WITH_KNOTS('',3,(#44018,#44019,#44020,#44021,#44022,
#44023,#44024,#44025,#44026,#44027,#44028,#44029,#44030,#44031,#44032,#44033,
#44034),.UNSPECIFIED.,.F.,.F.,(4,1,1,1,1,1,1,1,1,1,1,1,1,1,4),(185.353966561798,
185.4688333508,185.968780259085,186.46872716737,186.968674075655,187.46862098394,
187.968567892225,188.468514800509,188.968461708794,189.468408617079,189.968355525364,
190.468302433649,190.968249341934,191.468196250218,191.637151868978),
 .UNSPECIFIED.);
#353=B_SPLINE_CURVE_WITH_KNOTS('',3,(#44039,#44040,#44041,#44042,#44043,
#44044,#44045,#44046,#44047,#44048,#44049,#44050,#44051,#44052,#44053,#44054,
#44055,#44056,#44057,#44058,#44059,#44060,#44061,#44062,#44063),
 .UNSPECIFIED.,.F.,.F.,(4,3,3,3,3,3,3,3,4),(179.070781254618,179.91290911747,
180.755036980322,181.597164843174,182.439292706026,183.281420568878,184.12354843173,
184.965676294582,185.353966561798),.UNSPECIFIED.);
#354=B_SPLINE_CURVE_WITH_KNOTS('',3,(#44064,#44065,#44066,#44067,#44068,
#44069,#44070,#44071,#44072,#44073,#44074,#44075,#44076,#44077,#44078,#44079),
 .UNSPECIFIED.,.F.,.F.,(4,1,1,1,1,1,1,1,1,1,1,1,1,4),(179.070781254618,
179.469470451382,179.969417359667,180.469364267952,180.969311176237,181.469258084522,
181.969204992806,182.469151901091,182.969098809376,183.469045717661,183.968992625946,
184.468939534231,184.968886442515,185.353966561798),.UNSPECIFIED.);
#355=B_SPLINE_CURVE_WITH_KNOTS('',3,(#44084,#44085,#44086,#44087,#44088,
#44089,#44090,#44091,#44092,#44093,#44094,#44095,#44096,#44097,#44098),
 .UNSPECIFIED.,.F.,.F.,(4,1,1,1,1,1,1,1,1,1,1,1,4),(172.787595947439,173.16591461066,
173.664746219102,174.163577827544,174.662409435986,175.660072652869,176.158904261311,
176.657735869753,177.156567478195,177.655399086636,178.154230695078,178.65306230352,
179.070781254618),.UNSPECIFIED.);
#356=B_SPLINE_CURVE_WITH_KNOTS('',3,(#44099,#44100,#44101,#44102,#44103,
#44104,#44105,#44106,#44107,#44108,#44109,#44110,#44111,#44112,#44113,#44114,
#44115),.UNSPECIFIED.,.F.,.F.,(4,1,1,1,1,1,1,1,1,1,1,1,1,1,4),(172.787595947439,
172.970160643679,173.470107551964,173.970054460249,174.470001368534,174.969948276819,
175.469895185103,175.969842093388,176.469789001673,176.969735909958,177.469682818243,
177.969629726528,178.469576634813,178.969523543097,179.070781254618),
 .UNSPECIFIED.);
#357=B_SPLINE_CURVE_WITH_KNOTS('',3,(#44120,#44121,#44122,#44123,#44124,
#44125,#44126,#44127,#44128,#44129,#44130,#44131,#44132,#44133,#44134,#44135),
 .UNSPECIFIED.,.F.,.F.,(4,1,1,1,1,1,1,1,1,1,1,1,1,4),(166.504410640259,
166.681103700917,167.179935309359,167.678766917801,168.676430134684,169.175261743126,
169.674093351568,170.17292496001,170.671756568452,171.170588176893,171.669419785335,
172.168251393777,172.667083002219,172.787595947439),.UNSPECIFIED.);
#358=B_SPLINE_CURVE_WITH_KNOTS('',3,(#44136,#44137,#44138,#44139,#44140,
#44141,#44142,#44143,#44144,#44145,#44146,#44147,#44148,#44149,#44150,#44151),
 .UNSPECIFIED.,.F.,.F.,(4,1,1,1,1,1,1,1,1,1,1,1,1,4),(166.504410640259,
166.970797744261,167.470744652546,167.970691560831,168.470638469116,168.970585377401,
169.470532285685,169.97047919397,170.470426102255,170.97037301054,171.470319918825,
171.97026682711,172.470213735394,172.787595947439),.UNSPECIFIED.);
#359=B_SPLINE_CURVE_WITH_KNOTS('',3,(#44156,#44157,#44158,#44159,#44160,
#44161,#44162,#44163,#44164,#44165,#44166,#44167,#44168,#44169,#44170),
 .UNSPECIFIED.,.F.,.F.,(4,1,1,1,1,1,1,1,1,1,1,1,4),(160.22122533308,160.695124399616,
161.692787616499,162.191619224941,162.690450833383,163.189282441825,163.688114050267,
164.186945658708,164.68577726715,165.184608875592,165.683440484034,166.182272092475,
166.504410640259),.UNSPECIFIED.);
#360=B_SPLINE_CURVE_WITH_KNOTS('',3,(#44171,#44172,#44173,#44174,#44175,
#44176,#44177,#44178,#44179,#44180,#44181,#44182,#44183,#44184,#44185,#44186,
#44187),.UNSPECIFIED.,.F.,.F.,(4,1,1,1,1,1,1,1,1,1,1,1,1,1,4),(160.22122533308,
160.471487936558,160.971434844843,161.471381753128,161.971328661413,162.471275569698,
162.971222477982,163.471169386267,163.971116294552,164.471063202837,164.971010111122,
165.470957019407,165.970903927691,166.470850835976,166.504410640259),
 .UNSPECIFIED.);
#361=B_SPLINE_CURVE_WITH_KNOTS('',3,(#44192,#44193,#44194,#44195,#44196,
#44197,#44198,#44199,#44200,#44201,#44202,#44203,#44204,#44205,#44206,#44207),
 .UNSPECIFIED.,.F.,.F.,(4,1,1,1,1,1,1,1,1,1,1,1,1,4),(153.9380400259,154.709145098314,
155.207976706756,155.706808315198,156.20563992364,156.704471532082,157.203303140523,
157.702134748965,158.200966357407,158.699797965849,159.19862957429,159.697461182732,
160.196292791174,160.22122533308),.UNSPECIFIED.);
#362=B_SPLINE_CURVE_WITH_KNOTS('',3,(#44208,#44209,#44210,#44211,#44212,
#44213,#44214,#44215,#44216,#44217,#44218,#44219,#44220,#44221,#44222,#44223,
#44224),.UNSPECIFIED.,.F.,.F.,(4,1,1,1,1,1,1,1,1,1,1,1,1,1,4),(153.9380400259,
153.972178128855,154.47212503714,154.972071945425,155.47201885371,155.971965761995,
156.471912670279,156.971859578564,157.471806486849,157.971753395134,158.471700303419,
158.971647211704,159.471594119988,159.971541028273,160.22122533308),
 .UNSPECIFIED.);
#363=B_SPLINE_CURVE_WITH_KNOTS('',3,(#44229,#44230,#44231,#44232,#44233,
#44234,#44235,#44236,#44237,#44238,#44239,#44240,#44241,#44242,#44243,#44244,
#44245),.UNSPECIFIED.,.F.,.F.,(4,1,1,1,1,1,1,1,1,1,1,1,1,1,4),(147.654854718721,
147.725502580129,148.224334188571,148.723165797013,149.221997405455,149.720829013897,
150.219660622338,150.71849223078,151.217323839222,151.716155447664,152.214987056105,
152.713818664547,153.212650272989,153.711481881431,153.9380400259),
 .UNSPECIFIED.);
#364=B_SPLINE_CURVE_WITH_KNOTS('',3,(#44246,#44247,#44248,#44249,#44250,
#44251,#44252,#44253,#44254,#44255,#44256,#44257,#44258,#44259,#44260,#44261),
 .UNSPECIFIED.,.F.,.F.,(4,1,1,1,1,1,1,1,1,1,1,1,1,4),(147.654854718721,
147.972815229437,148.472762137722,148.972709046007,149.472655954292,149.972602862576,
150.472549770861,150.972496679146,151.472443587431,151.972390495716,152.472337404001,
152.972284312286,153.47223122057,153.9380400259),.UNSPECIFIED.);
#365=B_SPLINE_CURVE_WITH_KNOTS('',3,(#44266,#44267,#44268,#44269,#44270,
#44271,#44272,#44273,#44274,#44275,#44276,#44277,#44278,#44279),
 .UNSPECIFIED.,.F.,.F.,(4,1,1,1,1,1,1,1,1,1,1,4),(141.371669411541,141.739523278828,
142.737186495712,143.236018104153,143.734849712595,144.233681321037,144.732512929479,
145.231344537921,145.730176146362,146.229007754804,146.727839363246,147.654854718721),
 .UNSPECIFIED.);
#366=B_SPLINE_CURVE_WITH_KNOTS('',3,(#44280,#44281,#44282,#44283,#44284,
#44285,#44286,#44287,#44288,#44289,#44290,#44291,#44292,#44293,#44294,#44295,
#44296),.UNSPECIFIED.,.F.,.F.,(4,1,1,1,1,1,1,1,1,1,1,1,1,1,4),(141.371669411541,
141.473505421734,141.973452330019,142.473399238304,142.973346146589,143.473293054873,
143.973239963158,144.473186871443,144.973133779728,145.473080688013,145.973027596298,
146.472974504583,146.972921412867,147.472868321152,147.654854718721),
 .UNSPECIFIED.);
#367=B_SPLINE_CURVE_WITH_KNOTS('',3,(#44301,#44302,#44303,#44304,#44305,
#44306,#44307,#44308,#44309,#44310,#44311,#44312,#44313,#44314,#44315,#44316),
 .UNSPECIFIED.,.F.,.F.,(4,1,1,1,1,1,1,1,1,1,1,1,1,4),(135.088484104361,
135.753543977527,136.252375585968,136.75120719441,137.250038802852,137.748870411294,
138.247702019735,138.746533628177,139.245365236619,139.744196845061,140.243028453503,
140.741860061944,141.240691670386,141.371669411541),.UNSPECIFIED.);
#368=B_SPLINE_CURVE_WITH_KNOTS('',3,(#44317,#44318,#44319,#44320,#44321,
#44322,#44323,#44324,#44325,#44326,#44327,#44328,#44329,#44330),
 .UNSPECIFIED.,.F.,.F.,(4,1,1,1,1,1,1,1,1,1,1,4),(135.088484104361,135.474142522316,
135.974089430601,136.474036338886,136.973983247171,137.473930155455,137.97387706374,
138.473823972025,138.97377088031,139.97366469688,140.973558513449,141.371669411541),
 .UNSPECIFIED.);
#369=B_SPLINE_CURVE_WITH_KNOTS('',3,(#44335,#44336,#44337,#44338,#44339,
#44340,#44341,#44342,#44343,#44344,#44345,#44346,#44347,#44348,#44349,#44350),
 .UNSPECIFIED.,.F.,.F.,(4,1,1,1,1,1,1,1,1,1,1,1,1,4),(128.805298797182,
129.268733067783,129.767564676225,130.266396284667,130.765227893109,131.26405950155,
131.762891109992,132.261722718434,132.760554326876,133.259385935318,133.758217543759,
134.257049152201,134.755880760643,135.088484104361),.UNSPECIFIED.);
#370=B_SPLINE_CURVE_WITH_KNOTS('',3,(#44351,#44352,#44353,#44354,#44355,
#44356,#44357,#44358,#44359,#44360,#44361,#44362,#44363,#44364,#44365,#44366,
#44367),.UNSPECIFIED.,.F.,.F.,(4,1,1,1,1,1,1,1,1,1,1,1,1,1,4),(128.805298797182,
128.974832714613,129.474779622898,129.974726531183,130.474673439468,130.974620347752,
131.474567256037,131.974514164322,132.474461072607,132.974407980892,133.474354889177,
133.974301797461,134.474248705746,134.974195614031,135.088484104361),
 .UNSPECIFIED.);
#371=B_SPLINE_CURVE_WITH_KNOTS('',3,(#44372,#44373,#44374,#44375,#44376,
#44377,#44378,#44379,#44380,#44381,#44382,#44383,#44384,#44385,#44386,#44387),
 .UNSPECIFIED.,.F.,.F.,(4,1,1,1,1,1,1,1,1,1,1,1,1,4),(122.522113490002,
122.78392215804,123.282753766482,123.781585374924,124.280416983366,124.779248591807,
125.278080200249,125.776911808691,126.275743417133,126.774575025574,127.273406634016,
127.772238242458,128.769901459342,128.805298797182),.UNSPECIFIED.);
#372=B_SPLINE_CURVE_WITH_KNOTS('',3,(#44388,#44389,#44390,#44391,#44392,
#44393,#44394,#44395,#44396,#44397,#44398,#44399,#44400,#44401,#44402,#44403),
 .UNSPECIFIED.,.F.,.F.,(4,1,1,1,1,1,1,1,1,1,1,1,1,4),(122.522113490002,
122.975469815195,123.47541672348,123.975363631765,124.475310540049,124.975257448334,
125.475204356619,125.975151264904,126.475098173189,126.975045081474,127.474991989759,
127.974938898043,128.474885806328,128.805298797182),.UNSPECIFIED.);
#373=B_SPLINE_CURVE_WITH_KNOTS('',3,(#44408,#44409,#44410,#44411,#44412,
#44413,#44414,#44415,#44416,#44417,#44418,#44419,#44420,#44421,#44422,#44423),
 .UNSPECIFIED.,.F.,.F.,(4,1,1,1,1,1,1,1,1,1,1,1,1,4),(116.238928182823,
116.299111248297,116.797942856739,117.296774465181,117.795606073622,118.294437682064,
118.793269290506,119.292100898948,119.790932507389,120.289764115831,120.788595724273,
121.786258941157,122.285090549598,122.522113490002),.UNSPECIFIED.);
#374=B_SPLINE_CURVE_WITH_KNOTS('',3,(#44424,#44425,#44426,#44427,#44428,
#44429,#44430,#44431,#44432,#44433,#44434,#44435,#44436,#44437,#44438,#44439,
#44440),.UNSPECIFIED.,.F.,.F.,(4,1,1,1,1,1,1,1,1,1,1,1,1,1,4),(116.238928182823,
116.476160007492,116.976106915777,117.476053824062,117.976000732346,118.475947640631,
118.975894548916,119.475841457201,119.975788365486,120.475735273771,120.975682182056,
121.47562909034,121.975575998625,122.47552290691,122.522113490002),
 .UNSPECIFIED.);
#375=B_SPLINE_CURVE_WITH_KNOTS('',3,(#44445,#44446,#44447,#44448,#44449,
#44450,#44451,#44452,#44453,#44454,#44455,#44456,#44457,#44458,#44459),
 .UNSPECIFIED.,.F.,.F.,(4,1,1,1,1,1,1,1,1,1,1,1,4),(109.955742875643,110.313131946996,
110.811963555437,111.310795163879,111.809626772321,112.308458380763,112.807289989204,
113.306121597646,113.804953206088,114.802616422972,115.301448031413,115.800279639855,
116.238928182823),.UNSPECIFIED.);
#376=B_SPLINE_CURVE_WITH_KNOTS('',3,(#44460,#44461,#44462,#44463,#44464,
#44465,#44466,#44467,#44468,#44469,#44470,#44471,#44472,#44473,#44474,#44475,
#44476),.UNSPECIFIED.,.F.,.F.,(4,1,1,1,1,1,1,1,1,1,1,1,1,1,4),(109.955742875643,
109.976850199789,110.476797108074,110.976744016359,111.476690924644,111.976637832928,
112.476584741213,112.976531649498,113.476478557783,113.976425466068,114.476372374353,
114.976319282637,115.476266190922,115.976213099207,116.238928182823),
 .UNSPECIFIED.);
#377=B_SPLINE_CURVE_WITH_KNOTS('',3,(#44481,#44482,#44483,#44484,#44485,
#44486,#44487,#44488,#44489,#44490,#44491,#44492,#44493,#44494,#44495,#44496),
 .UNSPECIFIED.,.F.,.F.,(4,1,1,1,1,1,1,1,1,1,1,1,1,4),(103.672557568464,
103.828321037252,104.327152645694,104.825984254136,105.324815862578,105.823647471019,
106.322479079461,106.821310687903,107.818973904787,108.317805513228,108.81663712167,
109.315468730112,109.814300338554,109.955742875643),.UNSPECIFIED.);
#378=B_SPLINE_CURVE_WITH_KNOTS('',3,(#44497,#44498,#44499,#44500,#44501,
#44502,#44503,#44504,#44505,#44506,#44507,#44508,#44509,#44510,#44511,#44512),
 .UNSPECIFIED.,.F.,.F.,(4,1,1,1,1,1,1,1,1,1,1,1,1,4),(103.672557568464,
103.977487300371,104.477434208656,104.977381116941,105.477328025225,105.97727493351,
106.477221841795,106.97716875008,107.477115658365,107.97706256665,108.477009474934,
108.976956383219,109.476903291504,109.955742875643),.UNSPECIFIED.);
#379=B_SPLINE_CURVE_WITH_KNOTS('',3,(#44517,#44518,#44519,#44520,#44521,
#44522,#44523,#44524,#44525,#44526,#44527,#44528,#44529,#44530,#44531),
 .UNSPECIFIED.,.F.,.F.,(4,1,1,1,1,1,1,1,1,1,1,1,4),(97.3893722612839,97.8423417359509,
98.3411733443927,98.8400049528345,99.3388365612763,99.8376681697181,100.835331386602,
101.334162995043,101.832994603485,102.331826211927,102.830657820369,103.329489428811,
103.672557568464),.UNSPECIFIED.);
#380=B_SPLINE_CURVE_WITH_KNOTS('',3,(#44532,#44533,#44534,#44535,#44536,
#44537,#44538,#44539,#44540,#44541,#44542,#44543,#44544,#44545,#44546,#44547,
#44548),.UNSPECIFIED.,.F.,.F.,(4,1,1,1,1,1,1,1,1,1,1,1,1,1,4),(97.389372261284,
97.4781774926679,97.9781244009527,98.4780713092376,98.9780182175224,99.4779651258073,
99.9779120340921,100.477858942377,100.977805850662,101.477752758947,101.977699667231,
102.477646575516,102.977593483801,103.477540392086,103.672557568464),
 .UNSPECIFIED.);
#381=B_SPLINE_CURVE_WITH_KNOTS('',3,(#44553,#44554,#44555,#44556,#44557,
#44558,#44559,#44560,#44561,#44562,#44563,#44564,#44565,#44566,#44567,#44568),
 .UNSPECIFIED.,.F.,.F.,(4,1,1,1,1,1,1,1,1,1,1,1,1,4),(91.1061869541043,
91.3575308262077,91.8563624346495,92.3551940430913,92.8540256515331,93.8516888684167,
94.3505204768584,94.8493520853002,95.348183693742,95.8470153021838,96.3458469106256,
96.8446785190674,97.3435101275091,97.3893722612839),.UNSPECIFIED.);
#382=B_SPLINE_CURVE_WITH_KNOTS('',3,(#44569,#44570,#44571,#44572,#44573,
#44574,#44575,#44576,#44577,#44578,#44579,#44580,#44581,#44582,#44583,#44584),
 .UNSPECIFIED.,.F.,.F.,(4,1,1,1,1,1,1,1,1,1,1,1,1,4),(91.1061869541044,
91.4788145932498,91.9787615015346,92.4787084098195,92.9786553181043,93.4786022263891,
93.978549134674,94.4784960429588,94.9784429512437,95.4783898595285,95.9783367678134,
96.4782836760982,96.9782305843831,97.389372261284),.UNSPECIFIED.);
#383=B_SPLINE_CURVE_WITH_KNOTS('',3,(#44589,#44590,#44591,#44592,#44593,
#44594,#44595,#44596,#44597,#44598,#44599,#44600,#44601,#44602,#44603,#44604),
 .UNSPECIFIED.,.F.,.F.,(4,1,1,1,1,1,1,1,1,1,1,1,1,4),(84.8230016469247,
84.8727199164645,85.3715515249063,85.8703831333481,86.8680463502317,87.3668779586735,
87.8657095671152,88.364541175557,88.8633727839988,89.3622043924406,89.8610360008824,
90.3598676093242,90.8586992177659,91.1061869541043),.UNSPECIFIED.);
#384=B_SPLINE_CURVE_WITH_KNOTS('',3,(#44605,#44606,#44607,#44608,#44609,
#44610,#44611,#44612,#44613,#44614,#44615,#44616,#44617,#44618,#44619,#44620,
#44621),.UNSPECIFIED.,.F.,.F.,(4,1,1,1,1,1,1,1,1,1,1,1,1,1,4),(84.8230016469248,
84.9795047855468,85.4794516938317,85.9793986021165,86.4793455104013,86.9792924186862,
87.479239326971,87.9791862352559,88.4791331435407,88.9790800518255,89.4790269601104,
89.9789738683953,90.4789207766801,90.9788676849649,91.1061869541044),
 .UNSPECIFIED.);
#385=B_SPLINE_CURVE_WITH_KNOTS('',3,(#44626,#44627,#44628,#44629,#44630,
#44631,#44632,#44633,#44634,#44635,#44636,#44637,#44638,#44639,#44640),
 .UNSPECIFIED.,.F.,.F.,(4,1,1,1,1,1,1,1,1,1,1,1,4),(78.5398163397451,78.8867406151631,
79.8844038320467,80.3832354404885,80.8820670489303,81.380898657372,81.8797302658138,
82.3785618742556,82.8773934826974,83.3762250911392,83.875056699581,84.3738883080227,
84.8230016469247),.UNSPECIFIED.);
#386=B_SPLINE_CURVE_WITH_KNOTS('',3,(#44641,#44642,#44643,#44644,#44645,
#44646,#44647,#44648,#44649,#44650,#44651,#44652,#44653,#44654,#44655,#44656),
 .UNSPECIFIED.,.F.,.F.,(4,1,1,1,1,1,1,1,1,1,1,1,1,4),(78.5398163397452,
78.9801418861287,79.4800887944135,79.9800357026984,80.4799826109832,80.9799295192681,
81.4798764275529,81.9798233358378,82.4797702441226,82.9797171524074,83.4796640606923,
83.9796109689771,84.479557877262,84.8230016469248),.UNSPECIFIED.);
#387=B_SPLINE_CURVE_WITH_KNOTS('',3,(#44661,#44662,#44663,#44664,#44665,
#44666,#44667,#44668,#44669,#44670,#44671,#44672,#44673,#44674,#44675,#44676),
 .UNSPECIFIED.,.F.,.F.,(4,1,1,1,1,1,1,1,1,1,1,1,1,4),(72.2566310325655,
72.9007613138617,73.3995929223035,73.8984245307453,74.397256139187,74.8960877476288,
75.3949193560706,75.8937509645124,76.3925825729542,76.891414181396,77.3902457898378,
77.8890773982795,78.3879090067213,78.5398163397451),.UNSPECIFIED.);
#388=B_SPLINE_CURVE_WITH_KNOTS('',3,(#44677,#44678,#44679,#44680,#44681,
#44682,#44683,#44684,#44685,#44686,#44687,#44688,#44689,#44690,#44691,#44692,
#44693),.UNSPECIFIED.,.F.,.F.,(4,1,1,1,1,1,1,1,1,1,1,1,1,1,4),(72.2566310325657,
72.4808320784257,72.9807789867106,73.4807258949954,73.9806728032802,74.4806197115651,
74.98056661985,75.4805135281348,75.9804604364196,76.4804073447045,76.9803542529893,
77.4803011612742,77.980248069559,78.4801949778438,78.5398163397452),
 .UNSPECIFIED.);
#389=B_SPLINE_CURVE_WITH_KNOTS('',3,(#44698,#44699,#44700,#44701,#44702,
#44703,#44704,#44705,#44706,#44707,#44708,#44709,#44710,#44711,#44712,#44713),
 .UNSPECIFIED.,.F.,.F.,(4,1,1,1,1,1,1,1,1,1,1,1,1,4),(65.9734457253859,
66.4159504041185,66.9147820125603,67.4136136210021,67.9124452294438,68.4112768378856,
68.9101084463274,69.4089400547692,69.907771663211,70.4066032716528,70.9054348800946,
71.4042664885363,71.9030980969781,72.2566310325655),.UNSPECIFIED.);
#390=B_SPLINE_CURVE_WITH_KNOTS('',3,(#44714,#44715,#44716,#44717,#44718,
#44719,#44720,#44721,#44722,#44723,#44724,#44725,#44726,#44727,#44728,#44729,
#44730),.UNSPECIFIED.,.F.,.F.,(4,1,1,1,1,1,1,1,1,1,1,1,1,1,4),(65.973445725386,
65.9815222707228,66.4814691790076,66.9814160872924,67.4813629955773,67.9813099038621,
68.481256812147,68.9812037204318,69.4811506287167,69.9810975370015,70.4810444452864,
70.9809913535712,71.480938261856,71.9808851701409,72.2566310325657),
 .UNSPECIFIED.);
#391=B_SPLINE_CURVE_WITH_KNOTS('',3,(#44735,#44736,#44737,#44738,#44739,
#44740,#44741,#44742,#44743,#44744,#44745,#44746,#44747,#44748,#44749,#44750),
 .UNSPECIFIED.,.F.,.F.,(4,1,1,1,1,1,1,1,1,1,1,1,1,4),(59.6902604182064,
59.9311394943753,60.4299711028171,60.9288027112589,61.4276343197006,61.9264659281424,
62.4252975365842,62.924129145026,63.4229607534678,63.9217923619096,64.4206239703514,
64.9194555787931,65.9171187956767,65.9734457253859),.UNSPECIFIED.);
#392=B_SPLINE_CURVE_WITH_KNOTS('',3,(#44751,#44752,#44753,#44754,#44755,
#44756,#44757,#44758,#44759,#44760,#44761,#44762,#44763,#44764,#44765,#44766),
 .UNSPECIFIED.,.F.,.F.,(4,1,1,1,1,1,1,1,1,1,1,1,1,4),(59.6902604182065,
59.9821593713046,60.4821062795895,60.9820531878743,61.4820000961592,61.981947004444,
62.4818939127289,62.9818408210137,63.4817877292985,63.9817346375834,64.4816815458682,
64.9816284541531,65.4815753624379,65.973445725386),.UNSPECIFIED.);
#393=B_SPLINE_CURVE_WITH_KNOTS('',3,(#44771,#44772,#44773,#44774,#44775,
#44776,#44777,#44778,#44779,#44780,#44781,#44782,#44783,#44784,#44785,#44786),
 .UNSPECIFIED.,.F.,.F.,(4,1,1,1,1,1,1,1,1,1,1,1,1,4),(53.4070751110267,
53.4463285846321,53.9451601930739,54.4439918015157,54.9428234099574,55.4416550183992,
55.940486626841,56.4393182352828,56.9381498437246,57.4369814521664,57.9358130606082,
58.9334762774917,59.4323078859335,59.6902604182064),.UNSPECIFIED.);
#394=B_SPLINE_CURVE_WITH_KNOTS('',3,(#44787,#44788,#44789,#44790,#44791,
#44792,#44793,#44794,#44795,#44796,#44797,#44798,#44799,#44800,#44801,#44802,
#44803),.UNSPECIFIED.,.F.,.F.,(4,1,1,1,1,1,1,1,1,1,1,1,1,1,4),(53.4070751110269,
53.4828495636017,53.9827964718865,54.4827433801714,54.9826902884562,55.4826371967411,
55.9825841050259,56.4825310133107,56.9824779215956,57.4824248298804,57.9823717381653,
58.4823186464501,58.982265554735,59.4822124630198,59.6902604182065),
 .UNSPECIFIED.);
#395=B_SPLINE_CURVE_WITH_KNOTS('',3,(#44808,#44809,#44810,#44811,#44812,
#44813,#44814,#44815,#44816,#44817,#44818,#44819,#44820,#44821,#44822),
 .UNSPECIFIED.,.F.,.F.,(4,1,1,1,1,1,1,1,1,1,1,1,4),(47.1238898038472,47.4603492833307,
47.9591808917725,48.4580125002142,48.956844108656,49.4556757170978,49.9545073255396,
50.4533389339814,50.9521705424232,51.9498337593067,52.4486653677485,52.9474969761903,
53.4070751110267),.UNSPECIFIED.);
#396=B_SPLINE_CURVE_WITH_KNOTS('',3,(#44823,#44824,#44825,#44826,#44827,
#44828,#44829,#44830,#44831,#44832,#44833,#44834,#44835,#44836,#44837,#44838),
 .UNSPECIFIED.,.F.,.F.,(4,1,1,1,1,1,1,1,1,1,1,1,1,4),(47.1238898038473,
47.4834866641836,47.9834335724684,48.4833804807532,48.9833273890381,49.4832742973229,
49.9832212056078,50.4831681138926,50.9831150221775,51.4830619304623,51.9830088387471,
52.482955747032,52.9829026553168,53.4070751110269),.UNSPECIFIED.);
#397=B_SPLINE_CURVE_WITH_KNOTS('',3,(#44843,#44844,#44845,#44846,#44847,
#44848,#44849,#44850,#44851,#44852,#44853,#44854,#44855,#44856,#44857,#44858),
 .UNSPECIFIED.,.F.,.F.,(4,1,1,1,1,1,1,1,1,1,1,1,1,4),(40.8407044966676,
40.9755383735875,41.4743699820293,41.973201590471,42.4720331989128,42.9708648073546,
43.4696964157964,43.9685280242382,44.9661912411217,45.4650228495635,45.9638544580053,
46.4626860664471,46.9615176748889,47.1238898038472),.UNSPECIFIED.);
#398=B_SPLINE_CURVE_WITH_KNOTS('',3,(#44859,#44860,#44861,#44862,#44863,
#44864,#44865,#44866,#44867,#44868,#44869,#44870,#44871,#44872,#44873,#44874,
#44875),.UNSPECIFIED.,.F.,.F.,(4,1,1,1,1,1,1,1,1,1,1,1,1,1,4),(40.8407044966677,
40.9841768564806,41.4841237647654,41.9840706730503,42.4840175813351,42.98396448962,
43.4839113979048,43.9838583061896,44.4838052144745,44.9837521227593,45.4836990310442,
45.983645939329,46.4835928476139,46.9835397558987,47.1238898038473),
 .UNSPECIFIED.);
#399=B_SPLINE_CURVE_WITH_KNOTS('',3,(#44880,#44881,#44882,#44883,#44884,
#44885,#44886,#44887,#44888,#44889,#44890,#44891,#44892,#44893,#44894),
 .UNSPECIFIED.,.F.,.F.,(4,1,1,1,1,1,1,1,1,1,1,1,4),(34.557519189488,34.9895590722861,
35.4883906807278,35.9872222891696,36.4860538976114,36.9848855060532,37.9825487229368,
38.4813803313785,38.9802119398203,39.4790435482621,39.9778751567039,40.4767067651457,
40.8407044966676),.UNSPECIFIED.);
#400=B_SPLINE_CURVE_WITH_KNOTS('',3,(#44895,#44896,#44897,#44898,#44899,
#44900,#44901,#44902,#44903,#44904,#44905,#44906,#44907,#44908,#44909,#44910),
 .UNSPECIFIED.,.F.,.F.,(4,1,1,1,1,1,1,1,1,1,1,1,1,4),(34.5575191894881,
34.9848139570625,35.4847608653473,35.9847077736322,36.484654681917,36.9846015902018,
37.4845484984867,37.9844954067715,38.4844423150564,38.9843892233412,39.4843361316261,
39.9842830399109,40.4842299481957,40.8407044966677),.UNSPECIFIED.);
#401=B_SPLINE_CURVE_WITH_KNOTS('',3,(#44915,#44916,#44917,#44918,#44919,
#44920,#44921,#44922,#44923,#44924,#44925,#44926,#44927,#44928,#44929,#44930),
 .UNSPECIFIED.,.F.,.F.,(4,1,1,1,1,1,1,1,1,1,1,1,1,4),(28.2743338823084,
28.5047481625429,29.0035797709846,29.5024113794264,30.0012429878682,30.9989062047518,
31.4977378131936,31.9965694216353,32.4954010300771,32.9942326385189,33.4930642469607,
33.9918958554025,34.4907274638443,34.557519189488),.UNSPECIFIED.);
#402=B_SPLINE_CURVE_WITH_KNOTS('',3,(#44931,#44932,#44933,#44934,#44935,
#44936,#44937,#44938,#44939,#44940,#44941,#44942,#44943,#44944,#44945,#44946,
#44947),.UNSPECIFIED.,.F.,.F.,(4,1,1,1,1,1,1,1,1,1,1,1,1,1,4),(28.2743338823085,
28.4855041493595,28.9854510576443,29.4853979659292,29.985344874214,30.4852917824989,
30.9852386907837,31.4851855990686,31.9851325073534,32.4850794156383,32.9850263239231,
33.4849732322079,33.9849201404928,34.4848670487776,34.5575191894881),
 .UNSPECIFIED.);
#403=B_SPLINE_CURVE_WITH_KNOTS('',3,(#44952,#44953,#44954,#44955,#44956,
#44957,#44958,#44959,#44960,#44961,#44962,#44963,#44964,#44965,#44966,#44967),
 .UNSPECIFIED.,.F.,.F.,(4,1,1,1,1,1,1,1,1,1,1,1,1,4),(21.9911485751288,
22.0199372527997,22.5187688612414,23.0176004696832,24.0152636865668,24.5140952950086,
25.0129269034504,25.5117585118921,26.0105901203339,26.5094217287757,27.0082533372175,
27.5070849456593,28.0059165541011,28.2743338823084),.UNSPECIFIED.);
#404=B_SPLINE_CURVE_WITH_KNOTS('',3,(#44968,#44969,#44970,#44971,#44972,
#44973,#44974,#44975,#44976,#44977,#44978,#44979,#44980,#44981,#44982,#44983),
 .UNSPECIFIED.,.F.,.F.,(4,1,1,1,1,1,1,1,1,1,1,1,1,4),(21.9911485751289,
22.4861412499414,22.9860881582262,23.4860350665111,23.9859819747959,24.4859288830808,
24.9858757913656,25.4858226996504,25.9857696079353,26.4857165162201,26.985663424505,
27.4856103327898,27.9855572410747,28.2743338823085),.UNSPECIFIED.);
#405=B_SPLINE_CURVE_WITH_KNOTS('',3,(#44988,#44989,#44990,#44991,#44992,
#44993,#44994,#44995,#44996,#44997,#44998,#44999,#45000,#45001,#45002),
 .UNSPECIFIED.,.F.,.F.,(4,1,1,1,1,1,1,1,1,1,1,1,4),(15.7079632679492,16.0339579514982,
17.0316211683818,17.5304527768236,18.0292843852654,18.5281159937072,19.0269476021489,
19.5257792105907,20.0246108190325,20.5234424274743,21.0222740359161,21.5211056443579,
21.9911485751288),.UNSPECIFIED.);
#406=B_SPLINE_CURVE_WITH_KNOTS('',3,(#45003,#45004,#45005,#45006,#45007,
#45008,#45009,#45010,#45011,#45012,#45013,#45014,#45015,#45016,#45017,#45018,
#45019),.UNSPECIFIED.,.F.,.F.,(4,1,1,1,1,1,1,1,1,1,1,1,1,1,4),(15.7079632679493,
15.9868314422384,16.4867783505233,16.9867252588081,17.4866721670929,17.9866190753778,
18.4865659836626,18.9865128919475,19.4864598002323,19.9864067085172,20.486353616802,
20.9863005250869,21.4862474333717,21.9861943416565,21.9911485751289),
 .UNSPECIFIED.);
#407=B_SPLINE_CURVE_WITH_KNOTS('',3,(#45052,#45053,#45054,#45055,#45056,
#45057,#45058,#45059,#45060,#45061,#45062,#45063,#45064,#45065,#45066,#45067,
#45068,#45069,#45070,#45071,#45072,#45073,#45074,#45075,#45076,#45077,#45078,
#45079,#45080,#45081,#45082,#45083,#45084,#45085,#45086,#45087,#45088,#45089,
#45090,#45091,#45092,#45093,#45094,#45095,#45096,#45097,#45098,#45099,#45100,
#45101,#45102,#45103,#45104,#45105,#45106,#45107,#45108,#45109,#45110,#45111,
#45112),.UNSPECIFIED.,.F.,.F.,(4,3,3,3,3,3,3,3,3,3,3,3,3,3,3,3,3,3,3,3,
4),(-1.70371038777376,-1.57164896760842,-1.45968081939285,-1.42104956412851,
-1.38937747141726,-1.25766313377658,-1.18516797863899,-1.14888374991031,
-1.11514150461779,-0.984197499563139,-0.967682513226223,-0.845964405260809,
-0.78525894660507,-0.754188806238284,-0.728523041048962,-0.598532726708555,
-0.480810081364569,-0.419431608816291,-0.381410915251877,-0.356693156275484,
-0.245712839762795),.UNSPECIFIED.);
#408=B_SPLINE_CURVE_WITH_KNOTS('',3,(#45114,#45115,#45116,#45117,#45118,
#45119,#45120,#45121,#45122,#45123,#45124,#45125,#45126,#45127,#45128,#45129,
#45130,#45131,#45132,#45133,#45134,#45135,#45136,#45137,#45138,#45139,#45140,
#45141,#45142,#45143,#45144,#45145,#45146,#45147,#45148,#45149,#45150,#45151,
#45152,#45153,#45154,#45155,#45156,#45157,#45158,#45159,#45160,#45161,#45162),
 .UNSPECIFIED.,.F.,.F.,(4,3,3,3,3,3,3,3,3,3,3,3,3,3,3,3,4),(-1.16887606902948,
-1.04801251096666,-0.994206397697257,-0.946140023287794,-0.815780930032988,
-0.781046175157294,-0.751089839681922,-0.685421836778182,-0.554489283265102,
-0.46425321950904,-0.415674365158631,-0.389975975593583,-0.362776987536873,
-0.230336045464461,-0.193545028240855,-0.0612057741671412,-5.34073745228555E-5),
 .UNSPECIFIED.);
#409=B_SPLINE_CURVE_WITH_KNOTS('',3,(#47153,#47154,#47155,#47156,#47157,
#47158,#47159,#47160,#47161,#47162,#47163,#47164,#47165,#47166,#47167,#47168,
#47169,#47170,#47171,#47172,#47173,#47174),.UNSPECIFIED.,.F.,.F.,(4,3,3,
3,3,3,3,4),(-1.73957725076382,-1.61100415945136,-1.52396281589798,-1.48243222042214,
-1.45665092794175,-1.32808793138577,-1.26283878523785,-1.15068998546189),
 .UNSPECIFIED.);
#410=B_SPLINE_CURVE_WITH_KNOTS('',3,(#47175,#47176,#47177,#47178,#47179,
#47180,#47181,#47182,#47183,#47184,#47185,#47186,#47187,#47188,#47189,#47190,
#47191,#47192,#47193,#47194,#47195,#47196,#47197,#47198,#47199,#47200,#47201,
#47202,#47203,#47204,#47205,#47206,#47207,#47208),.UNSPECIFIED.,.F.,.F.,
(4,3,3,3,3,3,3,3,3,3,3,4),(-0.878140325105598,-0.777511794155485,-0.671462782584743,
-0.631586372873439,-0.604605941415006,-0.565413771014002,-0.456171084017733,
-0.390222098706532,-0.365207136260434,-0.340281065404979,-0.223557747407252,
-0.210417151407702),.UNSPECIFIED.);
#411=B_SPLINE_CURVE_WITH_KNOTS('',3,(#47210,#47211,#47212,#47213,#47214,
#47215,#47216,#47217,#47218,#47219,#47220),.UNSPECIFIED.,.F.,.F.,(4,1,1,
1,1,1,1,1,4),(12.043305083964,12.5421366924057,13.0409683008475,13.5397999092893,
14.0386315177311,14.5374631261729,15.0362947346147,15.5351263430564,15.7079632679492),
 .UNSPECIFIED.);
#412=B_SPLINE_CURVE_WITH_KNOTS('',3,(#47221,#47222,#47223,#47224,#47225,
#47226,#47227,#47228,#47229,#47230,#47231,#47232,#47233,#47234,#47235,#47236,
#47237,#47238,#47239,#47240,#47241,#47242,#47243,#47244,#47245,#47246,#47247,
#47248,#47249,#47250,#47251,#47252,#47253,#47254),.UNSPECIFIED.,.F.,.F.,
(4,3,3,3,3,3,3,3,3,3,3,4),(-0.873477877141213,-0.753141137816717,-0.635235160226647,
-0.592041969943734,-0.557997950910165,-0.446311798303827,-0.427982605240538,
-0.320986953930404,-0.284657590233497,-0.180950825577172,-0.0805654152611678,
0.),.UNSPECIFIED.);
#413=B_SPLINE_CURVE_WITH_KNOTS('',3,(#47255,#47256,#47257,#47258,#47259,
#47260,#47261,#47262,#47263,#47264,#47265,#47266,#47267,#47268,#47269,#47270,
#47271,#47272,#47273,#47274,#47275,#47276),.UNSPECIFIED.,.F.,.F.,(4,3,3,
3,3,3,3,4),(-264.186463227569,-263.881920865704,-263.383089257262,-262.884257648821,
-262.385426040379,-261.886594431937,-261.387762823495,-261.275255778348),
 .UNSPECIFIED.);
#414=B_SPLINE_CURVE_WITH_KNOTS('',3,(#47279,#47280,#47281,#47282,#47283,
#47284,#47285,#47286,#47287,#47288,#47289,#47290,#47291,#47292,#47293,#47294,
#47295,#47296,#47297),.UNSPECIFIED.,.F.,.F.,(4,3,3,3,3,3,4),(-1.43852457462426,
-1.3094245422137,-1.20010961474172,-1.15249379404292,-1.12530519830466,
-0.998964743453856,-0.966035327470543),.UNSPECIFIED.);
#415=B_SPLINE_CURVE_WITH_KNOTS('',3,(#47300,#47301,#47302,#47303,#47304,
#47305,#47306,#47307,#47308,#47309,#47310,#47311,#47312,#47313,#47314,#47315,
#47316,#47317,#47318,#47319,#47320,#47321,#47322,#47323,#47324,#47325,#47326,
#47327),.UNSPECIFIED.,.F.,.F.,(4,3,3,3,3,3,3,3,3,4),(-0.664303123679825,
-0.600044533881661,-0.572382428837333,-0.460522004544073,-0.429002315709467,
-0.3217517367821,-0.284511301345448,-0.180801420460334,-0.0803981151576599,
0.),.UNSPECIFIED.);
#416=B_SPLINE_CURVE_WITH_KNOTS('',3,(#49452,#49453,#49454,#49455,#49456,
#49457,#49458,#49459,#49460,#49461,#49462,#49463,#49464,#49465,#49466,#49467,
#49468,#49469,#49470,#49471,#49472,#49473,#49474,#49475,#49476,#49477,#49478,
#49479,#49480,#49481,#49482,#49483,#49484,#49485),.UNSPECIFIED.,.F.,.F.,
(4,3,3,3,3,3,3,3,3,3,3,4),(258.047800828882,258.472551583264,258.972498491549,
259.472445399834,259.972392308118,260.472339216403,260.972286124688,261.472233032973,
261.972179941258,262.472126849543,262.972073757828,263.226194462655),
 .UNSPECIFIED.);
#417=B_SPLINE_CURVE_WITH_KNOTS('',3,(#49487,#49488,#49489,#49490,#49491,
#49492,#49493,#49494,#49495,#49496,#49497,#49498,#49499,#49500,#49501,#49502,
#49503,#49504,#49505,#49506,#49507,#49508,#49509,#49510,#49511,#49512,#49513,
#49514,#49515,#49516,#49517,#49518,#49519,#49520,#49521,#49522,#49523),
 .UNSPECIFIED.,.F.,.F.,(4,3,3,3,3,3,3,3,3,3,3,3,4),(-0.878140325105315,
-0.777010465777669,-0.703471476437966,-0.636654823290452,-0.609982353575103,
-0.500671075341767,-0.483381692174221,-0.406298397291394,-0.367627872926269,
-0.343047565778001,-0.226089388522165,-0.105578325200182,0.),
 .UNSPECIFIED.);
#418=B_SPLINE_CURVE_WITH_KNOTS('',3,(#49524,#49525,#49526,#49527,#49528,
#49529,#49530,#49531,#49532,#49533,#49534,#49535,#49536,#49537,#49538,#49539),
 .UNSPECIFIED.,.F.,.F.,(4,1,1,1,1,1,1,1,1,1,1,1,1,4),(9.94784349116542,
9.98746854282029,10.4874154511051,10.98736235939,11.4873092676748,11.9872561759597,
12.4872030842445,12.9871499925294,13.4870969008142,13.987043809099,14.4869907173839,
14.9869376256687,15.4868845339536,15.7079632679493),.UNSPECIFIED.);
#419=B_SPLINE_CURVE_WITH_KNOTS('',3,(#49557,#49558,#49559,#49560,#49561,
#49562,#49563,#49564,#49565,#49566,#49567,#49568,#49569,#49570,#49571,#49572,
#49573,#49574),.UNSPECIFIED.,.F.,.F.,(4,2,2,2,2,2,2,2,4),(0.,0.0946120580087934,
0.189224116017587,0.283822945575014,0.378421775132442,0.473020604689869,
0.567619434247297,0.66223149225609,0.756843550264884),.UNSPECIFIED.);
#420=B_SPLINE_CURVE_WITH_KNOTS('',3,(#49585,#49586,#49587,#49588,#49589,
#49590,#49591,#49592,#49593,#49594,#49595,#49596,#49597,#49598,#49599,#49600,
#49601,#49602),.UNSPECIFIED.,.F.,.F.,(4,2,2,2,2,2,2,2,4),(-0.756843550264884,
-0.66223149225609,-0.567619434247297,-0.47302060468987,-0.378421775132442,
-0.283822945575015,-0.189224116017587,-0.0946120580087935,0.),
 .UNSPECIFIED.);
#1003=SHAPE_REPRESENTATION_RELATIONSHIP('SRR','None',#76740,#1023);
#1023=ADVANCED_BREP_SHAPE_REPRESENTATION('',(#1063),#76644);
#1043=STYLED_ITEM('',(#76913),#1063);
#1063=MANIFOLD_SOLID_BREP('Feed screw',#26668);
#1160=CYLINDRICAL_SURFACE('',#27590,0.9925);
#1161=CYLINDRICAL_SURFACE('',#27592,0.9925);
#1162=CYLINDRICAL_SURFACE('',#27593,0.9925);
#1163=CYLINDRICAL_SURFACE('',#27594,0.9925);
#1164=CYLINDRICAL_SURFACE('',#27595,0.9925);
#1165=CYLINDRICAL_SURFACE('',#27596,0.9925);
#1166=CYLINDRICAL_SURFACE('',#27597,0.9925);
#1167=CYLINDRICAL_SURFACE('',#27598,0.9925);
#1168=CYLINDRICAL_SURFACE('',#27599,0.9925);
#1169=CYLINDRICAL_SURFACE('',#27600,0.9925);
#1170=CYLINDRICAL_SURFACE('',#27601,0.9925);
#1171=CYLINDRICAL_SURFACE('',#27602,0.9925);
#1172=CYLINDRICAL_SURFACE('',#27603,0.9925);
#1173=CYLINDRICAL_SURFACE('',#27604,0.9925);
#1174=CYLINDRICAL_SURFACE('',#27605,0.9925);
#1175=CYLINDRICAL_SURFACE('',#27606,0.9925);
#1176=CYLINDRICAL_SURFACE('',#27607,0.9925);
#1177=CYLINDRICAL_SURFACE('',#27608,0.9925);
#1178=CYLINDRICAL_SURFACE('',#27609,0.9925);
#1179=CYLINDRICAL_SURFACE('',#27610,0.9925);
#1180=CYLINDRICAL_SURFACE('',#27611,0.9925);
#1181=CYLINDRICAL_SURFACE('',#27612,0.9925);
#1182=CYLINDRICAL_SURFACE('',#27613,0.9925);
#1183=CYLINDRICAL_SURFACE('',#27614,0.9925);
#1184=CYLINDRICAL_SURFACE('',#27615,0.9925);
#1185=CYLINDRICAL_SURFACE('',#27616,0.9925);
#1186=CYLINDRICAL_SURFACE('',#27617,0.9925);
#1187=CYLINDRICAL_SURFACE('',#27618,0.9925);
#1188=CYLINDRICAL_SURFACE('',#27619,0.9925);
#1189=CYLINDRICAL_SURFACE('',#27620,0.9925);
#1190=CYLINDRICAL_SURFACE('',#27621,0.9925);
#1191=CYLINDRICAL_SURFACE('',#27622,0.9925);
#1192=CYLINDRICAL_SURFACE('',#27623,0.9925);
#1193=CYLINDRICAL_SURFACE('',#27624,0.9925);
#1194=CYLINDRICAL_SURFACE('',#27625,0.9925);
#1195=CYLINDRICAL_SURFACE('',#27626,0.9925);
#1196=CYLINDRICAL_SURFACE('',#27627,0.9925);
#1197=CYLINDRICAL_SURFACE('',#27628,0.9925);
#1198=CYLINDRICAL_SURFACE('',#27629,0.9925);
#1199=CYLINDRICAL_SURFACE('',#27630,0.9925);
#1200=CYLINDRICAL_SURFACE('',#27631,0.9925);
#1201=CYLINDRICAL_SURFACE('',#27632,0.9925);
#1202=CYLINDRICAL_SURFACE('',#27633,0.76435);
#1203=CYLINDRICAL_SURFACE('',#27635,0.76435);
#1204=CYLINDRICAL_SURFACE('',#27636,0.76435);
#1205=CYLINDRICAL_SURFACE('',#27637,0.76435);
#1206=CYLINDRICAL_SURFACE('',#27638,0.76435);
#1207=CYLINDRICAL_SURFACE('',#27639,0.76435);
#1208=CYLINDRICAL_SURFACE('',#27640,0.76435);
#1209=CYLINDRICAL_SURFACE('',#27641,0.76435);
#1210=CYLINDRICAL_SURFACE('',#27642,0.76435);
#1211=CYLINDRICAL_SURFACE('',#27643,0.76435);
#1212=CYLINDRICAL_SURFACE('',#27644,0.76435);
#1213=CYLINDRICAL_SURFACE('',#27645,0.76435);
#1214=CYLINDRICAL_SURFACE('',#27646,0.76435);
#1215=CYLINDRICAL_SURFACE('',#27647,0.76435);
#1216=CYLINDRICAL_SURFACE('',#27648,0.76435);
#1217=CYLINDRICAL_SURFACE('',#27649,0.76435);
#1218=CYLINDRICAL_SURFACE('',#27650,0.76435);
#1219=CYLINDRICAL_SURFACE('',#27651,0.76435);
#1220=CYLINDRICAL_SURFACE('',#27652,0.76435);
#1221=CYLINDRICAL_SURFACE('',#27653,0.76435);
#1222=CYLINDRICAL_SURFACE('',#27654,0.76435);
#1223=CYLINDRICAL_SURFACE('',#27655,0.76435);
#1224=CYLINDRICAL_SURFACE('',#27656,0.76435);
#1225=CYLINDRICAL_SURFACE('',#27657,0.76435);
#1226=CYLINDRICAL_SURFACE('',#27658,0.76435);
#1227=CYLINDRICAL_SURFACE('',#27659,0.76435);
#1228=CYLINDRICAL_SURFACE('',#27660,0.76435);
#1229=CYLINDRICAL_SURFACE('',#27661,0.76435);
#1230=CYLINDRICAL_SURFACE('',#27662,0.76435);
#1231=CYLINDRICAL_SURFACE('',#27663,0.76435);
#1232=CYLINDRICAL_SURFACE('',#27664,0.76435);
#1233=CYLINDRICAL_SURFACE('',#27665,0.76435);
#1234=CYLINDRICAL_SURFACE('',#27666,0.76435);
#1235=CYLINDRICAL_SURFACE('',#27667,0.76435);
#1236=CYLINDRICAL_SURFACE('',#27668,0.76435);
#1237=CYLINDRICAL_SURFACE('',#27669,0.76435);
#1238=CYLINDRICAL_SURFACE('',#27670,0.76435);
#1239=CYLINDRICAL_SURFACE('',#27671,0.76435);
#1240=CYLINDRICAL_SURFACE('',#27672,0.76435);
#1241=CYLINDRICAL_SURFACE('',#27673,0.76435);
#1242=CYLINDRICAL_SURFACE('',#27674,0.76435);
#1243=CYLINDRICAL_SURFACE('',#27675,0.76435);
#1244=CYLINDRICAL_SURFACE('',#27688,0.405000000000001);
#1245=CYLINDRICAL_SURFACE('',#27697,0.76435);
#1246=CYLINDRICAL_SURFACE('',#27699,0.9925);
#1247=CYLINDRICAL_SURFACE('',#27702,0.25);
#1248=CYLINDRICAL_SURFACE('',#27705,0.25);
#1249=CYLINDRICAL_SURFACE('',#27710,1.);
#1250=CYLINDRICAL_SURFACE('',#27716,1.6);
#1606=FACE_BOUND('',#4656,.T.);
#1607=FACE_BOUND('',#4672,.T.);
#1608=FACE_BOUND('',#4674,.T.);
#1609=FACE_BOUND('',#4679,.T.);
#1917=PLANE('',#27684);
#1918=PLANE('',#27690);
#1919=PLANE('',#27696);
#1920=PLANE('',#27701);
#1921=PLANE('',#27704);
#1922=PLANE('',#27707);
#1923=PLANE('',#27712);
#1924=PLANE('',#27720);
#2961=FACE_OUTER_BOUND('',#4566,.T.);
#2962=FACE_OUTER_BOUND('',#4567,.T.);
#2963=FACE_OUTER_BOUND('',#4568,.T.);
#2964=FACE_OUTER_BOUND('',#4569,.T.);
#2965=FACE_OUTER_BOUND('',#4570,.T.);
#2966=FACE_OUTER_BOUND('',#4571,.T.);
#2967=FACE_OUTER_BOUND('',#4572,.T.);
#2968=FACE_OUTER_BOUND('',#4573,.T.);
#2969=FACE_OUTER_BOUND('',#4574,.T.);
#2970=FACE_OUTER_BOUND('',#4575,.T.);
#2971=FACE_OUTER_BOUND('',#4576,.T.);
#2972=FACE_OUTER_BOUND('',#4577,.T.);
#2973=FACE_OUTER_BOUND('',#4578,.T.);
#2974=FACE_OUTER_BOUND('',#4579,.T.);
#2975=FACE_OUTER_BOUND('',#4580,.T.);
#2976=FACE_OUTER_BOUND('',#4581,.T.);
#2977=FACE_OUTER_BOUND('',#4582,.T.);
#2978=FACE_OUTER_BOUND('',#4583,.T.);
#2979=FACE_OUTER_BOUND('',#4584,.T.);
#2980=FACE_OUTER_BOUND('',#4585,.T.);
#2981=FACE_OUTER_BOUND('',#4586,.T.);
#2982=FACE_OUTER_BOUND('',#4587,.T.);
#2983=FACE_OUTER_BOUND('',#4588,.T.);
#2984=FACE_OUTER_BOUND('',#4589,.T.);
#2985=FACE_OUTER_BOUND('',#4590,.T.);
#2986=FACE_OUTER_BOUND('',#4591,.T.);
#2987=FACE_OUTER_BOUND('',#4592,.T.);
#2988=FACE_OUTER_BOUND('',#4593,.T.);
#2989=FACE_OUTER_BOUND('',#4594,.T.);
#2990=FACE_OUTER_BOUND('',#4595,.T.);
#2991=FACE_OUTER_BOUND('',#4596,.T.);
#2992=FACE_OUTER_BOUND('',#4597,.T.);
#2993=FACE_OUTER_BOUND('',#4598,.T.);
#2994=FACE_OUTER_BOUND('',#4599,.T.);
#2995=FACE_OUTER_BOUND('',#4600,.T.);
#2996=FACE_OUTER_BOUND('',#4601,.T.);
#2997=FACE_OUTER_BOUND('',#4602,.T.);
#2998=FACE_OUTER_BOUND('',#4603,.T.);
#2999=FACE_OUTER_BOUND('',#4604,.T.);
#3000=FACE_OUTER_BOUND('',#4605,.T.);
#3001=FACE_OUTER_BOUND('',#4606,.T.);
#3002=FACE_OUTER_BOUND('',#4607,.T.);
#3003=FACE_OUTER_BOUND('',#4608,.T.);
#3004=FACE_OUTER_BOUND('',#4609,.T.);
#3005=FACE_OUTER_BOUND('',#4610,.T.);
#3006=FACE_OUTER_BOUND('',#4611,.T.);
#3007=FACE_OUTER_BOUND('',#4612,.T.);
#3008=FACE_OUTER_BOUND('',#4613,.T.);
#3009=FACE_OUTER_BOUND('',#4614,.T.);
#3010=FACE_OUTER_BOUND('',#4615,.T.);
#3011=FACE_OUTER_BOUND('',#4616,.T.);
#3012=FACE_OUTER_BOUND('',#4617,.T.);
#3013=FACE_OUTER_BOUND('',#4618,.T.);
#3014=FACE_OUTER_BOUND('',#4619,.T.);
#3015=FACE_OUTER_BOUND('',#4620,.T.);
#3016=FACE_OUTER_BOUND('',#4621,.T.);
#3017=FACE_OUTER_BOUND('',#4622,.T.);
#3018=FACE_OUTER_BOUND('',#4623,.T.);
#3019=FACE_OUTER_BOUND('',#4624,.T.);
#3020=FACE_OUTER_BOUND('',#4625,.T.);
#3021=FACE_OUTER_BOUND('',#4626,.T.);
#3022=FACE_OUTER_BOUND('',#4627,.T.);
#3023=FACE_OUTER_BOUND('',#4628,.T.);
#3024=FACE_OUTER_BOUND('',#4629,.T.);
#3025=FACE_OUTER_BOUND('',#4630,.T.);
#3026=FACE_OUTER_BOUND('',#4631,.T.);
#3027=FACE_OUTER_BOUND('',#4632,.T.);
#3028=FACE_OUTER_BOUND('',#4633,.T.);
#3029=FACE_OUTER_BOUND('',#4634,.T.);
#3030=FACE_OUTER_BOUND('',#4635,.T.);
#3031=FACE_OUTER_BOUND('',#4636,.T.);
#3032=FACE_OUTER_BOUND('',#4637,.T.);
#3033=FACE_OUTER_BOUND('',#4638,.T.);
#3034=FACE_OUTER_BOUND('',#4639,.T.);
#3035=FACE_OUTER_BOUND('',#4640,.T.);
#3036=FACE_OUTER_BOUND('',#4641,.T.);
#3037=FACE_OUTER_BOUND('',#4642,.T.);
#3038=FACE_OUTER_BOUND('',#4643,.T.);
#3039=FACE_OUTER_BOUND('',#4644,.T.);
#3040=FACE_OUTER_BOUND('',#4645,.T.);
#3041=FACE_OUTER_BOUND('',#4646,.T.);
#3042=FACE_OUTER_BOUND('',#4647,.T.);
#3043=FACE_OUTER_BOUND('',#4648,.T.);
#3044=FACE_OUTER_BOUND('',#4649,.T.);
#3045=FACE_OUTER_BOUND('',#4650,.T.);
#3046=FACE_OUTER_BOUND('',#4651,.T.);
#3047=FACE_OUTER_BOUND('',#4652,.T.);
#3048=FACE_OUTER_BOUND('',#4653,.T.);
#3049=FACE_OUTER_BOUND('',#4654,.T.);
#3050=FACE_OUTER_BOUND('',#4655,.T.);
#3051=FACE_OUTER_BOUND('',#4657,.T.);
#3052=FACE_OUTER_BOUND('',#4658,.T.);
#3053=FACE_OUTER_BOUND('',#4659,.T.);
#3054=FACE_OUTER_BOUND('',#4660,.T.);
#3055=FACE_OUTER_BOUND('',#4661,.T.);
#3056=FACE_OUTER_BOUND('',#4662,.T.);
#3057=FACE_OUTER_BOUND('',#4663,.T.);
#3058=FACE_OUTER_BOUND('',#4664,.T.);
#3059=FACE_OUTER_BOUND('',#4665,.T.);
#3060=FACE_OUTER_BOUND('',#4666,.T.);
#3061=FACE_OUTER_BOUND('',#4667,.T.);
#3062=FACE_OUTER_BOUND('',#4668,.T.);
#3063=FACE_OUTER_BOUND('',#4669,.T.);
#3064=FACE_OUTER_BOUND('',#4670,.T.);
#3065=FACE_OUTER_BOUND('',#4671,.T.);
#3066=FACE_OUTER_BOUND('',#4673,.T.);
#3067=FACE_OUTER_BOUND('',#4675,.T.);
#3068=FACE_OUTER_BOUND('',#4676,.T.);
#3069=FACE_OUTER_BOUND('',#4677,.T.);
#3070=FACE_OUTER_BOUND('',#4678,.T.);
#4566=EDGE_LOOP('',(#19245,#19246,#19247,#19248));
#4567=EDGE_LOOP('',(#19249,#19250,#19251,#19252));
#4568=EDGE_LOOP('',(#19253,#19254,#19255,#19256));
#4569=EDGE_LOOP('',(#19257,#19258,#19259,#19260));
#4570=EDGE_LOOP('',(#19261,#19262,#19263,#19264));
#4571=EDGE_LOOP('',(#19265,#19266,#19267,#19268));
#4572=EDGE_LOOP('',(#19269,#19270,#19271,#19272));
#4573=EDGE_LOOP('',(#19273,#19274,#19275,#19276));
#4574=EDGE_LOOP('',(#19277,#19278,#19279,#19280));
#4575=EDGE_LOOP('',(#19281,#19282,#19283,#19284));
#4576=EDGE_LOOP('',(#19285,#19286,#19287,#19288));
#4577=EDGE_LOOP('',(#19289,#19290,#19291,#19292));
#4578=EDGE_LOOP('',(#19293,#19294,#19295,#19296));
#4579=EDGE_LOOP('',(#19297,#19298,#19299,#19300));
#4580=EDGE_LOOP('',(#19301,#19302,#19303,#19304));
#4581=EDGE_LOOP('',(#19305,#19306,#19307,#19308));
#4582=EDGE_LOOP('',(#19309,#19310,#19311,#19312));
#4583=EDGE_LOOP('',(#19313,#19314,#19315,#19316));
#4584=EDGE_LOOP('',(#19317,#19318,#19319,#19320));
#4585=EDGE_LOOP('',(#19321,#19322,#19323,#19324));
#4586=EDGE_LOOP('',(#19325,#19326,#19327,#19328));
#4587=EDGE_LOOP('',(#19329,#19330,#19331,#19332));
#4588=EDGE_LOOP('',(#19333,#19334,#19335,#19336));
#4589=EDGE_LOOP('',(#19337,#19338,#19339,#19340));
#4590=EDGE_LOOP('',(#19341,#19342,#19343,#19344));
#4591=EDGE_LOOP('',(#19345,#19346,#19347,#19348));
#4592=EDGE_LOOP('',(#19349,#19350,#19351,#19352));
#4593=EDGE_LOOP('',(#19353,#19354,#19355,#19356));
#4594=EDGE_LOOP('',(#19357,#19358,#19359,#19360));
#4595=EDGE_LOOP('',(#19361,#19362,#19363,#19364));
#4596=EDGE_LOOP('',(#19365,#19366,#19367,#19368));
#4597=EDGE_LOOP('',(#19369,#19370,#19371,#19372));
#4598=EDGE_LOOP('',(#19373,#19374,#19375,#19376));
#4599=EDGE_LOOP('',(#19377,#19378,#19379,#19380));
#4600=EDGE_LOOP('',(#19381,#19382,#19383,#19384));
#4601=EDGE_LOOP('',(#19385,#19386,#19387,#19388));
#4602=EDGE_LOOP('',(#19389,#19390,#19391,#19392));
#4603=EDGE_LOOP('',(#19393,#19394,#19395,#19396));
#4604=EDGE_LOOP('',(#19397,#19398,#19399,#19400));
#4605=EDGE_LOOP('',(#19401,#19402,#19403,#19404));
#4606=EDGE_LOOP('',(#19405,#19406,#19407,#19408));
#4607=EDGE_LOOP('',(#19409,#19410,#19411,#19412));
#4608=EDGE_LOOP('',(#19413,#19414,#19415,#19416));
#4609=EDGE_LOOP('',(#19417,#19418,#19419,#19420));
#4610=EDGE_LOOP('',(#19421,#19422,#19423,#19424));
#4611=EDGE_LOOP('',(#19425,#19426,#19427,#19428));
#4612=EDGE_LOOP('',(#19429,#19430,#19431,#19432));
#4613=EDGE_LOOP('',(#19433,#19434,#19435,#19436));
#4614=EDGE_LOOP('',(#19437,#19438,#19439,#19440));
#4615=EDGE_LOOP('',(#19441,#19442,#19443,#19444));
#4616=EDGE_LOOP('',(#19445,#19446,#19447,#19448));
#4617=EDGE_LOOP('',(#19449,#19450,#19451,#19452));
#4618=EDGE_LOOP('',(#19453,#19454,#19455,#19456));
#4619=EDGE_LOOP('',(#19457,#19458,#19459,#19460));
#4620=EDGE_LOOP('',(#19461,#19462,#19463,#19464));
#4621=EDGE_LOOP('',(#19465,#19466,#19467,#19468));
#4622=EDGE_LOOP('',(#19469,#19470,#19471,#19472));
#4623=EDGE_LOOP('',(#19473,#19474,#19475,#19476));
#4624=EDGE_LOOP('',(#19477,#19478,#19479,#19480));
#4625=EDGE_LOOP('',(#19481,#19482,#19483,#19484));
#4626=EDGE_LOOP('',(#19485,#19486,#19487,#19488));
#4627=EDGE_LOOP('',(#19489,#19490,#19491,#19492));
#4628=EDGE_LOOP('',(#19493,#19494,#19495,#19496));
#4629=EDGE_LOOP('',(#19497,#19498,#19499,#19500));
#4630=EDGE_LOOP('',(#19501,#19502,#19503,#19504));
#4631=EDGE_LOOP('',(#19505,#19506,#19507,#19508));
#4632=EDGE_LOOP('',(#19509,#19510,#19511,#19512));
#4633=EDGE_LOOP('',(#19513,#19514,#19515,#19516));
#4634=EDGE_LOOP('',(#19517,#19518,#19519,#19520));
#4635=EDGE_LOOP('',(#19521,#19522,#19523,#19524));
#4636=EDGE_LOOP('',(#19525,#19526,#19527,#19528));
#4637=EDGE_LOOP('',(#19529,#19530,#19531,#19532));
#4638=EDGE_LOOP('',(#19533,#19534,#19535,#19536));
#4639=EDGE_LOOP('',(#19537,#19538,#19539,#19540));
#4640=EDGE_LOOP('',(#19541,#19542,#19543,#19544));
#4641=EDGE_LOOP('',(#19545,#19546,#19547,#19548));
#4642=EDGE_LOOP('',(#19549,#19550,#19551,#19552));
#4643=EDGE_LOOP('',(#19553,#19554,#19555,#19556));
#4644=EDGE_LOOP('',(#19557,#19558,#19559,#19560));
#4645=EDGE_LOOP('',(#19561,#19562,#19563,#19564));
#4646=EDGE_LOOP('',(#19565,#19566,#19567,#19568));
#4647=EDGE_LOOP('',(#19569,#19570,#19571,#19572));
#4648=EDGE_LOOP('',(#19573,#19574,#19575,#19576));
#4649=EDGE_LOOP('',(#19577,#19578,#19579,#19580));
#4650=EDGE_LOOP('',(#19581,#19582,#19583,#19584,#19585));
#4651=EDGE_LOOP('',(#19586,#19587,#19588,#19589,#19590,#19591,#19592));
#4652=EDGE_LOOP('',(#19593));
#4653=EDGE_LOOP('',(#19594,#19595,#19596,#19597));
#4654=EDGE_LOOP('',(#19598,#19599,#19600,#19601));
#4655=EDGE_LOOP('',(#19602));
#4656=EDGE_LOOP('',(#19603));
#4657=EDGE_LOOP('',(#19604,#19605,#19606,#19607,#19608));
#4658=EDGE_LOOP('',(#19609,#19610,#19611,#19612,#19613,#19614,#19615,#19616,
#19617,#19618,#19619,#19620,#19621,#19622,#19623,#19624,#19625,#19626,#19627,
#19628,#19629,#19630,#19631,#19632,#19633,#19634,#19635,#19636,#19637,#19638,
#19639,#19640,#19641,#19642,#19643,#19644,#19645,#19646,#19647,#19648,#19649,
#19650,#19651,#19652,#19653,#19654,#19655,#19656,#19657,#19658,#19659,#19660,
#19661,#19662,#19663,#19664,#19665,#19666,#19667,#19668,#19669,#19670,#19671,
#19672,#19673,#19674,#19675,#19676,#19677,#19678,#19679,#19680,#19681,#19682,
#19683,#19684,#19685,#19686,#19687,#19688,#19689,#19690,#19691,#19692,#19693,
#19694,#19695,#19696,#19697,#19698));
#4659=EDGE_LOOP('',(#19699,#19700,#19701,#19702));
#4660=EDGE_LOOP('',(#19703,#19704,#19705,#19706));
#4661=EDGE_LOOP('',(#19707,#19708,#19709,#19710,#19711,#19712,#19713,#19714,
#19715,#19716,#19717,#19718,#19719,#19720,#19721,#19722,#19723,#19724,#19725,
#19726,#19727,#19728,#19729,#19730,#19731,#19732,#19733,#19734,#19735,#19736,
#19737,#19738,#19739,#19740,#19741,#19742,#19743,#19744,#19745,#19746,#19747,
#19748,#19749,#19750,#19751,#19752,#19753,#19754,#19755,#19756,#19757,#19758,
#19759,#19760,#19761,#19762,#19763,#19764,#19765,#19766,#19767,#19768,#19769,
#19770,#19771,#19772,#19773,#19774,#19775,#19776,#19777,#19778,#19779,#19780,
#19781,#19782,#19783,#19784,#19785,#19786,#19787,#19788,#19789,#19790,#19791,
#19792,#19793,#19794,#19795,#19796));
#4662=EDGE_LOOP('',(#19797,#19798,#19799,#19800));
#4663=EDGE_LOOP('',(#19801,#19802,#19803,#19804));
#4664=EDGE_LOOP('',(#19805,#19806,#19807));
#4665=EDGE_LOOP('',(#19808,#19809,#19810,#19811));
#4666=EDGE_LOOP('',(#19812,#19813,#19814,#19815));
#4667=EDGE_LOOP('',(#19816,#19817,#19818,#19819));
#4668=EDGE_LOOP('',(#19820,#19821,#19822,#19823));
#4669=EDGE_LOOP('',(#19824,#19825,#19826,#19827));
#4670=EDGE_LOOP('',(#19828,#19829,#19830,#19831));
#4671=EDGE_LOOP('',(#19832,#19833,#19834,#19835));
#4672=EDGE_LOOP('',(#19836,#19837,#19838,#19839));
#4673=EDGE_LOOP('',(#19840));
#4674=EDGE_LOOP('',(#19841));
#4675=EDGE_LOOP('',(#19842,#19843,#19844,#19845));
#4676=EDGE_LOOP('',(#19846,#19847,#19848,#19849));
#4677=EDGE_LOOP('',(#19850,#19851,#19852,#19853));
#4678=EDGE_LOOP('',(#19854));
#4679=EDGE_LOOP('',(#19855,#19856,#19857,#19858));
#5983=CIRCLE('',#27591,0.9925);
#5984=CIRCLE('',#27634,0.76435);
#5985=CIRCLE('',#27677,0.85);
#5986=CIRCLE('',#27678,0.935355339059328);
#5987=CIRCLE('',#27679,0.935355339059328);
#5988=CIRCLE('',#27681,0.957144660940674);
#5989=CIRCLE('',#27682,0.95714466094067);
#5990=CIRCLE('',#27683,0.957144660940674);
#5991=CIRCLE('',#27686,0.455000000000002);
#5992=CIRCLE('',#27687,0.405000000000001);
#5993=CIRCLE('',#27689,0.405000000000001);
#5994=CIRCLE('',#27691,0.95);
#5995=CIRCLE('',#27693,0.9925);
#5996=CIRCLE('',#27695,0.942499999999996);
#5997=CIRCLE('',#27698,0.76435);
#5998=CIRCLE('',#27703,0.25);
#5999=CIRCLE('',#27706,0.25);
#6000=CIRCLE('',#27709,1.);
#6001=CIRCLE('',#27711,1.);
#6002=CIRCLE('',#27713,1.55);
#6003=CIRCLE('',#27715,1.6);
#6004=CIRCLE('',#27717,1.6);
#6005=CIRCLE('',#27719,1.55);
#7295=LINE('',#40098,#9451);
#7296=LINE('',#40131,#9452);
#7297=LINE('',#40215,#9453);
#7298=LINE('',#40302,#9454);
#7299=LINE('',#40386,#9455);
#7300=LINE('',#40458,#9456);
#7301=LINE('',#40527,#9457);
#7302=LINE('',#40611,#9458);
#7303=LINE('',#40695,#9459);
#7304=LINE('',#40782,#9460);
#7305=LINE('',#40866,#9461);
#7306=LINE('',#40953,#9462);
#7307=LINE('',#41037,#9463);
#7308=LINE('',#41121,#9464);
#7309=LINE('',#41208,#9465);
#7310=LINE('',#41277,#9466);
#7311=LINE('',#41349,#9467);
#7312=LINE('',#41430,#9468);
#7313=LINE('',#41517,#9469);
#7314=LINE('',#41604,#9470);
#7315=LINE('',#41688,#9471);
#7316=LINE('',#41775,#9472);
#7317=LINE('',#41847,#9473);
#7318=LINE('',#41937,#9474);
#7319=LINE('',#42021,#9475);
#7320=LINE('',#42105,#9476);
#7321=LINE('',#42192,#9477);
#7322=LINE('',#42273,#9478);
#7323=LINE('',#42345,#9479);
#7324=LINE('',#42414,#9480);
#7325=LINE('',#42498,#9481);
#7326=LINE('',#42582,#9482);
#7327=LINE('',#42666,#9483);
#7328=LINE('',#42756,#9484);
#7329=LINE('',#42840,#9485);
#7330=LINE('',#42924,#9486);
#7331=LINE('',#43008,#9487);
#7332=LINE('',#43092,#9488);
#7333=LINE('',#43161,#9489);
#7334=LINE('',#43245,#9490);
#7335=LINE('',#43332,#9491);
#7336=LINE('',#43416,#9492);
#7337=LINE('',#43500,#9493);
#7338=LINE('',#43522,#9494);
#7339=LINE('',#43557,#9495);
#7340=LINE('',#43594,#9496);
#7341=LINE('',#43630,#9497);
#7342=LINE('',#43666,#9498);
#7343=LINE('',#43712,#9499);
#7344=LINE('',#43747,#9500);
#7345=LINE('',#43784,#9501);
#7346=LINE('',#43819,#9502);
#7347=LINE('',#43856,#9503);
#7348=LINE('',#43893,#9504);
#7349=LINE('',#43929,#9505);
#7350=LINE('',#43966,#9506);
#7351=LINE('',#44001,#9507);
#7352=LINE('',#44038,#9508);
#7353=LINE('',#44083,#9509);
#7354=LINE('',#44119,#9510);
#7355=LINE('',#44155,#9511);
#7356=LINE('',#44191,#9512);
#7357=LINE('',#44228,#9513);
#7358=LINE('',#44265,#9514);
#7359=LINE('',#44300,#9515);
#7360=LINE('',#44334,#9516);
#7361=LINE('',#44371,#9517);
#7362=LINE('',#44407,#9518);
#7363=LINE('',#44444,#9519);
#7364=LINE('',#44480,#9520);
#7365=LINE('',#44516,#9521);
#7366=LINE('',#44552,#9522);
#7367=LINE('',#44588,#9523);
#7368=LINE('',#44625,#9524);
#7369=LINE('',#44660,#9525);
#7370=LINE('',#44697,#9526);
#7371=LINE('',#44734,#9527);
#7372=LINE('',#44770,#9528);
#7373=LINE('',#44807,#9529);
#7374=LINE('',#44842,#9530);
#7375=LINE('',#44879,#9531);
#7376=LINE('',#44914,#9532);
#7377=LINE('',#44951,#9533);
#7378=LINE('',#44987,#9534);
#7379=LINE('',#45024,#9535);
#7380=LINE('',#45030,#9536);
#7381=LINE('',#45041,#9537);
#7382=LINE('',#45046,#9538);
#7383=LINE('',#49545,#9539);
#7384=LINE('',#49549,#9540);
#7385=LINE('',#49551,#9541);
#7386=LINE('',#49553,#9542);
#7387=LINE('',#49554,#9543);
#7388=LINE('',#49577,#9544);
#7389=LINE('',#49580,#9545);
#7390=LINE('',#49582,#9546);
#7391=LINE('',#49583,#9547);
#7392=LINE('',#49608,#9548);
#7393=LINE('',#49612,#9549);
#7394=LINE('',#49619,#9550);
#7395=LINE('',#49623,#9551);
#7396=LINE('',#49627,#9552);
#9451=VECTOR('',#31420,1.);
#9452=VECTOR('',#31425,1.);
#9453=VECTOR('',#31428,1.);
#9454=VECTOR('',#31431,1.);
#9455=VECTOR('',#31434,1.);
#9456=VECTOR('',#31437,1.);
#9457=VECTOR('',#31440,1.);
#9458=VECTOR('',#31443,1.);
#9459=VECTOR('',#31446,1.);
#9460=VECTOR('',#31449,1.);
#9461=VECTOR('',#31452,1.);
#9462=VECTOR('',#31455,1.);
#9463=VECTOR('',#31458,1.);
#9464=VECTOR('',#31461,1.);
#9465=VECTOR('',#31464,1.);
#9466=VECTOR('',#31467,1.);
#9467=VECTOR('',#31470,1.);
#9468=VECTOR('',#31473,1.);
#9469=VECTOR('',#31476,1.);
#9470=VECTOR('',#31479,1.);
#9471=VECTOR('',#31482,1.);
#9472=VECTOR('',#31485,1.);
#9473=VECTOR('',#31488,1.);
#9474=VECTOR('',#31491,1.);
#9475=VECTOR('',#31494,1.);
#9476=VECTOR('',#31497,1.);
#9477=VECTOR('',#31500,1.);
#9478=VECTOR('',#31503,1.);
#9479=VECTOR('',#31506,1.);
#9480=VECTOR('',#31509,1.);
#9481=VECTOR('',#31512,1.);
#9482=VECTOR('',#31515,1.);
#9483=VECTOR('',#31518,1.);
#9484=VECTOR('',#31521,1.);
#9485=VECTOR('',#31524,1.);
#9486=VECTOR('',#31527,1.);
#9487=VECTOR('',#31530,1.);
#9488=VECTOR('',#31533,1.);
#9489=VECTOR('',#31536,1.);
#9490=VECTOR('',#31539,1.);
#9491=VECTOR('',#31542,1.);
#9492=VECTOR('',#31545,1.);
#9493=VECTOR('',#31548,0.76435);
#9494=VECTOR('',#31553,0.76435);
#9495=VECTOR('',#31556,0.76435);
#9496=VECTOR('',#31559,0.76435);
#9497=VECTOR('',#31562,0.76435);
#9498=VECTOR('',#31565,0.76435);
#9499=VECTOR('',#31568,0.76435);
#9500=VECTOR('',#31571,0.76435);
#9501=VECTOR('',#31574,0.76435);
#9502=VECTOR('',#31577,0.76435);
#9503=VECTOR('',#31580,0.76435);
#9504=VECTOR('',#31583,0.76435);
#9505=VECTOR('',#31586,0.76435);
#9506=VECTOR('',#31589,0.76435);
#9507=VECTOR('',#31592,0.76435);
#9508=VECTOR('',#31595,0.76435);
#9509=VECTOR('',#31598,0.76435);
#9510=VECTOR('',#31601,0.76435);
#9511=VECTOR('',#31604,0.76435);
#9512=VECTOR('',#31607,0.76435);
#9513=VECTOR('',#31610,0.76435);
#9514=VECTOR('',#31613,0.76435);
#9515=VECTOR('',#31616,0.76435);
#9516=VECTOR('',#31619,0.76435);
#9517=VECTOR('',#31622,0.76435);
#9518=VECTOR('',#31625,0.76435);
#9519=VECTOR('',#31628,0.76435);
#9520=VECTOR('',#31631,0.76435);
#9521=VECTOR('',#31634,0.76435);
#9522=VECTOR('',#31637,0.76435);
#9523=VECTOR('',#31640,0.76435);
#9524=VECTOR('',#31643,0.76435);
#9525=VECTOR('',#31646,0.76435);
#9526=VECTOR('',#31649,0.76435);
#9527=VECTOR('',#31652,0.76435);
#9528=VECTOR('',#31655,0.76435);
#9529=VECTOR('',#31658,0.76435);
#9530=VECTOR('',#31661,0.76435);
#9531=VECTOR('',#31664,0.76435);
#9532=VECTOR('',#31667,0.76435);
#9533=VECTOR('',#31670,0.76435);
#9534=VECTOR('',#31673,0.76435);
#9535=VECTOR('',#31678,0.892677669529664);
#9536=VECTOR('',#31685,0.95);
#9537=VECTOR('',#31698,0.430000000000001);
#9538=VECTOR('',#31705,0.405000000000001);
#9539=VECTOR('',#31728,0.202500000000001);
#9540=VECTOR('',#31731,1.);
#9541=VECTOR('',#31732,1.);
#9542=VECTOR('',#31733,1.);
#9543=VECTOR('',#31734,1.);
#9544=VECTOR('',#31739,1.);
#9545=VECTOR('',#31742,1.);
#9546=VECTOR('',#31743,1.);
#9547=VECTOR('',#31744,1.);
#9548=VECTOR('',#31755,0.975);
#9549=VECTOR('',#31760,1.);
#9550=VECTOR('',#31769,1.575);
#9551=VECTOR('',#31774,1.6);
#9552=VECTOR('',#31779,1.575);
#11534=VERTEX_POINT('',#40096);
#11535=VERTEX_POINT('',#40097);
#11536=VERTEX_POINT('',#40099);
#11537=VERTEX_POINT('',#40122);
#11538=VERTEX_POINT('',#40129);
#11539=VERTEX_POINT('',#40130);
#11540=VERTEX_POINT('',#40213);
#11541=VERTEX_POINT('',#40214);
#11542=VERTEX_POINT('',#40300);
#11543=VERTEX_POINT('',#40301);
#11544=VERTEX_POINT('',#40384);
#11545=VERTEX_POINT('',#40385);
#11546=VERTEX_POINT('',#40456);
#11547=VERTEX_POINT('',#40457);
#11548=VERTEX_POINT('',#40525);
#11549=VERTEX_POINT('',#40526);
#11550=VERTEX_POINT('',#40609);
#11551=VERTEX_POINT('',#40610);
#11552=VERTEX_POINT('',#40693);
#11553=VERTEX_POINT('',#40694);
#11554=VERTEX_POINT('',#40780);
#11555=VERTEX_POINT('',#40781);
#11556=VERTEX_POINT('',#40864);
#11557=VERTEX_POINT('',#40865);
#11558=VERTEX_POINT('',#40951);
#11559=VERTEX_POINT('',#40952);
#11560=VERTEX_POINT('',#41035);
#11561=VERTEX_POINT('',#41036);
#11562=VERTEX_POINT('',#41119);
#11563=VERTEX_POINT('',#41120);
#11564=VERTEX_POINT('',#41206);
#11565=VERTEX_POINT('',#41207);
#11566=VERTEX_POINT('',#41275);
#11567=VERTEX_POINT('',#41276);
#11568=VERTEX_POINT('',#41347);
#11569=VERTEX_POINT('',#41348);
#11570=VERTEX_POINT('',#41428);
#11571=VERTEX_POINT('',#41429);
#11572=VERTEX_POINT('',#41515);
#11573=VERTEX_POINT('',#41516);
#11574=VERTEX_POINT('',#41602);
#11575=VERTEX_POINT('',#41603);
#11576=VERTEX_POINT('',#41686);
#11577=VERTEX_POINT('',#41687);
#11578=VERTEX_POINT('',#41773);
#11579=VERTEX_POINT('',#41774);
#11580=VERTEX_POINT('',#41845);
#11581=VERTEX_POINT('',#41846);
#11582=VERTEX_POINT('',#41935);
#11583=VERTEX_POINT('',#41936);
#11584=VERTEX_POINT('',#42019);
#11585=VERTEX_POINT('',#42020);
#11586=VERTEX_POINT('',#42103);
#11587=VERTEX_POINT('',#42104);
#11588=VERTEX_POINT('',#42190);
#11589=VERTEX_POINT('',#42191);
#11590=VERTEX_POINT('',#42271);
#11591=VERTEX_POINT('',#42272);
#11592=VERTEX_POINT('',#42343);
#11593=VERTEX_POINT('',#42344);
#11594=VERTEX_POINT('',#42412);
#11595=VERTEX_POINT('',#42413);
#11596=VERTEX_POINT('',#42496);
#11597=VERTEX_POINT('',#42497);
#11598=VERTEX_POINT('',#42580);
#11599=VERTEX_POINT('',#42581);
#11600=VERTEX_POINT('',#42664);
#11601=VERTEX_POINT('',#42665);
#11602=VERTEX_POINT('',#42754);
#11603=VERTEX_POINT('',#42755);
#11604=VERTEX_POINT('',#42838);
#11605=VERTEX_POINT('',#42839);
#11606=VERTEX_POINT('',#42922);
#11607=VERTEX_POINT('',#42923);
#11608=VERTEX_POINT('',#43006);
#11609=VERTEX_POINT('',#43007);
#11610=VERTEX_POINT('',#43090);
#11611=VERTEX_POINT('',#43091);
#11612=VERTEX_POINT('',#43159);
#11613=VERTEX_POINT('',#43160);
#11614=VERTEX_POINT('',#43243);
#11615=VERTEX_POINT('',#43244);
#11616=VERTEX_POINT('',#43330);
#11617=VERTEX_POINT('',#43331);
#11618=VERTEX_POINT('',#43414);
#11619=VERTEX_POINT('',#43415);
#11620=VERTEX_POINT('',#43498);
#11621=VERTEX_POINT('',#43499);
#11622=VERTEX_POINT('',#43501);
#11623=VERTEX_POINT('',#43512);
#11624=VERTEX_POINT('',#43520);
#11625=VERTEX_POINT('',#43521);
#11626=VERTEX_POINT('',#43555);
#11627=VERTEX_POINT('',#43556);
#11628=VERTEX_POINT('',#43592);
#11629=VERTEX_POINT('',#43593);
#11630=VERTEX_POINT('',#43628);
#11631=VERTEX_POINT('',#43629);
#11632=VERTEX_POINT('',#43664);
#11633=VERTEX_POINT('',#43665);
#11634=VERTEX_POINT('',#43710);
#11635=VERTEX_POINT('',#43711);
#11636=VERTEX_POINT('',#43745);
#11637=VERTEX_POINT('',#43746);
#11638=VERTEX_POINT('',#43782);
#11639=VERTEX_POINT('',#43783);
#11640=VERTEX_POINT('',#43817);
#11641=VERTEX_POINT('',#43818);
#11642=VERTEX_POINT('',#43854);
#11643=VERTEX_POINT('',#43855);
#11644=VERTEX_POINT('',#43891);
#11645=VERTEX_POINT('',#43892);
#11646=VERTEX_POINT('',#43927);
#11647=VERTEX_POINT('',#43928);
#11648=VERTEX_POINT('',#43964);
#11649=VERTEX_POINT('',#43965);
#11650=VERTEX_POINT('',#43999);
#11651=VERTEX_POINT('',#44000);
#11652=VERTEX_POINT('',#44036);
#11653=VERTEX_POINT('',#44037);
#11654=VERTEX_POINT('',#44081);
#11655=VERTEX_POINT('',#44082);
#11656=VERTEX_POINT('',#44117);
#11657=VERTEX_POINT('',#44118);
#11658=VERTEX_POINT('',#44153);
#11659=VERTEX_POINT('',#44154);
#11660=VERTEX_POINT('',#44189);
#11661=VERTEX_POINT('',#44190);
#11662=VERTEX_POINT('',#44226);
#11663=VERTEX_POINT('',#44227);
#11664=VERTEX_POINT('',#44263);
#11665=VERTEX_POINT('',#44264);
#11666=VERTEX_POINT('',#44298);
#11667=VERTEX_POINT('',#44299);
#11668=VERTEX_POINT('',#44332);
#11669=VERTEX_POINT('',#44333);
#11670=VERTEX_POINT('',#44369);
#11671=VERTEX_POINT('',#44370);
#11672=VERTEX_POINT('',#44405);
#11673=VERTEX_POINT('',#44406);
#11674=VERTEX_POINT('',#44442);
#11675=VERTEX_POINT('',#44443);
#11676=VERTEX_POINT('',#44478);
#11677=VERTEX_POINT('',#44479);
#11678=VERTEX_POINT('',#44514);
#11679=VERTEX_POINT('',#44515);
#11680=VERTEX_POINT('',#44550);
#11681=VERTEX_POINT('',#44551);
#11682=VERTEX_POINT('',#44586);
#11683=VERTEX_POINT('',#44587);
#11684=VERTEX_POINT('',#44623);
#11685=VERTEX_POINT('',#44624);
#11686=VERTEX_POINT('',#44658);
#11687=VERTEX_POINT('',#44659);
#11688=VERTEX_POINT('',#44695);
#11689=VERTEX_POINT('',#44696);
#11690=VERTEX_POINT('',#44732);
#11691=VERTEX_POINT('',#44733);
#11692=VERTEX_POINT('',#44768);
#11693=VERTEX_POINT('',#44769);
#11694=VERTEX_POINT('',#44805);
#11695=VERTEX_POINT('',#44806);
#11696=VERTEX_POINT('',#44840);
#11697=VERTEX_POINT('',#44841);
#11698=VERTEX_POINT('',#44877);
#11699=VERTEX_POINT('',#44878);
#11700=VERTEX_POINT('',#44912);
#11701=VERTEX_POINT('',#44913);
#11702=VERTEX_POINT('',#44949);
#11703=VERTEX_POINT('',#44950);
#11704=VERTEX_POINT('',#44985);
#11705=VERTEX_POINT('',#44986);
#11706=VERTEX_POINT('',#45021);
#11707=VERTEX_POINT('',#45023);
#11708=VERTEX_POINT('',#45025);
#11709=VERTEX_POINT('',#45029);
#11710=VERTEX_POINT('',#45031);
#11711=VERTEX_POINT('',#45033);
#11712=VERTEX_POINT('',#45038);
#11713=VERTEX_POINT('',#45040);
#11714=VERTEX_POINT('',#45044);
#11715=VERTEX_POINT('',#45048);
#11716=VERTEX_POINT('',#45051);
#11717=VERTEX_POINT('',#45113);
#11718=VERTEX_POINT('',#47152);
#11719=VERTEX_POINT('',#47209);
#11720=VERTEX_POINT('',#47278);
#11721=VERTEX_POINT('',#49486);
#11722=VERTEX_POINT('',#49544);
#11723=VERTEX_POINT('',#49547);
#11724=VERTEX_POINT('',#49548);
#11725=VERTEX_POINT('',#49550);
#11726=VERTEX_POINT('',#49552);
#11727=VERTEX_POINT('',#49556);
#11728=VERTEX_POINT('',#49575);
#11729=VERTEX_POINT('',#49579);
#11730=VERTEX_POINT('',#49581);
#11731=VERTEX_POINT('',#49606);
#11732=VERTEX_POINT('',#49610);
#11733=VERTEX_POINT('',#49614);
#11734=VERTEX_POINT('',#49617);
#11735=VERTEX_POINT('',#49621);
#11736=VERTEX_POINT('',#49625);
#14345=EDGE_CURVE('',#11534,#11535,#7295,.T.);
#14346=EDGE_CURVE('',#11534,#11536,#239,.T.);
#14347=EDGE_CURVE('',#11536,#11537,#5983,.F.);
#14348=EDGE_CURVE('',#11537,#11535,#240,.T.);
#14349=EDGE_CURVE('',#11538,#11539,#7296,.T.);
#14350=EDGE_CURVE('',#11538,#11534,#241,.T.);
#14351=EDGE_CURVE('',#11535,#11539,#242,.T.);
#14352=EDGE_CURVE('',#11540,#11541,#7297,.T.);
#14353=EDGE_CURVE('',#11540,#11538,#243,.T.);
#14354=EDGE_CURVE('',#11539,#11541,#244,.T.);
#14355=EDGE_CURVE('',#11542,#11543,#7298,.T.);
#14356=EDGE_CURVE('',#11542,#11540,#245,.T.);
#14357=EDGE_CURVE('',#11541,#11543,#246,.T.);
#14358=EDGE_CURVE('',#11544,#11545,#7299,.T.);
#14359=EDGE_CURVE('',#11544,#11542,#247,.T.);
#14360=EDGE_CURVE('',#11543,#11545,#248,.T.);
#14361=EDGE_CURVE('',#11546,#11547,#7300,.T.);
#14362=EDGE_CURVE('',#11546,#11544,#249,.T.);
#14363=EDGE_CURVE('',#11545,#11547,#250,.T.);
#14364=EDGE_CURVE('',#11548,#11549,#7301,.T.);
#14365=EDGE_CURVE('',#11548,#11546,#251,.T.);
#14366=EDGE_CURVE('',#11547,#11549,#252,.T.);
#14367=EDGE_CURVE('',#11550,#11551,#7302,.T.);
#14368=EDGE_CURVE('',#11550,#11548,#253,.T.);
#14369=EDGE_CURVE('',#11549,#11551,#254,.T.);
#14370=EDGE_CURVE('',#11552,#11553,#7303,.T.);
#14371=EDGE_CURVE('',#11552,#11550,#255,.T.);
#14372=EDGE_CURVE('',#11551,#11553,#256,.T.);
#14373=EDGE_CURVE('',#11554,#11555,#7304,.T.);
#14374=EDGE_CURVE('',#11554,#11552,#257,.T.);
#14375=EDGE_CURVE('',#11553,#11555,#258,.T.);
#14376=EDGE_CURVE('',#11556,#11557,#7305,.T.);
#14377=EDGE_CURVE('',#11556,#11554,#259,.T.);
#14378=EDGE_CURVE('',#11555,#11557,#260,.T.);
#14379=EDGE_CURVE('',#11558,#11559,#7306,.T.);
#14380=EDGE_CURVE('',#11558,#11556,#261,.T.);
#14381=EDGE_CURVE('',#11557,#11559,#262,.T.);
#14382=EDGE_CURVE('',#11560,#11561,#7307,.T.);
#14383=EDGE_CURVE('',#11560,#11558,#263,.T.);
#14384=EDGE_CURVE('',#11559,#11561,#264,.T.);
#14385=EDGE_CURVE('',#11562,#11563,#7308,.T.);
#14386=EDGE_CURVE('',#11562,#11560,#265,.T.);
#14387=EDGE_CURVE('',#11561,#11563,#266,.T.);
#14388=EDGE_CURVE('',#11564,#11565,#7309,.T.);
#14389=EDGE_CURVE('',#11564,#11562,#267,.T.);
#14390=EDGE_CURVE('',#11563,#11565,#268,.T.);
#14391=EDGE_CURVE('',#11566,#11567,#7310,.T.);
#14392=EDGE_CURVE('',#11566,#11564,#269,.T.);
#14393=EDGE_CURVE('',#11565,#11567,#270,.T.);
#14394=EDGE_CURVE('',#11568,#11569,#7311,.T.);
#14395=EDGE_CURVE('',#11568,#11566,#271,.T.);
#14396=EDGE_CURVE('',#11567,#11569,#272,.T.);
#14397=EDGE_CURVE('',#11570,#11571,#7312,.T.);
#14398=EDGE_CURVE('',#11570,#11568,#273,.T.);
#14399=EDGE_CURVE('',#11569,#11571,#274,.T.);
#14400=EDGE_CURVE('',#11572,#11573,#7313,.T.);
#14401=EDGE_CURVE('',#11572,#11570,#275,.T.);
#14402=EDGE_CURVE('',#11571,#11573,#276,.T.);
#14403=EDGE_CURVE('',#11574,#11575,#7314,.T.);
#14404=EDGE_CURVE('',#11574,#11572,#277,.T.);
#14405=EDGE_CURVE('',#11573,#11575,#278,.T.);
#14406=EDGE_CURVE('',#11576,#11577,#7315,.T.);
#14407=EDGE_CURVE('',#11576,#11574,#279,.T.);
#14408=EDGE_CURVE('',#11575,#11577,#280,.T.);
#14409=EDGE_CURVE('',#11578,#11579,#7316,.T.);
#14410=EDGE_CURVE('',#11578,#11576,#281,.T.);
#14411=EDGE_CURVE('',#11577,#11579,#282,.T.);
#14412=EDGE_CURVE('',#11580,#11581,#7317,.T.);
#14413=EDGE_CURVE('',#11580,#11578,#283,.T.);
#14414=EDGE_CURVE('',#11579,#11581,#284,.T.);
#14415=EDGE_CURVE('',#11582,#11583,#7318,.T.);
#14416=EDGE_CURVE('',#11582,#11580,#285,.T.);
#14417=EDGE_CURVE('',#11581,#11583,#286,.T.);
#14418=EDGE_CURVE('',#11584,#11585,#7319,.T.);
#14419=EDGE_CURVE('',#11584,#11582,#287,.T.);
#14420=EDGE_CURVE('',#11583,#11585,#288,.T.);
#14421=EDGE_CURVE('',#11586,#11587,#7320,.T.);
#14422=EDGE_CURVE('',#11586,#11584,#289,.T.);
#14423=EDGE_CURVE('',#11585,#11587,#290,.T.);
#14424=EDGE_CURVE('',#11588,#11589,#7321,.T.);
#14425=EDGE_CURVE('',#11588,#11586,#291,.T.);
#14426=EDGE_CURVE('',#11587,#11589,#292,.T.);
#14427=EDGE_CURVE('',#11590,#11591,#7322,.T.);
#14428=EDGE_CURVE('',#11590,#11588,#293,.T.);
#14429=EDGE_CURVE('',#11589,#11591,#294,.T.);
#14430=EDGE_CURVE('',#11592,#11593,#7323,.T.);
#14431=EDGE_CURVE('',#11592,#11590,#295,.T.);
#14432=EDGE_CURVE('',#11591,#11593,#296,.T.);
#14433=EDGE_CURVE('',#11594,#11595,#7324,.T.);
#14434=EDGE_CURVE('',#11594,#11592,#297,.T.);
#14435=EDGE_CURVE('',#11593,#11595,#298,.T.);
#14436=EDGE_CURVE('',#11596,#11597,#7325,.T.);
#14437=EDGE_CURVE('',#11596,#11594,#299,.T.);
#14438=EDGE_CURVE('',#11595,#11597,#300,.T.);
#14439=EDGE_CURVE('',#11598,#11599,#7326,.T.);
#14440=EDGE_CURVE('',#11598,#11596,#301,.T.);
#14441=EDGE_CURVE('',#11597,#11599,#302,.T.);
#14442=EDGE_CURVE('',#11600,#11601,#7327,.T.);
#14443=EDGE_CURVE('',#11600,#11598,#303,.T.);
#14444=EDGE_CURVE('',#11599,#11601,#304,.T.);
#14445=EDGE_CURVE('',#11602,#11603,#7328,.T.);
#14446=EDGE_CURVE('',#11602,#11600,#305,.T.);
#14447=EDGE_CURVE('',#11601,#11603,#306,.T.);
#14448=EDGE_CURVE('',#11604,#11605,#7329,.T.);
#14449=EDGE_CURVE('',#11604,#11602,#307,.T.);
#14450=EDGE_CURVE('',#11603,#11605,#308,.T.);
#14451=EDGE_CURVE('',#11606,#11607,#7330,.T.);
#14452=EDGE_CURVE('',#11606,#11604,#309,.T.);
#14453=EDGE_CURVE('',#11605,#11607,#310,.T.);
#14454=EDGE_CURVE('',#11608,#11609,#7331,.T.);
#14455=EDGE_CURVE('',#11608,#11606,#311,.T.);
#14456=EDGE_CURVE('',#11607,#11609,#312,.T.);
#14457=EDGE_CURVE('',#11610,#11611,#7332,.T.);
#14458=EDGE_CURVE('',#11610,#11608,#313,.T.);
#14459=EDGE_CURVE('',#11609,#11611,#314,.T.);
#14460=EDGE_CURVE('',#11612,#11613,#7333,.T.);
#14461=EDGE_CURVE('',#11612,#11610,#315,.T.);
#14462=EDGE_CURVE('',#11611,#11613,#316,.T.);
#14463=EDGE_CURVE('',#11614,#11615,#7334,.T.);
#14464=EDGE_CURVE('',#11614,#11612,#317,.T.);
#14465=EDGE_CURVE('',#11613,#11615,#318,.T.);
#14466=EDGE_CURVE('',#11616,#11617,#7335,.T.);
#14467=EDGE_CURVE('',#11616,#11614,#319,.T.);
#14468=EDGE_CURVE('',#11615,#11617,#320,.T.);
#14469=EDGE_CURVE('',#11618,#11619,#7336,.T.);
#14470=EDGE_CURVE('',#11618,#11616,#321,.T.);
#14471=EDGE_CURVE('',#11617,#11619,#322,.T.);
#14472=EDGE_CURVE('',#11620,#11621,#7337,.T.);
#14473=EDGE_CURVE('',#11620,#11622,#323,.T.);
#14474=EDGE_CURVE('',#11623,#11622,#5984,.T.);
#14475=EDGE_CURVE('',#11621,#11623,#324,.T.);
#14476=EDGE_CURVE('',#11624,#11625,#7338,.T.);
#14477=EDGE_CURVE('',#11624,#11620,#325,.T.);
#14478=EDGE_CURVE('',#11625,#11621,#326,.T.);
#14479=EDGE_CURVE('',#11626,#11627,#7339,.T.);
#14480=EDGE_CURVE('',#11626,#11624,#327,.T.);
#14481=EDGE_CURVE('',#11627,#11625,#328,.T.);
#14482=EDGE_CURVE('',#11628,#11629,#7340,.T.);
#14483=EDGE_CURVE('',#11628,#11626,#329,.T.);
#14484=EDGE_CURVE('',#11629,#11627,#330,.T.);
#14485=EDGE_CURVE('',#11630,#11631,#7341,.T.);
#14486=EDGE_CURVE('',#11630,#11628,#331,.T.);
#14487=EDGE_CURVE('',#11631,#11629,#332,.T.);
#14488=EDGE_CURVE('',#11632,#11633,#7342,.T.);
#14489=EDGE_CURVE('',#11632,#11630,#333,.T.);
#14490=EDGE_CURVE('',#11633,#11631,#334,.T.);
#14491=EDGE_CURVE('',#11634,#11635,#7343,.T.);
#14492=EDGE_CURVE('',#11634,#11632,#335,.T.);
#14493=EDGE_CURVE('',#11635,#11633,#336,.T.);
#14494=EDGE_CURVE('',#11636,#11637,#7344,.T.);
#14495=EDGE_CURVE('',#11636,#11634,#337,.T.);
#14496=EDGE_CURVE('',#11637,#11635,#338,.T.);
#14497=EDGE_CURVE('',#11638,#11639,#7345,.T.);
#14498=EDGE_CURVE('',#11638,#11636,#339,.T.);
#14499=EDGE_CURVE('',#11639,#11637,#340,.T.);
#14500=EDGE_CURVE('',#11640,#11641,#7346,.T.);
#14501=EDGE_CURVE('',#11640,#11638,#341,.T.);
#14502=EDGE_CURVE('',#11641,#11639,#342,.T.);
#14503=EDGE_CURVE('',#11642,#11643,#7347,.T.);
#14504=EDGE_CURVE('',#11642,#11640,#343,.T.);
#14505=EDGE_CURVE('',#11643,#11641,#344,.T.);
#14506=EDGE_CURVE('',#11644,#11645,#7348,.T.);
#14507=EDGE_CURVE('',#11644,#11642,#345,.T.);
#14508=EDGE_CURVE('',#11645,#11643,#346,.T.);
#14509=EDGE_CURVE('',#11646,#11647,#7349,.T.);
#14510=EDGE_CURVE('',#11646,#11644,#347,.T.);
#14511=EDGE_CURVE('',#11647,#11645,#348,.T.);
#14512=EDGE_CURVE('',#11648,#11649,#7350,.T.);
#14513=EDGE_CURVE('',#11648,#11646,#349,.T.);
#14514=EDGE_CURVE('',#11649,#11647,#350,.T.);
#14515=EDGE_CURVE('',#11650,#11651,#7351,.T.);
#14516=EDGE_CURVE('',#11650,#11648,#351,.T.);
#14517=EDGE_CURVE('',#11651,#11649,#352,.T.);
#14518=EDGE_CURVE('',#11652,#11653,#7352,.T.);
#14519=EDGE_CURVE('',#11652,#11650,#353,.T.);
#14520=EDGE_CURVE('',#11653,#11651,#354,.T.);
#14521=EDGE_CURVE('',#11654,#11655,#7353,.T.);
#14522=EDGE_CURVE('',#11654,#11652,#355,.T.);
#14523=EDGE_CURVE('',#11655,#11653,#356,.T.);
#14524=EDGE_CURVE('',#11656,#11657,#7354,.T.);
#14525=EDGE_CURVE('',#11656,#11654,#357,.T.);
#14526=EDGE_CURVE('',#11657,#11655,#358,.T.);
#14527=EDGE_CURVE('',#11658,#11659,#7355,.T.);
#14528=EDGE_CURVE('',#11658,#11656,#359,.T.);
#14529=EDGE_CURVE('',#11659,#11657,#360,.T.);
#14530=EDGE_CURVE('',#11660,#11661,#7356,.T.);
#14531=EDGE_CURVE('',#11660,#11658,#361,.T.);
#14532=EDGE_CURVE('',#11661,#11659,#362,.T.);
#14533=EDGE_CURVE('',#11662,#11663,#7357,.T.);
#14534=EDGE_CURVE('',#11662,#11660,#363,.T.);
#14535=EDGE_CURVE('',#11663,#11661,#364,.T.);
#14536=EDGE_CURVE('',#11664,#11665,#7358,.T.);
#14537=EDGE_CURVE('',#11664,#11662,#365,.T.);
#14538=EDGE_CURVE('',#11665,#11663,#366,.T.);
#14539=EDGE_CURVE('',#11666,#11667,#7359,.T.);
#14540=EDGE_CURVE('',#11666,#11664,#367,.T.);
#14541=EDGE_CURVE('',#11667,#11665,#368,.T.);
#14542=EDGE_CURVE('',#11668,#11669,#7360,.T.);
#14543=EDGE_CURVE('',#11668,#11666,#369,.T.);
#14544=EDGE_CURVE('',#11669,#11667,#370,.T.);
#14545=EDGE_CURVE('',#11670,#11671,#7361,.T.);
#14546=EDGE_CURVE('',#11670,#11668,#371,.T.);
#14547=EDGE_CURVE('',#11671,#11669,#372,.T.);
#14548=EDGE_CURVE('',#11672,#11673,#7362,.T.);
#14549=EDGE_CURVE('',#11672,#11670,#373,.T.);
#14550=EDGE_CURVE('',#11673,#11671,#374,.T.);
#14551=EDGE_CURVE('',#11674,#11675,#7363,.T.);
#14552=EDGE_CURVE('',#11674,#11672,#375,.T.);
#14553=EDGE_CURVE('',#11675,#11673,#376,.T.);
#14554=EDGE_CURVE('',#11676,#11677,#7364,.T.);
#14555=EDGE_CURVE('',#11676,#11674,#377,.T.);
#14556=EDGE_CURVE('',#11677,#11675,#378,.T.);
#14557=EDGE_CURVE('',#11678,#11679,#7365,.T.);
#14558=EDGE_CURVE('',#11678,#11676,#379,.T.);
#14559=EDGE_CURVE('',#11679,#11677,#380,.T.);
#14560=EDGE_CURVE('',#11680,#11681,#7366,.T.);
#14561=EDGE_CURVE('',#11680,#11678,#381,.T.);
#14562=EDGE_CURVE('',#11681,#11679,#382,.T.);
#14563=EDGE_CURVE('',#11682,#11683,#7367,.T.);
#14564=EDGE_CURVE('',#11682,#11680,#383,.T.);
#14565=EDGE_CURVE('',#11683,#11681,#384,.T.);
#14566=EDGE_CURVE('',#11684,#11685,#7368,.T.);
#14567=EDGE_CURVE('',#11684,#11682,#385,.T.);
#14568=EDGE_CURVE('',#11685,#11683,#386,.T.);
#14569=EDGE_CURVE('',#11686,#11687,#7369,.T.);
#14570=EDGE_CURVE('',#11686,#11684,#387,.T.);
#14571=EDGE_CURVE('',#11687,#11685,#388,.T.);
#14572=EDGE_CURVE('',#11688,#11689,#7370,.T.);
#14573=EDGE_CURVE('',#11688,#11686,#389,.T.);
#14574=EDGE_CURVE('',#11689,#11687,#390,.T.);
#14575=EDGE_CURVE('',#11690,#11691,#7371,.T.);
#14576=EDGE_CURVE('',#11690,#11688,#391,.T.);
#14577=EDGE_CURVE('',#11691,#11689,#392,.T.);
#14578=EDGE_CURVE('',#11692,#11693,#7372,.T.);
#14579=EDGE_CURVE('',#11692,#11690,#393,.T.);
#14580=EDGE_CURVE('',#11693,#11691,#394,.T.);
#14581=EDGE_CURVE('',#11694,#11695,#7373,.T.);
#14582=EDGE_CURVE('',#11694,#11692,#395,.T.);
#14583=EDGE_CURVE('',#11695,#11693,#396,.T.);
#14584=EDGE_CURVE('',#11696,#11697,#7374,.T.);
#14585=EDGE_CURVE('',#11696,#11694,#397,.T.);
#14586=EDGE_CURVE('',#11697,#11695,#398,.T.);
#14587=EDGE_CURVE('',#11698,#11699,#7375,.T.);
#14588=EDGE_CURVE('',#11698,#11696,#399,.T.);
#14589=EDGE_CURVE('',#11699,#11697,#400,.T.);
#14590=EDGE_CURVE('',#11700,#11701,#7376,.T.);
#14591=EDGE_CURVE('',#11700,#11698,#401,.T.);
#14592=EDGE_CURVE('',#11701,#11699,#402,.T.);
#14593=EDGE_CURVE('',#11702,#11703,#7377,.T.);
#14594=EDGE_CURVE('',#11702,#11700,#403,.T.);
#14595=EDGE_CURVE('',#11703,#11701,#404,.T.);
#14596=EDGE_CURVE('',#11704,#11705,#7378,.T.);
#14597=EDGE_CURVE('',#11704,#11702,#405,.T.);
#14598=EDGE_CURVE('',#11705,#11703,#406,.T.);
#14599=EDGE_CURVE('',#11706,#11706,#5985,.T.);
#14600=EDGE_CURVE('',#11706,#11707,#7379,.T.);
#14601=EDGE_CURVE('',#11707,#11708,#5986,.T.);
#14602=EDGE_CURVE('',#11708,#11707,#5987,.T.);
#14603=EDGE_CURVE('',#11708,#11709,#7380,.T.);
#14604=EDGE_CURVE('',#11710,#11709,#5988,.T.);
#14605=EDGE_CURVE('',#11711,#11710,#5989,.T.);
#14606=EDGE_CURVE('',#11709,#11711,#5990,.T.);
#14607=EDGE_CURVE('',#11712,#11712,#5991,.T.);
#14608=EDGE_CURVE('',#11712,#11713,#7381,.T.);
#14609=EDGE_CURVE('',#11713,#11713,#5992,.T.);
#14610=EDGE_CURVE('',#11714,#11714,#5993,.T.);
#14611=EDGE_CURVE('',#11714,#11713,#7382,.T.);
#14612=EDGE_CURVE('',#11715,#11715,#5994,.T.);
#14613=EDGE_CURVE('',#11716,#11710,#407,.T.);
#14614=EDGE_CURVE('',#11711,#11717,#408,.T.);
#14615=EDGE_CURVE('',#11717,#11716,#5995,.T.);
#14616=EDGE_CURVE('',#11711,#11718,#409,.T.);
#14617=EDGE_CURVE('',#11622,#11718,#410,.T.);
#14618=EDGE_CURVE('',#11719,#11704,#411,.T.);
#14619=EDGE_CURVE('',#11536,#11719,#412,.T.);
#14620=EDGE_CURVE('',#11717,#11618,#413,.T.);
#14621=EDGE_CURVE('',#11710,#11720,#414,.F.);
#14622=EDGE_CURVE('',#11720,#11718,#5996,.T.);
#14623=EDGE_CURVE('',#11720,#11623,#415,.T.);
#14624=EDGE_CURVE('',#11619,#11716,#416,.T.);
#14625=EDGE_CURVE('',#11721,#11537,#417,.T.);
#14626=EDGE_CURVE('',#11721,#11705,#418,.T.);
#14627=EDGE_CURVE('',#11719,#11721,#5997,.T.);
#14628=EDGE_CURVE('',#11722,#11714,#7383,.T.);
#14629=EDGE_CURVE('',#11723,#11724,#7384,.T.);
#14630=EDGE_CURVE('',#11725,#11723,#7385,.T.);
#14631=EDGE_CURVE('',#11726,#11725,#7386,.T.);
#14632=EDGE_CURVE('',#11726,#11724,#7387,.T.);
#14633=EDGE_CURVE('',#11724,#11727,#419,.T.);
#14634=EDGE_CURVE('',#11728,#11726,#5998,.T.);
#14635=EDGE_CURVE('',#11728,#11727,#7388,.T.);
#14636=EDGE_CURVE('',#11727,#11729,#7389,.T.);
#14637=EDGE_CURVE('',#11730,#11728,#7390,.T.);
#14638=EDGE_CURVE('',#11730,#11729,#7391,.T.);
#14639=EDGE_CURVE('',#11729,#11723,#420,.T.);
#14640=EDGE_CURVE('',#11725,#11730,#5999,.T.);
#14641=EDGE_CURVE('',#11731,#11731,#6000,.T.);
#14642=EDGE_CURVE('',#11731,#11715,#7392,.T.);
#14643=EDGE_CURVE('',#11732,#11732,#6001,.T.);
#14644=EDGE_CURVE('',#11732,#11731,#7393,.T.);
#14645=EDGE_CURVE('',#11733,#11733,#6002,.T.);
#14646=EDGE_CURVE('',#11734,#11734,#6003,.T.);
#14647=EDGE_CURVE('',#11734,#11733,#7394,.T.);
#14648=EDGE_CURVE('',#11735,#11735,#6004,.T.);
#14649=EDGE_CURVE('',#11735,#11734,#7395,.T.);
#14650=EDGE_CURVE('',#11736,#11736,#6005,.T.);
#14651=EDGE_CURVE('',#11736,#11735,#7396,.T.);
#19245=ORIENTED_EDGE('',*,*,#14345,.F.);
#19246=ORIENTED_EDGE('',*,*,#14346,.T.);
#19247=ORIENTED_EDGE('',*,*,#14347,.T.);
#19248=ORIENTED_EDGE('',*,*,#14348,.T.);
#19249=ORIENTED_EDGE('',*,*,#14349,.F.);
#19250=ORIENTED_EDGE('',*,*,#14350,.T.);
#19251=ORIENTED_EDGE('',*,*,#14345,.T.);
#19252=ORIENTED_EDGE('',*,*,#14351,.T.);
#19253=ORIENTED_EDGE('',*,*,#14352,.F.);
#19254=ORIENTED_EDGE('',*,*,#14353,.T.);
#19255=ORIENTED_EDGE('',*,*,#14349,.T.);
#19256=ORIENTED_EDGE('',*,*,#14354,.T.);
#19257=ORIENTED_EDGE('',*,*,#14355,.F.);
#19258=ORIENTED_EDGE('',*,*,#14356,.T.);
#19259=ORIENTED_EDGE('',*,*,#14352,.T.);
#19260=ORIENTED_EDGE('',*,*,#14357,.T.);
#19261=ORIENTED_EDGE('',*,*,#14358,.F.);
#19262=ORIENTED_EDGE('',*,*,#14359,.T.);
#19263=ORIENTED_EDGE('',*,*,#14355,.T.);
#19264=ORIENTED_EDGE('',*,*,#14360,.T.);
#19265=ORIENTED_EDGE('',*,*,#14361,.F.);
#19266=ORIENTED_EDGE('',*,*,#14362,.T.);
#19267=ORIENTED_EDGE('',*,*,#14358,.T.);
#19268=ORIENTED_EDGE('',*,*,#14363,.T.);
#19269=ORIENTED_EDGE('',*,*,#14364,.F.);
#19270=ORIENTED_EDGE('',*,*,#14365,.T.);
#19271=ORIENTED_EDGE('',*,*,#14361,.T.);
#19272=ORIENTED_EDGE('',*,*,#14366,.T.);
#19273=ORIENTED_EDGE('',*,*,#14367,.F.);
#19274=ORIENTED_EDGE('',*,*,#14368,.T.);
#19275=ORIENTED_EDGE('',*,*,#14364,.T.);
#19276=ORIENTED_EDGE('',*,*,#14369,.T.);
#19277=ORIENTED_EDGE('',*,*,#14370,.F.);
#19278=ORIENTED_EDGE('',*,*,#14371,.T.);
#19279=ORIENTED_EDGE('',*,*,#14367,.T.);
#19280=ORIENTED_EDGE('',*,*,#14372,.T.);
#19281=ORIENTED_EDGE('',*,*,#14373,.F.);
#19282=ORIENTED_EDGE('',*,*,#14374,.T.);
#19283=ORIENTED_EDGE('',*,*,#14370,.T.);
#19284=ORIENTED_EDGE('',*,*,#14375,.T.);
#19285=ORIENTED_EDGE('',*,*,#14376,.F.);
#19286=ORIENTED_EDGE('',*,*,#14377,.T.);
#19287=ORIENTED_EDGE('',*,*,#14373,.T.);
#19288=ORIENTED_EDGE('',*,*,#14378,.T.);
#19289=ORIENTED_EDGE('',*,*,#14379,.F.);
#19290=ORIENTED_EDGE('',*,*,#14380,.T.);
#19291=ORIENTED_EDGE('',*,*,#14376,.T.);
#19292=ORIENTED_EDGE('',*,*,#14381,.T.);
#19293=ORIENTED_EDGE('',*,*,#14382,.F.);
#19294=ORIENTED_EDGE('',*,*,#14383,.T.);
#19295=ORIENTED_EDGE('',*,*,#14379,.T.);
#19296=ORIENTED_EDGE('',*,*,#14384,.T.);
#19297=ORIENTED_EDGE('',*,*,#14385,.F.);
#19298=ORIENTED_EDGE('',*,*,#14386,.T.);
#19299=ORIENTED_EDGE('',*,*,#14382,.T.);
#19300=ORIENTED_EDGE('',*,*,#14387,.T.);
#19301=ORIENTED_EDGE('',*,*,#14388,.F.);
#19302=ORIENTED_EDGE('',*,*,#14389,.T.);
#19303=ORIENTED_EDGE('',*,*,#14385,.T.);
#19304=ORIENTED_EDGE('',*,*,#14390,.T.);
#19305=ORIENTED_EDGE('',*,*,#14391,.F.);
#19306=ORIENTED_EDGE('',*,*,#14392,.T.);
#19307=ORIENTED_EDGE('',*,*,#14388,.T.);
#19308=ORIENTED_EDGE('',*,*,#14393,.T.);
#19309=ORIENTED_EDGE('',*,*,#14394,.F.);
#19310=ORIENTED_EDGE('',*,*,#14395,.T.);
#19311=ORIENTED_EDGE('',*,*,#14391,.T.);
#19312=ORIENTED_EDGE('',*,*,#14396,.T.);
#19313=ORIENTED_EDGE('',*,*,#14397,.F.);
#19314=ORIENTED_EDGE('',*,*,#14398,.T.);
#19315=ORIENTED_EDGE('',*,*,#14394,.T.);
#19316=ORIENTED_EDGE('',*,*,#14399,.T.);
#19317=ORIENTED_EDGE('',*,*,#14400,.F.);
#19318=ORIENTED_EDGE('',*,*,#14401,.T.);
#19319=ORIENTED_EDGE('',*,*,#14397,.T.);
#19320=ORIENTED_EDGE('',*,*,#14402,.T.);
#19321=ORIENTED_EDGE('',*,*,#14403,.F.);
#19322=ORIENTED_EDGE('',*,*,#14404,.T.);
#19323=ORIENTED_EDGE('',*,*,#14400,.T.);
#19324=ORIENTED_EDGE('',*,*,#14405,.T.);
#19325=ORIENTED_EDGE('',*,*,#14406,.F.);
#19326=ORIENTED_EDGE('',*,*,#14407,.T.);
#19327=ORIENTED_EDGE('',*,*,#14403,.T.);
#19328=ORIENTED_EDGE('',*,*,#14408,.T.);
#19329=ORIENTED_EDGE('',*,*,#14409,.F.);
#19330=ORIENTED_EDGE('',*,*,#14410,.T.);
#19331=ORIENTED_EDGE('',*,*,#14406,.T.);
#19332=ORIENTED_EDGE('',*,*,#14411,.T.);
#19333=ORIENTED_EDGE('',*,*,#14412,.F.);
#19334=ORIENTED_EDGE('',*,*,#14413,.T.);
#19335=ORIENTED_EDGE('',*,*,#14409,.T.);
#19336=ORIENTED_EDGE('',*,*,#14414,.T.);
#19337=ORIENTED_EDGE('',*,*,#14415,.F.);
#19338=ORIENTED_EDGE('',*,*,#14416,.T.);
#19339=ORIENTED_EDGE('',*,*,#14412,.T.);
#19340=ORIENTED_EDGE('',*,*,#14417,.T.);
#19341=ORIENTED_EDGE('',*,*,#14418,.F.);
#19342=ORIENTED_EDGE('',*,*,#14419,.T.);
#19343=ORIENTED_EDGE('',*,*,#14415,.T.);
#19344=ORIENTED_EDGE('',*,*,#14420,.T.);
#19345=ORIENTED_EDGE('',*,*,#14421,.F.);
#19346=ORIENTED_EDGE('',*,*,#14422,.T.);
#19347=ORIENTED_EDGE('',*,*,#14418,.T.);
#19348=ORIENTED_EDGE('',*,*,#14423,.T.);
#19349=ORIENTED_EDGE('',*,*,#14424,.F.);
#19350=ORIENTED_EDGE('',*,*,#14425,.T.);
#19351=ORIENTED_EDGE('',*,*,#14421,.T.);
#19352=ORIENTED_EDGE('',*,*,#14426,.T.);
#19353=ORIENTED_EDGE('',*,*,#14427,.F.);
#19354=ORIENTED_EDGE('',*,*,#14428,.T.);
#19355=ORIENTED_EDGE('',*,*,#14424,.T.);
#19356=ORIENTED_EDGE('',*,*,#14429,.T.);
#19357=ORIENTED_EDGE('',*,*,#14430,.F.);
#19358=ORIENTED_EDGE('',*,*,#14431,.T.);
#19359=ORIENTED_EDGE('',*,*,#14427,.T.);
#19360=ORIENTED_EDGE('',*,*,#14432,.T.);
#19361=ORIENTED_EDGE('',*,*,#14433,.F.);
#19362=ORIENTED_EDGE('',*,*,#14434,.T.);
#19363=ORIENTED_EDGE('',*,*,#14430,.T.);
#19364=ORIENTED_EDGE('',*,*,#14435,.T.);
#19365=ORIENTED_EDGE('',*,*,#14436,.F.);
#19366=ORIENTED_EDGE('',*,*,#14437,.T.);
#19367=ORIENTED_EDGE('',*,*,#14433,.T.);
#19368=ORIENTED_EDGE('',*,*,#14438,.T.);
#19369=ORIENTED_EDGE('',*,*,#14439,.F.);
#19370=ORIENTED_EDGE('',*,*,#14440,.T.);
#19371=ORIENTED_EDGE('',*,*,#14436,.T.);
#19372=ORIENTED_EDGE('',*,*,#14441,.T.);
#19373=ORIENTED_EDGE('',*,*,#14442,.F.);
#19374=ORIENTED_EDGE('',*,*,#14443,.T.);
#19375=ORIENTED_EDGE('',*,*,#14439,.T.);
#19376=ORIENTED_EDGE('',*,*,#14444,.T.);
#19377=ORIENTED_EDGE('',*,*,#14445,.F.);
#19378=ORIENTED_EDGE('',*,*,#14446,.T.);
#19379=ORIENTED_EDGE('',*,*,#14442,.T.);
#19380=ORIENTED_EDGE('',*,*,#14447,.T.);
#19381=ORIENTED_EDGE('',*,*,#14448,.F.);
#19382=ORIENTED_EDGE('',*,*,#14449,.T.);
#19383=ORIENTED_EDGE('',*,*,#14445,.T.);
#19384=ORIENTED_EDGE('',*,*,#14450,.T.);
#19385=ORIENTED_EDGE('',*,*,#14451,.F.);
#19386=ORIENTED_EDGE('',*,*,#14452,.T.);
#19387=ORIENTED_EDGE('',*,*,#14448,.T.);
#19388=ORIENTED_EDGE('',*,*,#14453,.T.);
#19389=ORIENTED_EDGE('',*,*,#14454,.F.);
#19390=ORIENTED_EDGE('',*,*,#14455,.T.);
#19391=ORIENTED_EDGE('',*,*,#14451,.T.);
#19392=ORIENTED_EDGE('',*,*,#14456,.T.);
#19393=ORIENTED_EDGE('',*,*,#14457,.F.);
#19394=ORIENTED_EDGE('',*,*,#14458,.T.);
#19395=ORIENTED_EDGE('',*,*,#14454,.T.);
#19396=ORIENTED_EDGE('',*,*,#14459,.T.);
#19397=ORIENTED_EDGE('',*,*,#14460,.F.);
#19398=ORIENTED_EDGE('',*,*,#14461,.T.);
#19399=ORIENTED_EDGE('',*,*,#14457,.T.);
#19400=ORIENTED_EDGE('',*,*,#14462,.T.);
#19401=ORIENTED_EDGE('',*,*,#14463,.F.);
#19402=ORIENTED_EDGE('',*,*,#14464,.T.);
#19403=ORIENTED_EDGE('',*,*,#14460,.T.);
#19404=ORIENTED_EDGE('',*,*,#14465,.T.);
#19405=ORIENTED_EDGE('',*,*,#14466,.F.);
#19406=ORIENTED_EDGE('',*,*,#14467,.T.);
#19407=ORIENTED_EDGE('',*,*,#14463,.T.);
#19408=ORIENTED_EDGE('',*,*,#14468,.T.);
#19409=ORIENTED_EDGE('',*,*,#14469,.F.);
#19410=ORIENTED_EDGE('',*,*,#14470,.T.);
#19411=ORIENTED_EDGE('',*,*,#14466,.T.);
#19412=ORIENTED_EDGE('',*,*,#14471,.T.);
#19413=ORIENTED_EDGE('',*,*,#14472,.F.);
#19414=ORIENTED_EDGE('',*,*,#14473,.T.);
#19415=ORIENTED_EDGE('',*,*,#14474,.F.);
#19416=ORIENTED_EDGE('',*,*,#14475,.F.);
#19417=ORIENTED_EDGE('',*,*,#14476,.F.);
#19418=ORIENTED_EDGE('',*,*,#14477,.T.);
#19419=ORIENTED_EDGE('',*,*,#14472,.T.);
#19420=ORIENTED_EDGE('',*,*,#14478,.F.);
#19421=ORIENTED_EDGE('',*,*,#14479,.F.);
#19422=ORIENTED_EDGE('',*,*,#14480,.T.);
#19423=ORIENTED_EDGE('',*,*,#14476,.T.);
#19424=ORIENTED_EDGE('',*,*,#14481,.F.);
#19425=ORIENTED_EDGE('',*,*,#14482,.F.);
#19426=ORIENTED_EDGE('',*,*,#14483,.T.);
#19427=ORIENTED_EDGE('',*,*,#14479,.T.);
#19428=ORIENTED_EDGE('',*,*,#14484,.F.);
#19429=ORIENTED_EDGE('',*,*,#14485,.F.);
#19430=ORIENTED_EDGE('',*,*,#14486,.T.);
#19431=ORIENTED_EDGE('',*,*,#14482,.T.);
#19432=ORIENTED_EDGE('',*,*,#14487,.F.);
#19433=ORIENTED_EDGE('',*,*,#14488,.F.);
#19434=ORIENTED_EDGE('',*,*,#14489,.T.);
#19435=ORIENTED_EDGE('',*,*,#14485,.T.);
#19436=ORIENTED_EDGE('',*,*,#14490,.F.);
#19437=ORIENTED_EDGE('',*,*,#14491,.F.);
#19438=ORIENTED_EDGE('',*,*,#14492,.T.);
#19439=ORIENTED_EDGE('',*,*,#14488,.T.);
#19440=ORIENTED_EDGE('',*,*,#14493,.F.);
#19441=ORIENTED_EDGE('',*,*,#14494,.F.);
#19442=ORIENTED_EDGE('',*,*,#14495,.T.);
#19443=ORIENTED_EDGE('',*,*,#14491,.T.);
#19444=ORIENTED_EDGE('',*,*,#14496,.F.);
#19445=ORIENTED_EDGE('',*,*,#14497,.F.);
#19446=ORIENTED_EDGE('',*,*,#14498,.T.);
#19447=ORIENTED_EDGE('',*,*,#14494,.T.);
#19448=ORIENTED_EDGE('',*,*,#14499,.F.);
#19449=ORIENTED_EDGE('',*,*,#14500,.F.);
#19450=ORIENTED_EDGE('',*,*,#14501,.T.);
#19451=ORIENTED_EDGE('',*,*,#14497,.T.);
#19452=ORIENTED_EDGE('',*,*,#14502,.F.);
#19453=ORIENTED_EDGE('',*,*,#14503,.F.);
#19454=ORIENTED_EDGE('',*,*,#14504,.T.);
#19455=ORIENTED_EDGE('',*,*,#14500,.T.);
#19456=ORIENTED_EDGE('',*,*,#14505,.F.);
#19457=ORIENTED_EDGE('',*,*,#14506,.F.);
#19458=ORIENTED_EDGE('',*,*,#14507,.T.);
#19459=ORIENTED_EDGE('',*,*,#14503,.T.);
#19460=ORIENTED_EDGE('',*,*,#14508,.F.);
#19461=ORIENTED_EDGE('',*,*,#14509,.F.);
#19462=ORIENTED_EDGE('',*,*,#14510,.T.);
#19463=ORIENTED_EDGE('',*,*,#14506,.T.);
#19464=ORIENTED_EDGE('',*,*,#14511,.F.);
#19465=ORIENTED_EDGE('',*,*,#14512,.F.);
#19466=ORIENTED_EDGE('',*,*,#14513,.T.);
#19467=ORIENTED_EDGE('',*,*,#14509,.T.);
#19468=ORIENTED_EDGE('',*,*,#14514,.F.);
#19469=ORIENTED_EDGE('',*,*,#14515,.F.);
#19470=ORIENTED_EDGE('',*,*,#14516,.T.);
#19471=ORIENTED_EDGE('',*,*,#14512,.T.);
#19472=ORIENTED_EDGE('',*,*,#14517,.F.);
#19473=ORIENTED_EDGE('',*,*,#14518,.F.);
#19474=ORIENTED_EDGE('',*,*,#14519,.T.);
#19475=ORIENTED_EDGE('',*,*,#14515,.T.);
#19476=ORIENTED_EDGE('',*,*,#14520,.F.);
#19477=ORIENTED_EDGE('',*,*,#14521,.F.);
#19478=ORIENTED_EDGE('',*,*,#14522,.T.);
#19479=ORIENTED_EDGE('',*,*,#14518,.T.);
#19480=ORIENTED_EDGE('',*,*,#14523,.F.);
#19481=ORIENTED_EDGE('',*,*,#14524,.F.);
#19482=ORIENTED_EDGE('',*,*,#14525,.T.);
#19483=ORIENTED_EDGE('',*,*,#14521,.T.);
#19484=ORIENTED_EDGE('',*,*,#14526,.F.);
#19485=ORIENTED_EDGE('',*,*,#14527,.F.);
#19486=ORIENTED_EDGE('',*,*,#14528,.T.);
#19487=ORIENTED_EDGE('',*,*,#14524,.T.);
#19488=ORIENTED_EDGE('',*,*,#14529,.F.);
#19489=ORIENTED_EDGE('',*,*,#14530,.F.);
#19490=ORIENTED_EDGE('',*,*,#14531,.T.);
#19491=ORIENTED_EDGE('',*,*,#14527,.T.);
#19492=ORIENTED_EDGE('',*,*,#14532,.F.);
#19493=ORIENTED_EDGE('',*,*,#14533,.F.);
#19494=ORIENTED_EDGE('',*,*,#14534,.T.);
#19495=ORIENTED_EDGE('',*,*,#14530,.T.);
#19496=ORIENTED_EDGE('',*,*,#14535,.F.);
#19497=ORIENTED_EDGE('',*,*,#14536,.F.);
#19498=ORIENTED_EDGE('',*,*,#14537,.T.);
#19499=ORIENTED_EDGE('',*,*,#14533,.T.);
#19500=ORIENTED_EDGE('',*,*,#14538,.F.);
#19501=ORIENTED_EDGE('',*,*,#14539,.F.);
#19502=ORIENTED_EDGE('',*,*,#14540,.T.);
#19503=ORIENTED_EDGE('',*,*,#14536,.T.);
#19504=ORIENTED_EDGE('',*,*,#14541,.F.);
#19505=ORIENTED_EDGE('',*,*,#14542,.F.);
#19506=ORIENTED_EDGE('',*,*,#14543,.T.);
#19507=ORIENTED_EDGE('',*,*,#14539,.T.);
#19508=ORIENTED_EDGE('',*,*,#14544,.F.);
#19509=ORIENTED_EDGE('',*,*,#14545,.F.);
#19510=ORIENTED_EDGE('',*,*,#14546,.T.);
#19511=ORIENTED_EDGE('',*,*,#14542,.T.);
#19512=ORIENTED_EDGE('',*,*,#14547,.F.);
#19513=ORIENTED_EDGE('',*,*,#14548,.F.);
#19514=ORIENTED_EDGE('',*,*,#14549,.T.);
#19515=ORIENTED_EDGE('',*,*,#14545,.T.);
#19516=ORIENTED_EDGE('',*,*,#14550,.F.);
#19517=ORIENTED_EDGE('',*,*,#14551,.F.);
#19518=ORIENTED_EDGE('',*,*,#14552,.T.);
#19519=ORIENTED_EDGE('',*,*,#14548,.T.);
#19520=ORIENTED_EDGE('',*,*,#14553,.F.);
#19521=ORIENTED_EDGE('',*,*,#14554,.F.);
#19522=ORIENTED_EDGE('',*,*,#14555,.T.);
#19523=ORIENTED_EDGE('',*,*,#14551,.T.);
#19524=ORIENTED_EDGE('',*,*,#14556,.F.);
#19525=ORIENTED_EDGE('',*,*,#14557,.F.);
#19526=ORIENTED_EDGE('',*,*,#14558,.T.);
#19527=ORIENTED_EDGE('',*,*,#14554,.T.);
#19528=ORIENTED_EDGE('',*,*,#14559,.F.);
#19529=ORIENTED_EDGE('',*,*,#14560,.F.);
#19530=ORIENTED_EDGE('',*,*,#14561,.T.);
#19531=ORIENTED_EDGE('',*,*,#14557,.T.);
#19532=ORIENTED_EDGE('',*,*,#14562,.F.);
#19533=ORIENTED_EDGE('',*,*,#14563,.F.);
#19534=ORIENTED_EDGE('',*,*,#14564,.T.);
#19535=ORIENTED_EDGE('',*,*,#14560,.T.);
#19536=ORIENTED_EDGE('',*,*,#14565,.F.);
#19537=ORIENTED_EDGE('',*,*,#14566,.F.);
#19538=ORIENTED_EDGE('',*,*,#14567,.T.);
#19539=ORIENTED_EDGE('',*,*,#14563,.T.);
#19540=ORIENTED_EDGE('',*,*,#14568,.F.);
#19541=ORIENTED_EDGE('',*,*,#14569,.F.);
#19542=ORIENTED_EDGE('',*,*,#14570,.T.);
#19543=ORIENTED_EDGE('',*,*,#14566,.T.);
#19544=ORIENTED_EDGE('',*,*,#14571,.F.);
#19545=ORIENTED_EDGE('',*,*,#14572,.F.);
#19546=ORIENTED_EDGE('',*,*,#14573,.T.);
#19547=ORIENTED_EDGE('',*,*,#14569,.T.);
#19548=ORIENTED_EDGE('',*,*,#14574,.F.);
#19549=ORIENTED_EDGE('',*,*,#14575,.F.);
#19550=ORIENTED_EDGE('',*,*,#14576,.T.);
#19551=ORIENTED_EDGE('',*,*,#14572,.T.);
#19552=ORIENTED_EDGE('',*,*,#14577,.F.);
#19553=ORIENTED_EDGE('',*,*,#14578,.F.);
#19554=ORIENTED_EDGE('',*,*,#14579,.T.);
#19555=ORIENTED_EDGE('',*,*,#14575,.T.);
#19556=ORIENTED_EDGE('',*,*,#14580,.F.);
#19557=ORIENTED_EDGE('',*,*,#14581,.F.);
#19558=ORIENTED_EDGE('',*,*,#14582,.T.);
#19559=ORIENTED_EDGE('',*,*,#14578,.T.);
#19560=ORIENTED_EDGE('',*,*,#14583,.F.);
#19561=ORIENTED_EDGE('',*,*,#14584,.F.);
#19562=ORIENTED_EDGE('',*,*,#14585,.T.);
#19563=ORIENTED_EDGE('',*,*,#14581,.T.);
#19564=ORIENTED_EDGE('',*,*,#14586,.F.);
#19565=ORIENTED_EDGE('',*,*,#14587,.F.);
#19566=ORIENTED_EDGE('',*,*,#14588,.T.);
#19567=ORIENTED_EDGE('',*,*,#14584,.T.);
#19568=ORIENTED_EDGE('',*,*,#14589,.F.);
#19569=ORIENTED_EDGE('',*,*,#14590,.F.);
#19570=ORIENTED_EDGE('',*,*,#14591,.T.);
#19571=ORIENTED_EDGE('',*,*,#14587,.T.);
#19572=ORIENTED_EDGE('',*,*,#14592,.F.);
#19573=ORIENTED_EDGE('',*,*,#14593,.F.);
#19574=ORIENTED_EDGE('',*,*,#14594,.T.);
#19575=ORIENTED_EDGE('',*,*,#14590,.T.);
#19576=ORIENTED_EDGE('',*,*,#14595,.F.);
#19577=ORIENTED_EDGE('',*,*,#14596,.F.);
#19578=ORIENTED_EDGE('',*,*,#14597,.T.);
#19579=ORIENTED_EDGE('',*,*,#14593,.T.);
#19580=ORIENTED_EDGE('',*,*,#14598,.F.);
#19581=ORIENTED_EDGE('',*,*,#14599,.T.);
#19582=ORIENTED_EDGE('',*,*,#14600,.T.);
#19583=ORIENTED_EDGE('',*,*,#14601,.T.);
#19584=ORIENTED_EDGE('',*,*,#14602,.T.);
#19585=ORIENTED_EDGE('',*,*,#14600,.F.);
#19586=ORIENTED_EDGE('',*,*,#14601,.F.);
#19587=ORIENTED_EDGE('',*,*,#14602,.F.);
#19588=ORIENTED_EDGE('',*,*,#14603,.T.);
#19589=ORIENTED_EDGE('',*,*,#14604,.F.);
#19590=ORIENTED_EDGE('',*,*,#14605,.F.);
#19591=ORIENTED_EDGE('',*,*,#14606,.F.);
#19592=ORIENTED_EDGE('',*,*,#14603,.F.);
#19593=ORIENTED_EDGE('',*,*,#14599,.F.);
#19594=ORIENTED_EDGE('',*,*,#14607,.T.);
#19595=ORIENTED_EDGE('',*,*,#14608,.T.);
#19596=ORIENTED_EDGE('',*,*,#14609,.T.);
#19597=ORIENTED_EDGE('',*,*,#14608,.F.);
#19598=ORIENTED_EDGE('',*,*,#14610,.F.);
#19599=ORIENTED_EDGE('',*,*,#14611,.T.);
#19600=ORIENTED_EDGE('',*,*,#14609,.F.);
#19601=ORIENTED_EDGE('',*,*,#14611,.F.);
#19602=ORIENTED_EDGE('',*,*,#14612,.F.);
#19603=ORIENTED_EDGE('',*,*,#14607,.F.);
#19604=ORIENTED_EDGE('',*,*,#14613,.T.);
#19605=ORIENTED_EDGE('',*,*,#14604,.T.);
#19606=ORIENTED_EDGE('',*,*,#14606,.T.);
#19607=ORIENTED_EDGE('',*,*,#14614,.T.);
#19608=ORIENTED_EDGE('',*,*,#14615,.T.);
#19609=ORIENTED_EDGE('',*,*,#14614,.F.);
#19610=ORIENTED_EDGE('',*,*,#14616,.T.);
#19611=ORIENTED_EDGE('',*,*,#14617,.F.);
#19612=ORIENTED_EDGE('',*,*,#14473,.F.);
#19613=ORIENTED_EDGE('',*,*,#14477,.F.);
#19614=ORIENTED_EDGE('',*,*,#14480,.F.);
#19615=ORIENTED_EDGE('',*,*,#14483,.F.);
#19616=ORIENTED_EDGE('',*,*,#14486,.F.);
#19617=ORIENTED_EDGE('',*,*,#14489,.F.);
#19618=ORIENTED_EDGE('',*,*,#14492,.F.);
#19619=ORIENTED_EDGE('',*,*,#14495,.F.);
#19620=ORIENTED_EDGE('',*,*,#14498,.F.);
#19621=ORIENTED_EDGE('',*,*,#14501,.F.);
#19622=ORIENTED_EDGE('',*,*,#14504,.F.);
#19623=ORIENTED_EDGE('',*,*,#14507,.F.);
#19624=ORIENTED_EDGE('',*,*,#14510,.F.);
#19625=ORIENTED_EDGE('',*,*,#14513,.F.);
#19626=ORIENTED_EDGE('',*,*,#14516,.F.);
#19627=ORIENTED_EDGE('',*,*,#14519,.F.);
#19628=ORIENTED_EDGE('',*,*,#14522,.F.);
#19629=ORIENTED_EDGE('',*,*,#14525,.F.);
#19630=ORIENTED_EDGE('',*,*,#14528,.F.);
#19631=ORIENTED_EDGE('',*,*,#14531,.F.);
#19632=ORIENTED_EDGE('',*,*,#14534,.F.);
#19633=ORIENTED_EDGE('',*,*,#14537,.F.);
#19634=ORIENTED_EDGE('',*,*,#14540,.F.);
#19635=ORIENTED_EDGE('',*,*,#14543,.F.);
#19636=ORIENTED_EDGE('',*,*,#14546,.F.);
#19637=ORIENTED_EDGE('',*,*,#14549,.F.);
#19638=ORIENTED_EDGE('',*,*,#14552,.F.);
#19639=ORIENTED_EDGE('',*,*,#14555,.F.);
#19640=ORIENTED_EDGE('',*,*,#14558,.F.);
#19641=ORIENTED_EDGE('',*,*,#14561,.F.);
#19642=ORIENTED_EDGE('',*,*,#14564,.F.);
#19643=ORIENTED_EDGE('',*,*,#14567,.F.);
#19644=ORIENTED_EDGE('',*,*,#14570,.F.);
#19645=ORIENTED_EDGE('',*,*,#14573,.F.);
#19646=ORIENTED_EDGE('',*,*,#14576,.F.);
#19647=ORIENTED_EDGE('',*,*,#14579,.F.);
#19648=ORIENTED_EDGE('',*,*,#14582,.F.);
#19649=ORIENTED_EDGE('',*,*,#14585,.F.);
#19650=ORIENTED_EDGE('',*,*,#14588,.F.);
#19651=ORIENTED_EDGE('',*,*,#14591,.F.);
#19652=ORIENTED_EDGE('',*,*,#14594,.F.);
#19653=ORIENTED_EDGE('',*,*,#14597,.F.);
#19654=ORIENTED_EDGE('',*,*,#14618,.F.);
#19655=ORIENTED_EDGE('',*,*,#14619,.F.);
#19656=ORIENTED_EDGE('',*,*,#14346,.F.);
#19657=ORIENTED_EDGE('',*,*,#14350,.F.);
#19658=ORIENTED_EDGE('',*,*,#14353,.F.);
#19659=ORIENTED_EDGE('',*,*,#14356,.F.);
#19660=ORIENTED_EDGE('',*,*,#14359,.F.);
#19661=ORIENTED_EDGE('',*,*,#14362,.F.);
#19662=ORIENTED_EDGE('',*,*,#14365,.F.);
#19663=ORIENTED_EDGE('',*,*,#14368,.F.);
#19664=ORIENTED_EDGE('',*,*,#14371,.F.);
#19665=ORIENTED_EDGE('',*,*,#14374,.F.);
#19666=ORIENTED_EDGE('',*,*,#14377,.F.);
#19667=ORIENTED_EDGE('',*,*,#14380,.F.);
#19668=ORIENTED_EDGE('',*,*,#14383,.F.);
#19669=ORIENTED_EDGE('',*,*,#14386,.F.);
#19670=ORIENTED_EDGE('',*,*,#14389,.F.);
#19671=ORIENTED_EDGE('',*,*,#14392,.F.);
#19672=ORIENTED_EDGE('',*,*,#14395,.F.);
#19673=ORIENTED_EDGE('',*,*,#14398,.F.);
#19674=ORIENTED_EDGE('',*,*,#14401,.F.);
#19675=ORIENTED_EDGE('',*,*,#14404,.F.);
#19676=ORIENTED_EDGE('',*,*,#14407,.F.);
#19677=ORIENTED_EDGE('',*,*,#14410,.F.);
#19678=ORIENTED_EDGE('',*,*,#14413,.F.);
#19679=ORIENTED_EDGE('',*,*,#14416,.F.);
#19680=ORIENTED_EDGE('',*,*,#14419,.F.);
#19681=ORIENTED_EDGE('',*,*,#14422,.F.);
#19682=ORIENTED_EDGE('',*,*,#14425,.F.);
#19683=ORIENTED_EDGE('',*,*,#14428,.F.);
#19684=ORIENTED_EDGE('',*,*,#14431,.F.);
#19685=ORIENTED_EDGE('',*,*,#14434,.F.);
#19686=ORIENTED_EDGE('',*,*,#14437,.F.);
#19687=ORIENTED_EDGE('',*,*,#14440,.F.);
#19688=ORIENTED_EDGE('',*,*,#14443,.F.);
#19689=ORIENTED_EDGE('',*,*,#14446,.F.);
#19690=ORIENTED_EDGE('',*,*,#14449,.F.);
#19691=ORIENTED_EDGE('',*,*,#14452,.F.);
#19692=ORIENTED_EDGE('',*,*,#14455,.F.);
#19693=ORIENTED_EDGE('',*,*,#14458,.F.);
#19694=ORIENTED_EDGE('',*,*,#14461,.F.);
#19695=ORIENTED_EDGE('',*,*,#14464,.F.);
#19696=ORIENTED_EDGE('',*,*,#14467,.F.);
#19697=ORIENTED_EDGE('',*,*,#14470,.F.);
#19698=ORIENTED_EDGE('',*,*,#14620,.F.);
#19699=ORIENTED_EDGE('',*,*,#14621,.T.);
#19700=ORIENTED_EDGE('',*,*,#14622,.T.);
#19701=ORIENTED_EDGE('',*,*,#14616,.F.);
#19702=ORIENTED_EDGE('',*,*,#14605,.T.);
#19703=ORIENTED_EDGE('',*,*,#14622,.F.);
#19704=ORIENTED_EDGE('',*,*,#14623,.T.);
#19705=ORIENTED_EDGE('',*,*,#14474,.T.);
#19706=ORIENTED_EDGE('',*,*,#14617,.T.);
#19707=ORIENTED_EDGE('',*,*,#14613,.F.);
#19708=ORIENTED_EDGE('',*,*,#14624,.F.);
#19709=ORIENTED_EDGE('',*,*,#14471,.F.);
#19710=ORIENTED_EDGE('',*,*,#14468,.F.);
#19711=ORIENTED_EDGE('',*,*,#14465,.F.);
#19712=ORIENTED_EDGE('',*,*,#14462,.F.);
#19713=ORIENTED_EDGE('',*,*,#14459,.F.);
#19714=ORIENTED_EDGE('',*,*,#14456,.F.);
#19715=ORIENTED_EDGE('',*,*,#14453,.F.);
#19716=ORIENTED_EDGE('',*,*,#14450,.F.);
#19717=ORIENTED_EDGE('',*,*,#14447,.F.);
#19718=ORIENTED_EDGE('',*,*,#14444,.F.);
#19719=ORIENTED_EDGE('',*,*,#14441,.F.);
#19720=ORIENTED_EDGE('',*,*,#14438,.F.);
#19721=ORIENTED_EDGE('',*,*,#14435,.F.);
#19722=ORIENTED_EDGE('',*,*,#14432,.F.);
#19723=ORIENTED_EDGE('',*,*,#14429,.F.);
#19724=ORIENTED_EDGE('',*,*,#14426,.F.);
#19725=ORIENTED_EDGE('',*,*,#14423,.F.);
#19726=ORIENTED_EDGE('',*,*,#14420,.F.);
#19727=ORIENTED_EDGE('',*,*,#14417,.F.);
#19728=ORIENTED_EDGE('',*,*,#14414,.F.);
#19729=ORIENTED_EDGE('',*,*,#14411,.F.);
#19730=ORIENTED_EDGE('',*,*,#14408,.F.);
#19731=ORIENTED_EDGE('',*,*,#14405,.F.);
#19732=ORIENTED_EDGE('',*,*,#14402,.F.);
#19733=ORIENTED_EDGE('',*,*,#14399,.F.);
#19734=ORIENTED_EDGE('',*,*,#14396,.F.);
#19735=ORIENTED_EDGE('',*,*,#14393,.F.);
#19736=ORIENTED_EDGE('',*,*,#14390,.F.);
#19737=ORIENTED_EDGE('',*,*,#14387,.F.);
#19738=ORIENTED_EDGE('',*,*,#14384,.F.);
#19739=ORIENTED_EDGE('',*,*,#14381,.F.);
#19740=ORIENTED_EDGE('',*,*,#14378,.F.);
#19741=ORIENTED_EDGE('',*,*,#14375,.F.);
#19742=ORIENTED_EDGE('',*,*,#14372,.F.);
#19743=ORIENTED_EDGE('',*,*,#14369,.F.);
#19744=ORIENTED_EDGE('',*,*,#14366,.F.);
#19745=ORIENTED_EDGE('',*,*,#14363,.F.);
#19746=ORIENTED_EDGE('',*,*,#14360,.F.);
#19747=ORIENTED_EDGE('',*,*,#14357,.F.);
#19748=ORIENTED_EDGE('',*,*,#14354,.F.);
#19749=ORIENTED_EDGE('',*,*,#14351,.F.);
#19750=ORIENTED_EDGE('',*,*,#14348,.F.);
#19751=ORIENTED_EDGE('',*,*,#14625,.F.);
#19752=ORIENTED_EDGE('',*,*,#14626,.T.);
#19753=ORIENTED_EDGE('',*,*,#14598,.T.);
#19754=ORIENTED_EDGE('',*,*,#14595,.T.);
#19755=ORIENTED_EDGE('',*,*,#14592,.T.);
#19756=ORIENTED_EDGE('',*,*,#14589,.T.);
#19757=ORIENTED_EDGE('',*,*,#14586,.T.);
#19758=ORIENTED_EDGE('',*,*,#14583,.T.);
#19759=ORIENTED_EDGE('',*,*,#14580,.T.);
#19760=ORIENTED_EDGE('',*,*,#14577,.T.);
#19761=ORIENTED_EDGE('',*,*,#14574,.T.);
#19762=ORIENTED_EDGE('',*,*,#14571,.T.);
#19763=ORIENTED_EDGE('',*,*,#14568,.T.);
#19764=ORIENTED_EDGE('',*,*,#14565,.T.);
#19765=ORIENTED_EDGE('',*,*,#14562,.T.);
#19766=ORIENTED_EDGE('',*,*,#14559,.T.);
#19767=ORIENTED_EDGE('',*,*,#14556,.T.);
#19768=ORIENTED_EDGE('',*,*,#14553,.T.);
#19769=ORIENTED_EDGE('',*,*,#14550,.T.);
#19770=ORIENTED_EDGE('',*,*,#14547,.T.);
#19771=ORIENTED_EDGE('',*,*,#14544,.T.);
#19772=ORIENTED_EDGE('',*,*,#14541,.T.);
#19773=ORIENTED_EDGE('',*,*,#14538,.T.);
#19774=ORIENTED_EDGE('',*,*,#14535,.T.);
#19775=ORIENTED_EDGE('',*,*,#14532,.T.);
#19776=ORIENTED_EDGE('',*,*,#14529,.T.);
#19777=ORIENTED_EDGE('',*,*,#14526,.T.);
#19778=ORIENTED_EDGE('',*,*,#14523,.T.);
#19779=ORIENTED_EDGE('',*,*,#14520,.T.);
#19780=ORIENTED_EDGE('',*,*,#14517,.T.);
#19781=ORIENTED_EDGE('',*,*,#14514,.T.);
#19782=ORIENTED_EDGE('',*,*,#14511,.T.);
#19783=ORIENTED_EDGE('',*,*,#14508,.T.);
#19784=ORIENTED_EDGE('',*,*,#14505,.T.);
#19785=ORIENTED_EDGE('',*,*,#14502,.T.);
#19786=ORIENTED_EDGE('',*,*,#14499,.T.);
#19787=ORIENTED_EDGE('',*,*,#14496,.T.);
#19788=ORIENTED_EDGE('',*,*,#14493,.T.);
#19789=ORIENTED_EDGE('',*,*,#14490,.T.);
#19790=ORIENTED_EDGE('',*,*,#14487,.T.);
#19791=ORIENTED_EDGE('',*,*,#14484,.T.);
#19792=ORIENTED_EDGE('',*,*,#14481,.T.);
#19793=ORIENTED_EDGE('',*,*,#14478,.T.);
#19794=ORIENTED_EDGE('',*,*,#14475,.T.);
#19795=ORIENTED_EDGE('',*,*,#14623,.F.);
#19796=ORIENTED_EDGE('',*,*,#14621,.F.);
#19797=ORIENTED_EDGE('',*,*,#14596,.T.);
#19798=ORIENTED_EDGE('',*,*,#14626,.F.);
#19799=ORIENTED_EDGE('',*,*,#14627,.F.);
#19800=ORIENTED_EDGE('',*,*,#14618,.T.);
#19801=ORIENTED_EDGE('',*,*,#14469,.T.);
#19802=ORIENTED_EDGE('',*,*,#14624,.T.);
#19803=ORIENTED_EDGE('',*,*,#14615,.F.);
#19804=ORIENTED_EDGE('',*,*,#14620,.T.);
#19805=ORIENTED_EDGE('',*,*,#14628,.T.);
#19806=ORIENTED_EDGE('',*,*,#14610,.T.);
#19807=ORIENTED_EDGE('',*,*,#14628,.F.);
#19808=ORIENTED_EDGE('',*,*,#14629,.F.);
#19809=ORIENTED_EDGE('',*,*,#14630,.F.);
#19810=ORIENTED_EDGE('',*,*,#14631,.F.);
#19811=ORIENTED_EDGE('',*,*,#14632,.T.);
#19812=ORIENTED_EDGE('',*,*,#14633,.F.);
#19813=ORIENTED_EDGE('',*,*,#14632,.F.);
#19814=ORIENTED_EDGE('',*,*,#14634,.F.);
#19815=ORIENTED_EDGE('',*,*,#14635,.T.);
#19816=ORIENTED_EDGE('',*,*,#14636,.F.);
#19817=ORIENTED_EDGE('',*,*,#14635,.F.);
#19818=ORIENTED_EDGE('',*,*,#14637,.F.);
#19819=ORIENTED_EDGE('',*,*,#14638,.T.);
#19820=ORIENTED_EDGE('',*,*,#14639,.F.);
#19821=ORIENTED_EDGE('',*,*,#14638,.F.);
#19822=ORIENTED_EDGE('',*,*,#14640,.F.);
#19823=ORIENTED_EDGE('',*,*,#14630,.T.);
#19824=ORIENTED_EDGE('',*,*,#14634,.T.);
#19825=ORIENTED_EDGE('',*,*,#14631,.T.);
#19826=ORIENTED_EDGE('',*,*,#14640,.T.);
#19827=ORIENTED_EDGE('',*,*,#14637,.T.);
#19828=ORIENTED_EDGE('',*,*,#14641,.F.);
#19829=ORIENTED_EDGE('',*,*,#14642,.T.);
#19830=ORIENTED_EDGE('',*,*,#14612,.T.);
#19831=ORIENTED_EDGE('',*,*,#14642,.F.);
#19832=ORIENTED_EDGE('',*,*,#14643,.F.);
#19833=ORIENTED_EDGE('',*,*,#14644,.T.);
#19834=ORIENTED_EDGE('',*,*,#14641,.T.);
#19835=ORIENTED_EDGE('',*,*,#14644,.F.);
#19836=ORIENTED_EDGE('',*,*,#14636,.T.);
#19837=ORIENTED_EDGE('',*,*,#14639,.T.);
#19838=ORIENTED_EDGE('',*,*,#14629,.T.);
#19839=ORIENTED_EDGE('',*,*,#14633,.T.);
#19840=ORIENTED_EDGE('',*,*,#14645,.F.);
#19841=ORIENTED_EDGE('',*,*,#14643,.T.);
#19842=ORIENTED_EDGE('',*,*,#14646,.F.);
#19843=ORIENTED_EDGE('',*,*,#14647,.T.);
#19844=ORIENTED_EDGE('',*,*,#14645,.T.);
#19845=ORIENTED_EDGE('',*,*,#14647,.F.);
#19846=ORIENTED_EDGE('',*,*,#14648,.F.);
#19847=ORIENTED_EDGE('',*,*,#14649,.T.);
#19848=ORIENTED_EDGE('',*,*,#14646,.T.);
#19849=ORIENTED_EDGE('',*,*,#14649,.F.);
#19850=ORIENTED_EDGE('',*,*,#14650,.F.);
#19851=ORIENTED_EDGE('',*,*,#14651,.T.);
#19852=ORIENTED_EDGE('',*,*,#14648,.T.);
#19853=ORIENTED_EDGE('',*,*,#14651,.F.);
#19854=ORIENTED_EDGE('',*,*,#14650,.T.);
#19855=ORIENTED_EDGE('',*,*,#14619,.T.);
#19856=ORIENTED_EDGE('',*,*,#14627,.T.);
#19857=ORIENTED_EDGE('',*,*,#14625,.T.);
#19858=ORIENTED_EDGE('',*,*,#14347,.F.);
#25018=CONICAL_SURFACE('',#27676,0.892677669529664,1.17809724509616);
#25019=CONICAL_SURFACE('',#27680,0.95,0.785398163397441);
#25020=CONICAL_SURFACE('',#27685,0.430000000000001,0.785398163397455);
#25021=CONICAL_SURFACE('',#27692,0.974822330470337,0.392699081698707);
#25022=CONICAL_SURFACE('',#27694,0.949822330470333,0.392699081698761);
#25023=CONICAL_SURFACE('',#27700,0.202500000000001,1.02974425867666);
#25024=CONICAL_SURFACE('',#27708,0.975,0.785398163397451);
#25025=CONICAL_SURFACE('',#27714,1.575,0.785398163397459);
#25026=CONICAL_SURFACE('',#27718,1.575,0.785398163397459);
#25549=ADVANCED_FACE('',(#2961),#1160,.T.);
#25550=ADVANCED_FACE('',(#2962),#1161,.T.);
#25551=ADVANCED_FACE('',(#2963),#1162,.T.);
#25552=ADVANCED_FACE('',(#2964),#1163,.T.);
#25553=ADVANCED_FACE('',(#2965),#1164,.T.);
#25554=ADVANCED_FACE('',(#2966),#1165,.T.);
#25555=ADVANCED_FACE('',(#2967),#1166,.T.);
#25556=ADVANCED_FACE('',(#2968),#1167,.T.);
#25557=ADVANCED_FACE('',(#2969),#1168,.T.);
#25558=ADVANCED_FACE('',(#2970),#1169,.T.);
#25559=ADVANCED_FACE('',(#2971),#1170,.T.);
#25560=ADVANCED_FACE('',(#2972),#1171,.T.);
#25561=ADVANCED_FACE('',(#2973),#1172,.T.);
#25562=ADVANCED_FACE('',(#2974),#1173,.T.);
#25563=ADVANCED_FACE('',(#2975),#1174,.T.);
#25564=ADVANCED_FACE('',(#2976),#1175,.T.);
#25565=ADVANCED_FACE('',(#2977),#1176,.T.);
#25566=ADVANCED_FACE('',(#2978),#1177,.T.);
#25567=ADVANCED_FACE('',(#2979),#1178,.T.);
#25568=ADVANCED_FACE('',(#2980),#1179,.T.);
#25569=ADVANCED_FACE('',(#2981),#1180,.T.);
#25570=ADVANCED_FACE('',(#2982),#1181,.T.);
#25571=ADVANCED_FACE('',(#2983),#1182,.T.);
#25572=ADVANCED_FACE('',(#2984),#1183,.T.);
#25573=ADVANCED_FACE('',(#2985),#1184,.T.);
#25574=ADVANCED_FACE('',(#2986),#1185,.T.);
#25575=ADVANCED_FACE('',(#2987),#1186,.T.);
#25576=ADVANCED_FACE('',(#2988),#1187,.T.);
#25577=ADVANCED_FACE('',(#2989),#1188,.T.);
#25578=ADVANCED_FACE('',(#2990),#1189,.T.);
#25579=ADVANCED_FACE('',(#2991),#1190,.T.);
#25580=ADVANCED_FACE('',(#2992),#1191,.T.);
#25581=ADVANCED_FACE('',(#2993),#1192,.T.);
#25582=ADVANCED_FACE('',(#2994),#1193,.T.);
#25583=ADVANCED_FACE('',(#2995),#1194,.T.);
#25584=ADVANCED_FACE('',(#2996),#1195,.T.);
#25585=ADVANCED_FACE('',(#2997),#1196,.T.);
#25586=ADVANCED_FACE('',(#2998),#1197,.T.);
#25587=ADVANCED_FACE('',(#2999),#1198,.T.);
#25588=ADVANCED_FACE('',(#3000),#1199,.T.);
#25589=ADVANCED_FACE('',(#3001),#1200,.T.);
#25590=ADVANCED_FACE('',(#3002),#1201,.T.);
#25591=ADVANCED_FACE('',(#3003),#1202,.T.);
#25592=ADVANCED_FACE('',(#3004),#1203,.T.);
#25593=ADVANCED_FACE('',(#3005),#1204,.T.);
#25594=ADVANCED_FACE('',(#3006),#1205,.T.);
#25595=ADVANCED_FACE('',(#3007),#1206,.T.);
#25596=ADVANCED_FACE('',(#3008),#1207,.T.);
#25597=ADVANCED_FACE('',(#3009),#1208,.T.);
#25598=ADVANCED_FACE('',(#3010),#1209,.T.);
#25599=ADVANCED_FACE('',(#3011),#1210,.T.);
#25600=ADVANCED_FACE('',(#3012),#1211,.T.);
#25601=ADVANCED_FACE('',(#3013),#1212,.T.);
#25602=ADVANCED_FACE('',(#3014),#1213,.T.);
#25603=ADVANCED_FACE('',(#3015),#1214,.T.);
#25604=ADVANCED_FACE('',(#3016),#1215,.T.);
#25605=ADVANCED_FACE('',(#3017),#1216,.T.);
#25606=ADVANCED_FACE('',(#3018),#1217,.T.);
#25607=ADVANCED_FACE('',(#3019),#1218,.T.);
#25608=ADVANCED_FACE('',(#3020),#1219,.T.);
#25609=ADVANCED_FACE('',(#3021),#1220,.T.);
#25610=ADVANCED_FACE('',(#3022),#1221,.T.);
#25611=ADVANCED_FACE('',(#3023),#1222,.T.);
#25612=ADVANCED_FACE('',(#3024),#1223,.T.);
#25613=ADVANCED_FACE('',(#3025),#1224,.T.);
#25614=ADVANCED_FACE('',(#3026),#1225,.T.);
#25615=ADVANCED_FACE('',(#3027),#1226,.T.);
#25616=ADVANCED_FACE('',(#3028),#1227,.T.);
#25617=ADVANCED_FACE('',(#3029),#1228,.T.);
#25618=ADVANCED_FACE('',(#3030),#1229,.T.);
#25619=ADVANCED_FACE('',(#3031),#1230,.T.);
#25620=ADVANCED_FACE('',(#3032),#1231,.T.);
#25621=ADVANCED_FACE('',(#3033),#1232,.T.);
#25622=ADVANCED_FACE('',(#3034),#1233,.T.);
#25623=ADVANCED_FACE('',(#3035),#1234,.T.);
#25624=ADVANCED_FACE('',(#3036),#1235,.T.);
#25625=ADVANCED_FACE('',(#3037),#1236,.T.);
#25626=ADVANCED_FACE('',(#3038),#1237,.T.);
#25627=ADVANCED_FACE('',(#3039),#1238,.T.);
#25628=ADVANCED_FACE('',(#3040),#1239,.T.);
#25629=ADVANCED_FACE('',(#3041),#1240,.T.);
#25630=ADVANCED_FACE('',(#3042),#1241,.T.);
#25631=ADVANCED_FACE('',(#3043),#1242,.T.);
#25632=ADVANCED_FACE('',(#3044),#1243,.T.);
#25633=ADVANCED_FACE('',(#3045),#25018,.T.);
#25634=ADVANCED_FACE('',(#3046),#25019,.T.);
#25635=ADVANCED_FACE('',(#3047),#1917,.T.);
#25636=ADVANCED_FACE('',(#3048),#25020,.F.);
#25637=ADVANCED_FACE('',(#3049),#1244,.F.);
#25638=ADVANCED_FACE('',(#3050,#1606),#1918,.T.);
#25639=ADVANCED_FACE('',(#3051),#25021,.T.);
#25640=ADVANCED_FACE('',(#3052),#158,.F.);
#25641=ADVANCED_FACE('',(#3053),#25022,.T.);
#25642=ADVANCED_FACE('',(#3054),#1919,.F.);
#25643=ADVANCED_FACE('',(#3055),#159,.F.);
#25644=ADVANCED_FACE('',(#3056),#1245,.T.);
#25645=ADVANCED_FACE('',(#3057),#1246,.T.);
#25646=ADVANCED_FACE('',(#3058),#25023,.F.);
#25647=ADVANCED_FACE('',(#3059),#1920,.F.);
#25648=ADVANCED_FACE('',(#3060),#1247,.F.);
#25649=ADVANCED_FACE('',(#3061),#1921,.F.);
#25650=ADVANCED_FACE('',(#3062),#1248,.F.);
#25651=ADVANCED_FACE('',(#3063),#1922,.T.);
#25652=ADVANCED_FACE('',(#3064),#25024,.T.);
#25653=ADVANCED_FACE('',(#3065,#1607),#1249,.T.);
#25654=ADVANCED_FACE('',(#3066,#1608),#1923,.T.);
#25655=ADVANCED_FACE('',(#3067),#25025,.T.);
#25656=ADVANCED_FACE('',(#3068),#1250,.T.);
#25657=ADVANCED_FACE('',(#3069),#25026,.T.);
#25658=ADVANCED_FACE('',(#3070,#1609),#1924,.T.);
#26668=CLOSED_SHELL('',(#25549,#25550,#25551,#25552,#25553,#25554,#25555,
#25556,#25557,#25558,#25559,#25560,#25561,#25562,#25563,#25564,#25565,#25566,
#25567,#25568,#25569,#25570,#25571,#25572,#25573,#25574,#25575,#25576,#25577,
#25578,#25579,#25580,#25581,#25582,#25583,#25584,#25585,#25586,#25587,#25588,
#25589,#25590,#25591,#25592,#25593,#25594,#25595,#25596,#25597,#25598,#25599,
#25600,#25601,#25602,#25603,#25604,#25605,#25606,#25607,#25608,#25609,#25610,
#25611,#25612,#25613,#25614,#25615,#25616,#25617,#25618,#25619,#25620,#25621,
#25622,#25623,#25624,#25625,#25626,#25627,#25628,#25629,#25630,#25631,#25632,
#25633,#25634,#25635,#25636,#25637,#25638,#25639,#25640,#25641,#25642,#25643,
#25644,#25645,#25646,#25647,#25648,#25649,#25650,#25651,#25652,#25653,#25654,
#25655,#25656,#25657,#25658));
#27589=AXIS2_PLACEMENT_3D('',#40094,#31416,#31417);
#27590=AXIS2_PLACEMENT_3D('',#40095,#31418,#31419);
#27591=AXIS2_PLACEMENT_3D('',#40123,#31421,#31422);
#27592=AXIS2_PLACEMENT_3D('',#40128,#31423,#31424);
#27593=AXIS2_PLACEMENT_3D('',#40212,#31426,#31427);
#27594=AXIS2_PLACEMENT_3D('',#40299,#31429,#31430);
#27595=AXIS2_PLACEMENT_3D('',#40383,#31432,#31433);
#27596=AXIS2_PLACEMENT_3D('',#40455,#31435,#31436);
#27597=AXIS2_PLACEMENT_3D('',#40524,#31438,#31439);
#27598=AXIS2_PLACEMENT_3D('',#40608,#31441,#31442);
#27599=AXIS2_PLACEMENT_3D('',#40692,#31444,#31445);
#27600=AXIS2_PLACEMENT_3D('',#40779,#31447,#31448);
#27601=AXIS2_PLACEMENT_3D('',#40863,#31450,#31451);
#27602=AXIS2_PLACEMENT_3D('',#40950,#31453,#31454);
#27603=AXIS2_PLACEMENT_3D('',#41034,#31456,#31457);
#27604=AXIS2_PLACEMENT_3D('',#41118,#31459,#31460);
#27605=AXIS2_PLACEMENT_3D('',#41205,#31462,#31463);
#27606=AXIS2_PLACEMENT_3D('',#41274,#31465,#31466);
#27607=AXIS2_PLACEMENT_3D('',#41346,#31468,#31469);
#27608=AXIS2_PLACEMENT_3D('',#41427,#31471,#31472);
#27609=AXIS2_PLACEMENT_3D('',#41514,#31474,#31475);
#27610=AXIS2_PLACEMENT_3D('',#41601,#31477,#31478);
#27611=AXIS2_PLACEMENT_3D('',#41685,#31480,#31481);
#27612=AXIS2_PLACEMENT_3D('',#41772,#31483,#31484);
#27613=AXIS2_PLACEMENT_3D('',#41844,#31486,#31487);
#27614=AXIS2_PLACEMENT_3D('',#41934,#31489,#31490);
#27615=AXIS2_PLACEMENT_3D('',#42018,#31492,#31493);
#27616=AXIS2_PLACEMENT_3D('',#42102,#31495,#31496);
#27617=AXIS2_PLACEMENT_3D('',#42189,#31498,#31499);
#27618=AXIS2_PLACEMENT_3D('',#42270,#31501,#31502);
#27619=AXIS2_PLACEMENT_3D('',#42342,#31504,#31505);
#27620=AXIS2_PLACEMENT_3D('',#42411,#31507,#31508);
#27621=AXIS2_PLACEMENT_3D('',#42495,#31510,#31511);
#27622=AXIS2_PLACEMENT_3D('',#42579,#31513,#31514);
#27623=AXIS2_PLACEMENT_3D('',#42663,#31516,#31517);
#27624=AXIS2_PLACEMENT_3D('',#42753,#31519,#31520);
#27625=AXIS2_PLACEMENT_3D('',#42837,#31522,#31523);
#27626=AXIS2_PLACEMENT_3D('',#42921,#31525,#31526);
#27627=AXIS2_PLACEMENT_3D('',#43005,#31528,#31529);
#27628=AXIS2_PLACEMENT_3D('',#43089,#31531,#31532);
#27629=AXIS2_PLACEMENT_3D('',#43158,#31534,#31535);
#27630=AXIS2_PLACEMENT_3D('',#43242,#31537,#31538);
#27631=AXIS2_PLACEMENT_3D('',#43329,#31540,#31541);
#27632=AXIS2_PLACEMENT_3D('',#43413,#31543,#31544);
#27633=AXIS2_PLACEMENT_3D('',#43497,#31546,#31547);
#27634=AXIS2_PLACEMENT_3D('',#43513,#31549,#31550);
#27635=AXIS2_PLACEMENT_3D('',#43519,#31551,#31552);
#27636=AXIS2_PLACEMENT_3D('',#43554,#31554,#31555);
#27637=AXIS2_PLACEMENT_3D('',#43591,#31557,#31558);
#27638=AXIS2_PLACEMENT_3D('',#43627,#31560,#31561);
#27639=AXIS2_PLACEMENT_3D('',#43663,#31563,#31564);
#27640=AXIS2_PLACEMENT_3D('',#43709,#31566,#31567);
#27641=AXIS2_PLACEMENT_3D('',#43744,#31569,#31570);
#27642=AXIS2_PLACEMENT_3D('',#43781,#31572,#31573);
#27643=AXIS2_PLACEMENT_3D('',#43816,#31575,#31576);
#27644=AXIS2_PLACEMENT_3D('',#43853,#31578,#31579);
#27645=AXIS2_PLACEMENT_3D('',#43890,#31581,#31582);
#27646=AXIS2_PLACEMENT_3D('',#43926,#31584,#31585);
#27647=AXIS2_PLACEMENT_3D('',#43963,#31587,#31588);
#27648=AXIS2_PLACEMENT_3D('',#43998,#31590,#31591);
#27649=AXIS2_PLACEMENT_3D('',#44035,#31593,#31594);
#27650=AXIS2_PLACEMENT_3D('',#44080,#31596,#31597);
#27651=AXIS2_PLACEMENT_3D('',#44116,#31599,#31600);
#27652=AXIS2_PLACEMENT_3D('',#44152,#31602,#31603);
#27653=AXIS2_PLACEMENT_3D('',#44188,#31605,#31606);
#27654=AXIS2_PLACEMENT_3D('',#44225,#31608,#31609);
#27655=AXIS2_PLACEMENT_3D('',#44262,#31611,#31612);
#27656=AXIS2_PLACEMENT_3D('',#44297,#31614,#31615);
#27657=AXIS2_PLACEMENT_3D('',#44331,#31617,#31618);
#27658=AXIS2_PLACEMENT_3D('',#44368,#31620,#31621);
#27659=AXIS2_PLACEMENT_3D('',#44404,#31623,#31624);
#27660=AXIS2_PLACEMENT_3D('',#44441,#31626,#31627);
#27661=AXIS2_PLACEMENT_3D('',#44477,#31629,#31630);
#27662=AXIS2_PLACEMENT_3D('',#44513,#31632,#31633);
#27663=AXIS2_PLACEMENT_3D('',#44549,#31635,#31636);
#27664=AXIS2_PLACEMENT_3D('',#44585,#31638,#31639);
#27665=AXIS2_PLACEMENT_3D('',#44622,#31641,#31642);
#27666=AXIS2_PLACEMENT_3D('',#44657,#31644,#31645);
#27667=AXIS2_PLACEMENT_3D('',#44694,#31647,#31648);
#27668=AXIS2_PLACEMENT_3D('',#44731,#31650,#31651);
#27669=AXIS2_PLACEMENT_3D('',#44767,#31653,#31654);
#27670=AXIS2_PLACEMENT_3D('',#44804,#31656,#31657);
#27671=AXIS2_PLACEMENT_3D('',#44839,#31659,#31660);
#27672=AXIS2_PLACEMENT_3D('',#44876,#31662,#31663);
#27673=AXIS2_PLACEMENT_3D('',#44911,#31665,#31666);
#27674=AXIS2_PLACEMENT_3D('',#44948,#31668,#31669);
#27675=AXIS2_PLACEMENT_3D('',#44984,#31671,#31672);
#27676=AXIS2_PLACEMENT_3D('',#45020,#31674,#31675);
#27677=AXIS2_PLACEMENT_3D('',#45022,#31676,#31677);
#27678=AXIS2_PLACEMENT_3D('',#45026,#31679,#31680);
#27679=AXIS2_PLACEMENT_3D('',#45027,#31681,#31682);
#27680=AXIS2_PLACEMENT_3D('',#45028,#31683,#31684);
#27681=AXIS2_PLACEMENT_3D('',#45032,#31686,#31687);
#27682=AXIS2_PLACEMENT_3D('',#45034,#31688,#31689);
#27683=AXIS2_PLACEMENT_3D('',#45035,#31690,#31691);
#27684=AXIS2_PLACEMENT_3D('',#45036,#31692,#31693);
#27685=AXIS2_PLACEMENT_3D('',#45037,#31694,#31695);
#27686=AXIS2_PLACEMENT_3D('',#45039,#31696,#31697);
#27687=AXIS2_PLACEMENT_3D('',#45042,#31699,#31700);
#27688=AXIS2_PLACEMENT_3D('',#45043,#31701,#31702);
#27689=AXIS2_PLACEMENT_3D('',#45045,#31703,#31704);
#27690=AXIS2_PLACEMENT_3D('',#45047,#31706,#31707);
#27691=AXIS2_PLACEMENT_3D('',#45049,#31708,#31709);
#27692=AXIS2_PLACEMENT_3D('',#45050,#31710,#31711);
#27693=AXIS2_PLACEMENT_3D('',#45163,#31712,#31713);
#27694=AXIS2_PLACEMENT_3D('',#47277,#31714,#31715);
#27695=AXIS2_PLACEMENT_3D('',#47298,#31716,#31717);
#27696=AXIS2_PLACEMENT_3D('',#47299,#31718,#31719);
#27697=AXIS2_PLACEMENT_3D('',#49540,#31720,#31721);
#27698=AXIS2_PLACEMENT_3D('',#49541,#31722,#31723);
#27699=AXIS2_PLACEMENT_3D('',#49542,#31724,#31725);
#27700=AXIS2_PLACEMENT_3D('',#49543,#31726,#31727);
#27701=AXIS2_PLACEMENT_3D('',#49546,#31729,#31730);
#27702=AXIS2_PLACEMENT_3D('',#49555,#31735,#31736);
#27703=AXIS2_PLACEMENT_3D('',#49576,#31737,#31738);
#27704=AXIS2_PLACEMENT_3D('',#49578,#31740,#31741);
#27705=AXIS2_PLACEMENT_3D('',#49584,#31745,#31746);
#27706=AXIS2_PLACEMENT_3D('',#49603,#31747,#31748);
#27707=AXIS2_PLACEMENT_3D('',#49604,#31749,#31750);
#27708=AXIS2_PLACEMENT_3D('',#49605,#31751,#31752);
#27709=AXIS2_PLACEMENT_3D('',#49607,#31753,#31754);
#27710=AXIS2_PLACEMENT_3D('',#49609,#31756,#31757);
#27711=AXIS2_PLACEMENT_3D('',#49611,#31758,#31759);
#27712=AXIS2_PLACEMENT_3D('',#49613,#31761,#31762);
#27713=AXIS2_PLACEMENT_3D('',#49615,#31763,#31764);
#27714=AXIS2_PLACEMENT_3D('',#49616,#31765,#31766);
#27715=AXIS2_PLACEMENT_3D('',#49618,#31767,#31768);
#27716=AXIS2_PLACEMENT_3D('',#49620,#31770,#31771);
#27717=AXIS2_PLACEMENT_3D('',#49622,#31772,#31773);
#27718=AXIS2_PLACEMENT_3D('',#49624,#31775,#31776);
#27719=AXIS2_PLACEMENT_3D('',#49626,#31777,#31778);
#27720=AXIS2_PLACEMENT_3D('',#49628,#31780,#31781);
#31416=DIRECTION('axis',(0.,0.,1.));
#31417=DIRECTION('refdir',(1.,0.,0.));
#31418=DIRECTION('center_axis',(1.,0.,0.));
#31419=DIRECTION('ref_axis',(0.,-0.216887865424076,0.976196524185468));
#31420=DIRECTION('',(-1.,0.,0.));
#31421=DIRECTION('center_axis',(-1.,0.,0.));
#31422=DIRECTION('ref_axis',(0.,1.,0.));
#31423=DIRECTION('center_axis',(1.,0.,0.));
#31424=DIRECTION('ref_axis',(0.,1.,0.));
#31425=DIRECTION('',(-1.,0.,0.));
#31426=DIRECTION('center_axis',(1.,0.,0.));
#31427=DIRECTION('ref_axis',(0.,1.,0.));
#31428=DIRECTION('',(-1.,0.,0.));
#31429=DIRECTION('center_axis',(1.,0.,0.));
#31430=DIRECTION('ref_axis',(0.,1.,0.));
#31431=DIRECTION('',(-1.,0.,0.));
#31432=DIRECTION('center_axis',(1.,0.,0.));
#31433=DIRECTION('ref_axis',(0.,1.,0.));
#31434=DIRECTION('',(-1.,0.,0.));
#31435=DIRECTION('center_axis',(1.,0.,0.));
#31436=DIRECTION('ref_axis',(0.,1.,0.));
#31437=DIRECTION('',(-1.,0.,0.));
#31438=DIRECTION('center_axis',(1.,0.,0.));
#31439=DIRECTION('ref_axis',(0.,1.,0.));
#31440=DIRECTION('',(-1.,0.,0.));
#31441=DIRECTION('center_axis',(1.,0.,0.));
#31442=DIRECTION('ref_axis',(0.,1.,0.));
#31443=DIRECTION('',(-1.,0.,0.));
#31444=DIRECTION('center_axis',(1.,0.,0.));
#31445=DIRECTION('ref_axis',(0.,1.,0.));
#31446=DIRECTION('',(-1.,0.,0.));
#31447=DIRECTION('center_axis',(1.,0.,0.));
#31448=DIRECTION('ref_axis',(0.,1.,0.));
#31449=DIRECTION('',(-1.,0.,0.));
#31450=DIRECTION('center_axis',(1.,0.,0.));
#31451=DIRECTION('ref_axis',(0.,1.,0.));
#31452=DIRECTION('',(-1.,0.,0.));
#31453=DIRECTION('center_axis',(1.,0.,0.));
#31454=DIRECTION('ref_axis',(0.,1.,0.));
#31455=DIRECTION('',(-1.,0.,0.));
#31456=DIRECTION('center_axis',(1.,0.,0.));
#31457=DIRECTION('ref_axis',(0.,1.,0.));
#31458=DIRECTION('',(-1.,0.,0.));
#31459=DIRECTION('center_axis',(1.,0.,0.));
#31460=DIRECTION('ref_axis',(0.,1.,0.));
#31461=DIRECTION('',(-1.,0.,0.));
#31462=DIRECTION('center_axis',(1.,0.,0.));
#31463=DIRECTION('ref_axis',(0.,1.,0.));
#31464=DIRECTION('',(-1.,0.,0.));
#31465=DIRECTION('center_axis',(1.,0.,0.));
#31466=DIRECTION('ref_axis',(0.,1.,0.));
#31467=DIRECTION('',(-1.,0.,0.));
#31468=DIRECTION('center_axis',(1.,0.,0.));
#31469=DIRECTION('ref_axis',(0.,1.,0.));
#31470=DIRECTION('',(-1.,0.,0.));
#31471=DIRECTION('center_axis',(1.,0.,0.));
#31472=DIRECTION('ref_axis',(0.,1.,0.));
#31473=DIRECTION('',(-1.,0.,0.));
#31474=DIRECTION('center_axis',(1.,0.,0.));
#31475=DIRECTION('ref_axis',(0.,1.,0.));
#31476=DIRECTION('',(-1.,0.,0.));
#31477=DIRECTION('center_axis',(1.,0.,0.));
#31478=DIRECTION('ref_axis',(0.,1.,0.));
#31479=DIRECTION('',(-1.,0.,0.));
#31480=DIRECTION('center_axis',(1.,0.,0.));
#31481=DIRECTION('ref_axis',(0.,1.,0.));
#31482=DIRECTION('',(-1.,0.,0.));
#31483=DIRECTION('center_axis',(1.,0.,0.));
#31484=DIRECTION('ref_axis',(0.,1.,0.));
#31485=DIRECTION('',(-1.,0.,0.));
#31486=DIRECTION('center_axis',(1.,0.,0.));
#31487=DIRECTION('ref_axis',(0.,1.,0.));
#31488=DIRECTION('',(-1.,0.,0.));
#31489=DIRECTION('center_axis',(1.,0.,0.));
#31490=DIRECTION('ref_axis',(0.,1.,0.));
#31491=DIRECTION('',(-1.,0.,0.));
#31492=DIRECTION('center_axis',(1.,0.,0.));
#31493=DIRECTION('ref_axis',(0.,1.,0.));
#31494=DIRECTION('',(-1.,0.,0.));
#31495=DIRECTION('center_axis',(1.,0.,0.));
#31496=DIRECTION('ref_axis',(0.,1.,0.));
#31497=DIRECTION('',(-1.,0.,0.));
#31498=DIRECTION('center_axis',(1.,0.,0.));
#31499=DIRECTION('ref_axis',(0.,1.,0.));
#31500=DIRECTION('',(-1.,0.,0.));
#31501=DIRECTION('center_axis',(1.,0.,0.));
#31502=DIRECTION('ref_axis',(0.,1.,0.));
#31503=DIRECTION('',(-1.,0.,0.));
#31504=DIRECTION('center_axis',(1.,0.,0.));
#31505=DIRECTION('ref_axis',(0.,1.,0.));
#31506=DIRECTION('',(-1.,0.,0.));
#31507=DIRECTION('center_axis',(1.,0.,0.));
#31508=DIRECTION('ref_axis',(0.,1.,0.));
#31509=DIRECTION('',(-1.,0.,0.));
#31510=DIRECTION('center_axis',(1.,0.,0.));
#31511=DIRECTION('ref_axis',(0.,1.,0.));
#31512=DIRECTION('',(-1.,0.,0.));
#31513=DIRECTION('center_axis',(1.,0.,0.));
#31514=DIRECTION('ref_axis',(0.,1.,0.));
#31515=DIRECTION('',(-1.,0.,0.));
#31516=DIRECTION('center_axis',(1.,0.,0.));
#31517=DIRECTION('ref_axis',(0.,1.,0.));
#31518=DIRECTION('',(-1.,0.,0.));
#31519=DIRECTION('center_axis',(1.,0.,0.));
#31520=DIRECTION('ref_axis',(0.,1.,0.));
#31521=DIRECTION('',(-1.,0.,0.));
#31522=DIRECTION('center_axis',(1.,0.,0.));
#31523=DIRECTION('ref_axis',(0.,1.,0.));
#31524=DIRECTION('',(-1.,0.,0.));
#31525=DIRECTION('center_axis',(1.,0.,0.));
#31526=DIRECTION('ref_axis',(0.,1.,0.));
#31527=DIRECTION('',(-1.,0.,0.));
#31528=DIRECTION('center_axis',(1.,0.,0.));
#31529=DIRECTION('ref_axis',(0.,1.,0.));
#31530=DIRECTION('',(-1.,0.,0.));
#31531=DIRECTION('center_axis',(1.,0.,0.));
#31532=DIRECTION('ref_axis',(0.,1.,0.));
#31533=DIRECTION('',(-1.,0.,0.));
#31534=DIRECTION('center_axis',(1.,0.,0.));
#31535=DIRECTION('ref_axis',(0.,1.,0.));
#31536=DIRECTION('',(-1.,0.,0.));
#31537=DIRECTION('center_axis',(1.,0.,0.));
#31538=DIRECTION('ref_axis',(0.,1.,0.));
#31539=DIRECTION('',(-1.,0.,0.));
#31540=DIRECTION('center_axis',(1.,0.,0.));
#31541=DIRECTION('ref_axis',(0.,1.,0.));
#31542=DIRECTION('',(-1.,0.,0.));
#31543=DIRECTION('center_axis',(1.,0.,0.));
#31544=DIRECTION('ref_axis',(0.,1.,0.));
#31545=DIRECTION('',(-1.,0.,0.));
#31546=DIRECTION('center_axis',(1.,0.,0.));
#31547=DIRECTION('ref_axis',(0.,-0.201340086992588,-0.979521398117375));
#31548=DIRECTION('',(1.,0.,0.));
#31549=DIRECTION('center_axis',(1.,0.,0.));
#31550=DIRECTION('ref_axis',(0.,1.,-4.88042043924972E-13));
#31551=DIRECTION('center_axis',(1.,0.,0.));
#31552=DIRECTION('ref_axis',(0.,1.,-4.88042043924972E-13));
#31553=DIRECTION('',(1.,0.,0.));
#31554=DIRECTION('center_axis',(1.,0.,0.));
#31555=DIRECTION('ref_axis',(0.,1.,-4.88042043924972E-13));
#31556=DIRECTION('',(1.,0.,0.));
#31557=DIRECTION('center_axis',(1.,0.,0.));
#31558=DIRECTION('ref_axis',(0.,1.,-4.88042043924972E-13));
#31559=DIRECTION('',(1.,0.,0.));
#31560=DIRECTION('center_axis',(1.,0.,0.));
#31561=DIRECTION('ref_axis',(0.,1.,-4.88042043924972E-13));
#31562=DIRECTION('',(1.,0.,0.));
#31563=DIRECTION('center_axis',(1.,0.,0.));
#31564=DIRECTION('ref_axis',(0.,1.,-4.88042043924972E-13));
#31565=DIRECTION('',(1.,0.,0.));
#31566=DIRECTION('center_axis',(1.,0.,0.));
#31567=DIRECTION('ref_axis',(0.,1.,-4.88042043924972E-13));
#31568=DIRECTION('',(1.,0.,0.));
#31569=DIRECTION('center_axis',(1.,0.,0.));
#31570=DIRECTION('ref_axis',(0.,1.,-4.88042043924972E-13));
#31571=DIRECTION('',(1.,0.,0.));
#31572=DIRECTION('center_axis',(1.,0.,0.));
#31573=DIRECTION('ref_axis',(0.,1.,-4.88042043924972E-13));
#31574=DIRECTION('',(1.,0.,0.));
#31575=DIRECTION('center_axis',(1.,0.,0.));
#31576=DIRECTION('ref_axis',(0.,1.,-4.88042043924972E-13));
#31577=DIRECTION('',(1.,0.,0.));
#31578=DIRECTION('center_axis',(1.,0.,0.));
#31579=DIRECTION('ref_axis',(0.,1.,-4.88042043924972E-13));
#31580=DIRECTION('',(1.,0.,0.));
#31581=DIRECTION('center_axis',(1.,0.,0.));
#31582=DIRECTION('ref_axis',(0.,1.,-4.88042043924972E-13));
#31583=DIRECTION('',(1.,0.,0.));
#31584=DIRECTION('center_axis',(1.,0.,0.));
#31585=DIRECTION('ref_axis',(0.,1.,-4.88042043924972E-13));
#31586=DIRECTION('',(1.,0.,0.));
#31587=DIRECTION('center_axis',(1.,0.,0.));
#31588=DIRECTION('ref_axis',(0.,1.,-4.88042043924972E-13));
#31589=DIRECTION('',(1.,0.,0.));
#31590=DIRECTION('center_axis',(1.,0.,0.));
#31591=DIRECTION('ref_axis',(0.,1.,-4.88042043924972E-13));
#31592=DIRECTION('',(1.,0.,0.));
#31593=DIRECTION('center_axis',(1.,0.,0.));
#31594=DIRECTION('ref_axis',(0.,1.,-4.88042043924972E-13));
#31595=DIRECTION('',(1.,0.,0.));
#31596=DIRECTION('center_axis',(1.,0.,0.));
#31597=DIRECTION('ref_axis',(0.,1.,-4.88042043924972E-13));
#31598=DIRECTION('',(1.,0.,0.));
#31599=DIRECTION('center_axis',(1.,0.,0.));
#31600=DIRECTION('ref_axis',(0.,1.,-4.88042043924972E-13));
#31601=DIRECTION('',(1.,0.,0.));
#31602=DIRECTION('center_axis',(1.,0.,0.));
#31603=DIRECTION('ref_axis',(0.,1.,-4.88042043924972E-13));
#31604=DIRECTION('',(1.,0.,0.));
#31605=DIRECTION('center_axis',(1.,0.,0.));
#31606=DIRECTION('ref_axis',(0.,1.,-4.88042043924972E-13));
#31607=DIRECTION('',(1.,0.,0.));
#31608=DIRECTION('center_axis',(1.,0.,0.));
#31609=DIRECTION('ref_axis',(0.,1.,-4.88042043924972E-13));
#31610=DIRECTION('',(1.,0.,0.));
#31611=DIRECTION('center_axis',(1.,0.,0.));
#31612=DIRECTION('ref_axis',(0.,1.,-4.88042043924972E-13));
#31613=DIRECTION('',(1.,0.,0.));
#31614=DIRECTION('center_axis',(1.,0.,0.));
#31615=DIRECTION('ref_axis',(0.,1.,-4.88042043924972E-13));
#31616=DIRECTION('',(1.,0.,0.));
#31617=DIRECTION('center_axis',(1.,0.,0.));
#31618=DIRECTION('ref_axis',(0.,1.,-4.88042043924972E-13));
#31619=DIRECTION('',(1.,0.,0.));
#31620=DIRECTION('center_axis',(1.,0.,0.));
#31621=DIRECTION('ref_axis',(0.,1.,-4.88042043924972E-13));
#31622=DIRECTION('',(1.,0.,0.));
#31623=DIRECTION('center_axis',(1.,0.,0.));
#31624=DIRECTION('ref_axis',(0.,1.,-4.88042043924972E-13));
#31625=DIRECTION('',(1.,0.,0.));
#31626=DIRECTION('center_axis',(1.,0.,0.));
#31627=DIRECTION('ref_axis',(0.,1.,-4.88042043924972E-13));
#31628=DIRECTION('',(1.,0.,0.));
#31629=DIRECTION('center_axis',(1.,0.,0.));
#31630=DIRECTION('ref_axis',(0.,1.,-4.88042043924972E-13));
#31631=DIRECTION('',(1.,0.,0.));
#31632=DIRECTION('center_axis',(1.,0.,0.));
#31633=DIRECTION('ref_axis',(0.,1.,-4.88042043924972E-13));
#31634=DIRECTION('',(1.,0.,0.));
#31635=DIRECTION('center_axis',(1.,0.,0.));
#31636=DIRECTION('ref_axis',(0.,1.,-4.88042043924972E-13));
#31637=DIRECTION('',(1.,0.,0.));
#31638=DIRECTION('center_axis',(1.,0.,0.));
#31639=DIRECTION('ref_axis',(0.,1.,-4.88042043924972E-13));
#31640=DIRECTION('',(1.,0.,0.));
#31641=DIRECTION('center_axis',(1.,0.,0.));
#31642=DIRECTION('ref_axis',(0.,1.,-4.88042043924972E-13));
#31643=DIRECTION('',(1.,0.,0.));
#31644=DIRECTION('center_axis',(1.,0.,0.));
#31645=DIRECTION('ref_axis',(0.,1.,-4.88042043924972E-13));
#31646=DIRECTION('',(1.,0.,0.));
#31647=DIRECTION('center_axis',(1.,0.,0.));
#31648=DIRECTION('ref_axis',(0.,1.,-4.88042043924972E-13));
#31649=DIRECTION('',(1.,0.,0.));
#31650=DIRECTION('center_axis',(1.,0.,0.));
#31651=DIRECTION('ref_axis',(0.,1.,-4.88042043924972E-13));
#31652=DIRECTION('',(1.,0.,0.));
#31653=DIRECTION('center_axis',(1.,0.,0.));
#31654=DIRECTION('ref_axis',(0.,1.,-4.88042043924972E-13));
#31655=DIRECTION('',(1.,0.,0.));
#31656=DIRECTION('center_axis',(1.,0.,0.));
#31657=DIRECTION('ref_axis',(0.,1.,-4.88042043924972E-13));
#31658=DIRECTION('',(1.,0.,0.));
#31659=DIRECTION('center_axis',(1.,0.,0.));
#31660=DIRECTION('ref_axis',(0.,1.,-4.88042043924972E-13));
#31661=DIRECTION('',(1.,0.,0.));
#31662=DIRECTION('center_axis',(1.,0.,0.));
#31663=DIRECTION('ref_axis',(0.,1.,-4.88042043924972E-13));
#31664=DIRECTION('',(1.,0.,0.));
#31665=DIRECTION('center_axis',(1.,0.,0.));
#31666=DIRECTION('ref_axis',(0.,1.,-4.88042043924972E-13));
#31667=DIRECTION('',(1.,0.,0.));
#31668=DIRECTION('center_axis',(1.,0.,0.));
#31669=DIRECTION('ref_axis',(0.,1.,-4.88042043924972E-13));
#31670=DIRECTION('',(1.,0.,0.));
#31671=DIRECTION('center_axis',(1.,0.,0.));
#31672=DIRECTION('ref_axis',(0.,1.,-4.88042043924972E-13));
#31673=DIRECTION('',(1.,0.,0.));
#31674=DIRECTION('center_axis',(-1.,0.,0.));
#31675=DIRECTION('ref_axis',(0.,-1.,0.));
#31676=DIRECTION('center_axis',(-1.,0.,0.));
#31677=DIRECTION('ref_axis',(0.,-1.,0.));
#31678=DIRECTION('',(-0.382683432365103,0.923879532511281,1.13142611228769E-16));
#31679=DIRECTION('center_axis',(1.,0.,0.));
#31680=DIRECTION('ref_axis',(0.,-1.,0.));
#31681=DIRECTION('center_axis',(1.,0.,0.));
#31682=DIRECTION('ref_axis',(0.,-1.,0.));
#31683=DIRECTION('center_axis',(-1.,0.,0.));
#31684=DIRECTION('ref_axis',(0.,1.,0.));
#31685=DIRECTION('',(-0.707106781186553,-0.707106781186542,-8.65956056235487E-17));
#31686=DIRECTION('center_axis',(-1.,0.,0.));
#31687=DIRECTION('ref_axis',(0.,-1.,0.));
#31688=DIRECTION('center_axis',(-1.,0.,0.));
#31689=DIRECTION('ref_axis',(0.,1.,0.));
#31690=DIRECTION('center_axis',(-1.,0.,0.));
#31691=DIRECTION('ref_axis',(0.,-1.,0.));
#31692=DIRECTION('center_axis',(1.,0.,0.));
#31693=DIRECTION('ref_axis',(0.,0.,-1.));
#31694=DIRECTION('center_axis',(-1.,0.,0.));
#31695=DIRECTION('ref_axis',(0.,0.,1.));
#31696=DIRECTION('center_axis',(-1.,0.,0.));
#31697=DIRECTION('ref_axis',(0.,0.,1.));
#31698=DIRECTION('',(0.707106781186543,8.65956056235499E-17,0.707106781186552));
#31699=DIRECTION('center_axis',(1.,0.,0.));
#31700=DIRECTION('ref_axis',(0.,0.,1.));
#31701=DIRECTION('center_axis',(-1.,0.,0.));
#31702=DIRECTION('ref_axis',(0.,0.,1.));
#31703=DIRECTION('center_axis',(-1.,0.,0.));
#31704=DIRECTION('ref_axis',(0.,0.,1.));
#31705=DIRECTION('',(-1.,0.,0.));
#31706=DIRECTION('center_axis',(-1.,0.,0.));
#31707=DIRECTION('ref_axis',(0.,0.,1.));
#31708=DIRECTION('center_axis',(1.,0.,0.));
#31709=DIRECTION('ref_axis',(0.,0.,-1.));
#31710=DIRECTION('center_axis',(-1.,0.,0.));
#31711=DIRECTION('ref_axis',(0.,-0.0771183618471287,0.997021944726401));
#31712=DIRECTION('center_axis',(1.,0.,0.));
#31713=DIRECTION('ref_axis',(0.,-1.,0.));
#31714=DIRECTION('center_axis',(1.,0.,0.));
#31715=DIRECTION('ref_axis',(0.,0.413513095306714,-0.91049817133801));
#31716=DIRECTION('center_axis',(1.,0.,0.));
#31717=DIRECTION('ref_axis',(0.,1.,0.));
#31718=DIRECTION('center_axis',(1.,0.,0.));
#31719=DIRECTION('ref_axis',(0.,0.,-1.));
#31720=DIRECTION('center_axis',(1.,0.,0.));
#31721=DIRECTION('ref_axis',(0.,0.965988671445919,0.258584389780489));
#31722=DIRECTION('center_axis',(-1.,0.,0.));
#31723=DIRECTION('ref_axis',(0.,1.,-4.88042043924972E-13));
#31724=DIRECTION('center_axis',(1.,0.,0.));
#31725=DIRECTION('ref_axis',(0.,0.851219542641563,-0.524809765748589));
#31726=DIRECTION('center_axis',(-1.,0.,0.));
#31727=DIRECTION('ref_axis',(0.,0.,1.));
#31728=DIRECTION('',(-0.515038074910053,-1.04972719113862E-16,-0.857167300702113));
#31729=DIRECTION('center_axis',(0.,-1.,0.));
#31730=DIRECTION('ref_axis',(1.,0.,0.));
#31731=DIRECTION('',(-1.,0.,0.));
#31732=DIRECTION('',(0.,0.,1.));
#31733=DIRECTION('',(1.,0.,0.));
#31734=DIRECTION('',(0.,0.,1.));
#31735=DIRECTION('center_axis',(0.,0.,1.));
#31736=DIRECTION('ref_axis',(0.,1.,0.));
#31737=DIRECTION('center_axis',(0.,0.,1.));
#31738=DIRECTION('ref_axis',(0.,1.,0.));
#31739=DIRECTION('',(0.,0.,1.));
#31740=DIRECTION('center_axis',(0.,1.,0.));
#31741=DIRECTION('ref_axis',(-1.,0.,0.));
#31742=DIRECTION('',(1.,0.,0.));
#31743=DIRECTION('',(-1.,0.,0.));
#31744=DIRECTION('',(0.,0.,1.));
#31745=DIRECTION('center_axis',(0.,0.,1.));
#31746=DIRECTION('ref_axis',(0.,-1.,0.));
#31747=DIRECTION('center_axis',(0.,0.,1.));
#31748=DIRECTION('ref_axis',(0.,-1.,0.));
#31749=DIRECTION('center_axis',(0.,0.,1.));
#31750=DIRECTION('ref_axis',(1.,0.,0.));
#31751=DIRECTION('center_axis',(1.,0.,0.));
#31752=DIRECTION('ref_axis',(0.,1.,0.));
#31753=DIRECTION('center_axis',(1.,0.,0.));
#31754=DIRECTION('ref_axis',(0.,0.,-1.));
#31755=DIRECTION('',(-0.707106781186546,0.707106781186549,8.65956056235495E-17));
#31756=DIRECTION('center_axis',(1.,0.,0.));
#31757=DIRECTION('ref_axis',(0.,1.,0.));
#31758=DIRECTION('center_axis',(1.,0.,0.));
#31759=DIRECTION('ref_axis',(0.,0.,-1.));
#31760=DIRECTION('',(-1.,0.,0.));
#31761=DIRECTION('center_axis',(-1.,0.,0.));
#31762=DIRECTION('ref_axis',(0.,0.,1.));
#31763=DIRECTION('center_axis',(1.,0.,0.));
#31764=DIRECTION('ref_axis',(0.,0.,-1.));
#31765=DIRECTION('center_axis',(1.,0.,0.));
#31766=DIRECTION('ref_axis',(0.,1.,0.));
#31767=DIRECTION('center_axis',(1.,0.,0.));
#31768=DIRECTION('ref_axis',(0.,0.,-1.));
#31769=DIRECTION('',(-0.70710678118654,0.707106781186555,8.65956056235503E-17));
#31770=DIRECTION('center_axis',(1.,0.,0.));
#31771=DIRECTION('ref_axis',(0.,1.,0.));
#31772=DIRECTION('center_axis',(1.,0.,0.));
#31773=DIRECTION('ref_axis',(0.,0.,-1.));
#31774=DIRECTION('',(-1.,0.,0.));
#31775=DIRECTION('center_axis',(-1.,0.,0.));
#31776=DIRECTION('ref_axis',(0.,1.,0.));
#31777=DIRECTION('center_axis',(1.,0.,0.));
#31778=DIRECTION('ref_axis',(0.,0.,-1.));
#31779=DIRECTION('',(-0.70710678118654,-0.707106781186555,-8.65956056235503E-17));
#31780=DIRECTION('center_axis',(1.,0.,0.));
#31781=DIRECTION('ref_axis',(0.,0.,-1.));
#40094=CARTESIAN_POINT('',(0.,0.,0.));
#40095=CARTESIAN_POINT('Origin',(18.,0.,26.5));
#40096=CARTESIAN_POINT('',(9.77216677763621,-0.992506281688296,26.4999529602842));
#40097=CARTESIAN_POINT('',(9.62783322236381,-0.992554123075758,26.4999819653825));
#40098=CARTESIAN_POINT('',(18.,-0.9925,26.5));
#40099=CARTESIAN_POINT('',(9.6,0.899181451069001,26.9202569089796));
#40100=CARTESIAN_POINT('Ctrl Pts',(9.77216677763621,-0.992506281688296,
26.4999529602842));
#40101=CARTESIAN_POINT('Ctrl Pts',(9.76849906417681,-0.992322713406021,
26.5573892908763));
#40102=CARTESIAN_POINT('Ctrl Pts',(9.7648313507174,-0.98724997471646,26.6148019975283));
#40103=CARTESIAN_POINT('Ctrl Pts',(9.761163637258,-0.977330565296219,26.6712121339029));
#40104=CARTESIAN_POINT('Ctrl Pts',(9.75057810175747,-0.948701758350262,
26.8340196999224));
#40105=CARTESIAN_POINT('Ctrl Pts',(9.73999256625695,-0.879701126231576,
26.9884760503927));
#40106=CARTESIAN_POINT('Ctrl Pts',(9.72940703075642,-0.777206743663004,
27.1174316127062));
#40107=CARTESIAN_POINT('Ctrl Pts',(9.71882149525589,-0.674712361094432,
27.2463871750197));
#40108=CARTESIAN_POINT('Ctrl Pts',(9.70823595975535,-0.538724228075975,
27.3498419491765));
#40109=CARTESIAN_POINT('Ctrl Pts',(9.69765042425482,-0.386683814844797,
27.4142439267999));
#40110=CARTESIAN_POINT('Ctrl Pts',(9.68706488875429,-0.234643401613619,
27.4786459044233));
#40111=CARTESIAN_POINT('Ctrl Pts',(9.67647935325376,-0.0665507081697208,
27.5039950855134));
#40112=CARTESIAN_POINT('Ctrl Pts',(9.66589381775323,0.0975834738780521,
27.4877049736369));
#40113=CARTESIAN_POINT('Ctrl Pts',(9.65530828225269,0.261717655925824,27.4714148617604));
#40114=CARTESIAN_POINT('Ctrl Pts',(9.64472274675216,0.421893326577472,27.4134854569173));
#40115=CARTESIAN_POINT('Ctrl Pts',(9.63413721125163,0.558332210706581,27.3207204680017));
#40116=CARTESIAN_POINT('Ctrl Pts',(9.6235516757511,0.694771094835691,27.2279554790861));
#40117=CARTESIAN_POINT('Ctrl Pts',(9.61296614025056,0.807473192442262,27.1003549060981));
#40118=CARTESIAN_POINT('Ctrl Pts',(9.60238060475003,0.882858904166957,26.9535801505133));
#40119=CARTESIAN_POINT('Ctrl Pts',(9.60158706983336,0.888510124595916,26.9425773161798));
#40120=CARTESIAN_POINT('Ctrl Pts',(9.60079353491668,0.893951641373926,26.9314667303586));
#40121=CARTESIAN_POINT('Ctrl Pts',(9.6,0.899181451069001,26.9202569089796));
#40122=CARTESIAN_POINT('',(9.6,-0.89914483070475,26.9202318686356));
#40123=CARTESIAN_POINT('Origin',(9.6,0.,26.5));
#40124=CARTESIAN_POINT('Ctrl Pts',(9.59999999999999,-0.899144830704751,
26.9202318686356));
#40125=CARTESIAN_POINT('Ctrl Pts',(9.60927774078793,-0.960387074776627,
26.7891955258737));
#40126=CARTESIAN_POINT('Ctrl Pts',(9.61855548157587,-0.992405952059857,
26.6445725249488));
#40127=CARTESIAN_POINT('Ctrl Pts',(9.62783322236381,-0.992554123075758,
26.4999819653825));
#40128=CARTESIAN_POINT('Origin',(18.,0.,26.5));
#40129=CARTESIAN_POINT('',(10.1721667776362,-0.992592959832253,26.4996174405759));
#40130=CARTESIAN_POINT('',(10.0278332223638,-0.992418708717116,26.5000088356422));
#40131=CARTESIAN_POINT('',(18.,-0.9925,26.5));
#40132=CARTESIAN_POINT('Ctrl Pts',(10.1721667776362,-0.992592959832253,
26.4996174405759));
#40133=CARTESIAN_POINT('Ctrl Pts',(10.1621921568499,-0.992517835256568,
26.654933495308));
#40134=CARTESIAN_POINT('Ctrl Pts',(10.1522175360635,-0.955345472933135,
26.8110036453976));
#40135=CARTESIAN_POINT('Ctrl Pts',(10.1422429152772,-0.884928666211468,
26.9497422894547));
#40136=CARTESIAN_POINT('Ctrl Pts',(10.1316573797766,-0.810199047577096,
27.0969782469332));
#40137=CARTESIAN_POINT('Ctrl Pts',(10.1210718442761,-0.698028039439853,
27.2246946822847));
#40138=CARTESIAN_POINT('Ctrl Pts',(10.1104863087756,-0.562037531190435,
27.3180407059247));
#40139=CARTESIAN_POINT('Ctrl Pts',(10.099900773275,-0.426047022941016,27.4113867295647));
#40140=CARTESIAN_POINT('Ctrl Pts',(10.0893152377745,-0.266237014579421,
27.4703623414932));
#40141=CARTESIAN_POINT('Ctrl Pts',(10.078729702274,-0.102133462578573,27.4873735628633));
#40142=CARTESIAN_POINT('Ctrl Pts',(10.0681441667734,0.0619700894222737,
27.5043847842334));
#40143=CARTESIAN_POINT('Ctrl Pts',(10.0575586312729,0.230367185062373,27.4794316150452));
#40144=CARTESIAN_POINT('Ctrl Pts',(10.0469730957724,0.382615538030601,27.4158249371804));
#40145=CARTESIAN_POINT('Ctrl Pts',(10.0363875602718,0.534863890998829,27.3522182593157));
#40146=CARTESIAN_POINT('Ctrl Pts',(10.0258020247713,0.670963501295187,27.2499580727743));
#40147=CARTESIAN_POINT('Ctrl Pts',(10.0152164892708,0.774192304741247,27.1212600859187));
#40148=CARTESIAN_POINT('Ctrl Pts',(10.0046309537702,0.877421108187307,26.9925620990631));
#40149=CARTESIAN_POINT('Ctrl Pts',(9.99404541826972,0.94777910478307,26.8374263118932));
#40150=CARTESIAN_POINT('Ctrl Pts',(9.98345988276919,0.976946047547642,26.6750804300979));
#40151=CARTESIAN_POINT('Ctrl Pts',(9.97287434726865,1.00611299031222,26.5127345483026));
#40152=CARTESIAN_POINT('Ctrl Pts',(9.96228881176813,0.994088879245598,26.3431785718819));
#40153=CARTESIAN_POINT('Ctrl Pts',(9.95170327626759,0.941865063348462,26.186540053417));
#40154=CARTESIAN_POINT('Ctrl Pts',(9.94111774076706,0.889641247451325,26.029901534952));
#40155=CARTESIAN_POINT('Ctrl Pts',(9.93053220526652,0.79721772672367,25.8861804744428));
#40156=CARTESIAN_POINT('Ctrl Pts',(9.91994666976599,0.676736285578297,25.7738447556785));
#40157=CARTESIAN_POINT('Ctrl Pts',(9.90936113426546,0.556254844432921,25.6615090369141));
#40158=CARTESIAN_POINT('Ctrl Pts',(9.89877559876493,0.407715482869826,25.5805586598948));
#40159=CARTESIAN_POINT('Ctrl Pts',(9.8881900632644,0.247669345390617,25.5391945047519));
#40160=CARTESIAN_POINT('Ctrl Pts',(9.87760452776387,0.0876232079114112,
25.4978303496091));
#40161=CARTESIAN_POINT('Ctrl Pts',(9.86701899226333,-0.0839297054839095,
25.4960524163428));
#40162=CARTESIAN_POINT('Ctrl Pts',(9.8564334567628,-0.243606213188065,25.5367364336125));
#40163=CARTESIAN_POINT('Ctrl Pts',(9.83526238576173,-0.562959228596377,
25.6181044681518));
#40164=CARTESIAN_POINT('Ctrl Pts',(9.81409131476069,-0.834806621240028,
25.869320304835));
#40165=CARTESIAN_POINT('Ctrl Pts',(9.79292024375962,-0.941079776423611,
26.1812706258213));
#40166=CARTESIAN_POINT('Ctrl Pts',(9.78600242171848,-0.975805406282986,
26.2832029657652));
#40167=CARTESIAN_POINT('Ctrl Pts',(9.77908459967735,-0.992852517217116,
26.3916199844045));
#40168=CARTESIAN_POINT('Ctrl Pts',(9.77216677763621,-0.992506281688296,
26.4999529602842));
#40169=CARTESIAN_POINT('Ctrl Pts',(9.62783322236381,-0.992554123075758,
26.4999819653825));
#40170=CARTESIAN_POINT('Ctrl Pts',(9.62916468447414,-0.99257538731433,26.4792315633208));
#40171=CARTESIAN_POINT('Ctrl Pts',(9.63049614658447,-0.99194025718962,26.4584818294063));
#40172=CARTESIAN_POINT('Ctrl Pts',(9.6318276086948,-0.99064090797148,26.4377730175542));
#40173=CARTESIAN_POINT('Ctrl Pts',(9.64243681159308,-0.980287583318831,
26.27276345024));
#40174=CARTESIAN_POINT('Ctrl Pts',(9.65304601449135,-0.927762739923163,
26.1103520399749));
#40175=CARTESIAN_POINT('Ctrl Pts',(9.66365521738962,-0.839546534340743,
25.970484223423));
#40176=CARTESIAN_POINT('Ctrl Pts',(9.6742644202879,-0.751330328758322,25.830616406871));
#40177=CARTESIAN_POINT('Ctrl Pts',(9.68487362318617,-0.627422760989149,
25.7132921840321));
#40178=CARTESIAN_POINT('Ctrl Pts',(9.69548282608444,-0.482965038876526,
25.6328393738232));
#40179=CARTESIAN_POINT('Ctrl Pts',(9.70609202898271,-0.338507316763903,
25.5523865636142));
#40180=CARTESIAN_POINT('Ctrl Pts',(9.71670123188098,-0.17349944030783,25.5088051660352));
#40181=CARTESIAN_POINT('Ctrl Pts',(9.72731043477925,-0.00814936056770701,
25.5074454729942));
#40182=CARTESIAN_POINT('Ctrl Pts',(9.73791963767753,0.157200719172416,25.5060857799532));
#40183=CARTESIAN_POINT('Ctrl Pts',(9.7485288405758,0.322893002196589,25.5469477914503));
#40184=CARTESIAN_POINT('Ctrl Pts',(9.75913804347408,0.468654544911551,25.6250217681518));
#40185=CARTESIAN_POINT('Ctrl Pts',(9.76974724637235,0.614416087626514,25.7030957448533));
#40186=CARTESIAN_POINT('Ctrl Pts',(9.78035644927062,0.740246890032266,25.8183816867594));
#40187=CARTESIAN_POINT('Ctrl Pts',(9.79096565216889,0.830742853754316,25.9567740422393));
#40188=CARTESIAN_POINT('Ctrl Pts',(9.80157485506716,0.921238817476365,26.0951663977193));
#40189=CARTESIAN_POINT('Ctrl Pts',(9.81218405796544,0.976399942514714,26.2566651667731));
#40190=CARTESIAN_POINT('Ctrl Pts',(9.82279326086371,0.989476757850026,26.4215017995226));
#40191=CARTESIAN_POINT('Ctrl Pts',(9.83340246376199,1.00255357318534,26.5863384322722));
#40192=CARTESIAN_POINT('Ctrl Pts',(9.84401166666025,0.973546078817614,26.7545129287174));
#40193=CARTESIAN_POINT('Ctrl Pts',(9.85462086955853,0.90600360183791,26.9054433464652));
#40194=CARTESIAN_POINT('Ctrl Pts',(9.8652300724568,0.838461124858205,27.056373764213));
#40195=CARTESIAN_POINT('Ctrl Pts',(9.87583927535507,0.73238366526652,27.1900601032633));
#40196=CARTESIAN_POINT('Ctrl Pts',(9.88644847825334,0.600754761208242,27.2901395554777));
#40197=CARTESIAN_POINT('Ctrl Pts',(9.89705768115162,0.469125857149964,27.3902190076921));
#40198=CARTESIAN_POINT('Ctrl Pts',(9.90766688404989,0.311945508625094,27.4566915730705));
#40199=CARTESIAN_POINT('Ctrl Pts',(9.91827608694816,0.148451062000284,27.4814218980271));
#40200=CARTESIAN_POINT('Ctrl Pts',(9.92888528984643,-0.0150433846245255,
27.5061522229836));
#40201=CARTESIAN_POINT('Ctrl Pts',(9.9394944927447,-0.184851929349274,27.4891403075182));
#40202=CARTESIAN_POINT('Ctrl Pts',(9.95010369564298,-0.340191224912641,
27.4324680853709));
#40203=CARTESIAN_POINT('Ctrl Pts',(9.96071289854125,-0.495530520476008,
27.3757958632236));
#40204=CARTESIAN_POINT('Ctrl Pts',(9.97132210143953,-0.636400566877995,
27.2794633343944));
#40205=CARTESIAN_POINT('Ctrl Pts',(9.9819313043378,-0.745560074739528,27.1552609281509));
#40206=CARTESIAN_POINT('Ctrl Pts',(9.99254050723607,-0.854719582601061,
27.0310585219074));
#40207=CARTESIAN_POINT('Ctrl Pts',(10.0031497101343,-0.932168551922139,
26.8789862382495));
#40208=CARTESIAN_POINT('Ctrl Pts',(10.0137589130326,-0.968427809645741,
26.7176564531269));
#40209=CARTESIAN_POINT('Ctrl Pts',(10.0184503494763,-0.984461813777658,
26.6463157086204));
#40210=CARTESIAN_POINT('Ctrl Pts',(10.0231417859201,-0.992441385989991,
26.5731647082902));
#40211=CARTESIAN_POINT('Ctrl Pts',(10.0278332223638,-0.992418708717116,
26.5000088356422));
#40212=CARTESIAN_POINT('Origin',(18.,0.,26.5));
#40213=CARTESIAN_POINT('',(10.5721667776362,-0.992503945737967,26.5001013395173));
#40214=CARTESIAN_POINT('',(10.4278332223638,-0.992585626431949,26.5000017565761));
#40215=CARTESIAN_POINT('',(18.,-0.9925,26.5));
#40216=CARTESIAN_POINT('Ctrl Pts',(10.5721667776362,-0.992503945737967,
26.5001013395173));
#40217=CARTESIAN_POINT('Ctrl Pts',(10.5664707850234,-0.992439806685457,
26.5888593811617));
#40218=CARTESIAN_POINT('Ctrl Pts',(10.5607747924107,-0.980556995371912,
26.67759125854));
#40219=CARTESIAN_POINT('Ctrl Pts',(10.5550787997979,-0.956986725286291,
26.7631600087317));
#40220=CARTESIAN_POINT('Ctrl Pts',(10.5444932642974,-0.913183309848331,
26.9221825188488));
#40221=CARTESIAN_POINT('Ctrl Pts',(10.5339077287969,-0.829014711658026,
27.0702804807433));
#40222=CARTESIAN_POINT('Ctrl Pts',(10.5233221932963,-0.714514616847861,
27.1890621572086));
#40223=CARTESIAN_POINT('Ctrl Pts',(10.5127366577958,-0.600014522037695,
27.3078438336738));
#40224=CARTESIAN_POINT('Ctrl Pts',(10.5021511222953,-0.455182930607668,
27.3973092247099));
#40225=CARTESIAN_POINT('Ctrl Pts',(10.4915655867947,-0.297783039914208,
27.4468132006782));
#40226=CARTESIAN_POINT('Ctrl Pts',(10.4809800512942,-0.140383149220748,
27.4963171766466));
#40227=CARTESIAN_POINT('Ctrl Pts',(10.4703945157937,0.029585040736145,27.5058597375472));
#40228=CARTESIAN_POINT('Ctrl Pts',(10.4598089802931,0.191462890804785,27.4740019279372));
#40229=CARTESIAN_POINT('Ctrl Pts',(10.4492234447926,0.353340740873424,27.4421441183272));
#40230=CARTESIAN_POINT('Ctrl Pts',(10.4386379092921,0.507128251053811,27.3688859382066));
#40231=CARTESIAN_POINT('Ctrl Pts',(10.4280523737915,0.634070607296442,27.2635648286469));
#40232=CARTESIAN_POINT('Ctrl Pts',(10.417466838291,0.761012963539074,27.1582437190873));
#40233=CARTESIAN_POINT('Ctrl Pts',(10.4068813027905,0.861110165843951,27.0208596800887));
#40234=CARTESIAN_POINT('Ctrl Pts',(10.3962957672899,0.922146658222156,26.8674403530521));
#40235=CARTESIAN_POINT('Ctrl Pts',(10.3857102317894,0.983183150600361,26.7140210260155));
#40236=CARTESIAN_POINT('Ctrl Pts',(10.3751246962889,1.00515893305189,26.5445664109409));
#40237=CARTESIAN_POINT('Ctrl Pts',(10.3645391607883,0.985453047942944,26.3810219498978));
#40238=CARTESIAN_POINT('Ctrl Pts',(10.3539536252878,0.965747162833992,26.2174774888548));
#40239=CARTESIAN_POINT('Ctrl Pts',(10.3433680897873,0.904359610164555,26.0598431818432));
#40240=CARTESIAN_POINT('Ctrl Pts',(10.3327825542867,0.80865874018317,25.9250578875996));
#40241=CARTESIAN_POINT('Ctrl Pts',(10.3221970187862,0.712957870201786,25.790272593356));
#40242=CARTESIAN_POINT('Ctrl Pts',(10.3116114832857,0.582943682908454,25.6783363118803));
#40243=CARTESIAN_POINT('Ctrl Pts',(10.3010259477851,0.434639808109102,25.6065189153853));
#40244=CARTESIAN_POINT('Ctrl Pts',(10.2798548767841,0.138032058510397,25.4628841223952));
#40245=CARTESIAN_POINT('Ctrl Pts',(10.258683805783,-0.231734441112391,25.479724869328));
#40246=CARTESIAN_POINT('Ctrl Pts',(10.237512734782,-0.514057839417016,25.6497266620276));
#40247=CARTESIAN_POINT('Ctrl Pts',(10.2269271992814,-0.655219538569327,
25.7347275583773));
#40248=CARTESIAN_POINT('Ctrl Pts',(10.2163416637809,-0.774520462392098,
25.8580187161688));
#40249=CARTESIAN_POINT('Ctrl Pts',(10.2057561282804,-0.857573150452479,
26.000945211532));
#40250=CARTESIAN_POINT('Ctrl Pts',(10.1951705927798,-0.94062583851286,26.1438717068953));
#40251=CARTESIAN_POINT('Ctrl Pts',(10.1845850572793,-0.987430290810851,
26.3064335398303));
#40252=CARTESIAN_POINT('Ctrl Pts',(10.1739995217788,-0.992188402394096,
26.4710921961006));
#40253=CARTESIAN_POINT('Ctrl Pts',(10.1733886070646,-0.992463003558845,
26.4805950120826));
#40254=CARTESIAN_POINT('Ctrl Pts',(10.1727776923504,-0.992597560980474,
26.490104811954));
#40255=CARTESIAN_POINT('Ctrl Pts',(10.1721667776362,-0.992592959832253,
26.4996174405759));
#40256=CARTESIAN_POINT('Ctrl Pts',(10.0278332223638,-0.992418708717116,
26.5000088356422));
#40257=CARTESIAN_POINT('Ctrl Pts',(10.0337509888184,-0.992390103660582,
26.4077301968285));
#40258=CARTESIAN_POINT('Ctrl Pts',(10.0396687552729,-0.979628929082159,
26.315443805554));
#40259=CARTESIAN_POINT('Ctrl Pts',(10.0455865217274,-0.95423991719696,26.2267731381084));
#40260=CARTESIAN_POINT('Ctrl Pts',(10.0561957246257,-0.908723220898453,
26.0678068947998));
#40261=CARTESIAN_POINT('Ctrl Pts',(10.066804927524,-0.822620282175313,25.92046169477));
#40262=CARTESIAN_POINT('Ctrl Pts',(10.0774141304222,-0.7064693994913,25.8027713948326));
#40263=CARTESIAN_POINT('Ctrl Pts',(10.0880233333205,-0.590318516807288,
25.6850810948951));
#40264=CARTESIAN_POINT('Ctrl Pts',(10.0986325362188,-0.444119690162403,
25.5970456950502));
#40265=CARTESIAN_POINT('Ctrl Pts',(10.1092417391171,-0.28576649020178,25.5494400305557));
#40266=CARTESIAN_POINT('Ctrl Pts',(10.1198509420153,-0.127413290241156,
25.5018343660612));
#40267=CARTESIAN_POINT('Ctrl Pts',(10.1304601449136,0.0430942830352055,
25.4946584369172));
#40268=CARTESIAN_POINT('Ctrl Pts',(10.1410693478119,0.204887472275318,25.5287905151852));
#40269=CARTESIAN_POINT('Ctrl Pts',(10.1516785507101,0.366680661515429,25.5629225934533));
#40270=CARTESIAN_POINT('Ctrl Pts',(10.1622877536084,0.519759466719291,25.6383626791333));
#40271=CARTESIAN_POINT('Ctrl Pts',(10.1728969565067,0.645388267268235,25.7458775125298));
#40272=CARTESIAN_POINT('Ctrl Pts',(10.183506159405,0.77101706781718,25.8533923459262));
#40273=CARTESIAN_POINT('Ctrl Pts',(10.1941153623032,0.869195863711207,25.9929819270389));
#40274=CARTESIAN_POINT('Ctrl Pts',(10.2047245652015,0.927908358035644,26.1475616086697));
#40275=CARTESIAN_POINT('Ctrl Pts',(10.2153337680998,0.986620852360081,26.3021412903005));
#40276=CARTESIAN_POINT('Ctrl Pts',(10.2259429709981,1.00586704511493,26.4717110724493));
#40277=CARTESIAN_POINT('Ctrl Pts',(10.2365521738963,0.983291356083112,26.6355169733609));
#40278=CARTESIAN_POINT('Ctrl Pts',(10.2471613767946,0.960715667051297,26.7993228742725));
#40279=CARTESIAN_POINT('Ctrl Pts',(10.2577705796929,0.896318096232822,26.9573648939469));
#40280=CARTESIAN_POINT('Ctrl Pts',(10.2683797825912,0.797980390449239,27.0902999554258));
#40281=CARTESIAN_POINT('Ctrl Pts',(10.2789889854894,0.699642684665656,27.2232350169047));
#40282=CARTESIAN_POINT('Ctrl Pts',(10.2895981883877,0.567364843916966,27.331063120188));
#40283=CARTESIAN_POINT('Ctrl Pts',(10.300207391286,0.417336615681909,27.4005869697607));
#40284=CARTESIAN_POINT('Ctrl Pts',(10.3108165941842,0.267308387446851,27.4701108193334));
#40285=CARTESIAN_POINT('Ctrl Pts',(10.3214257970825,0.0995297717254275,
27.5013304151955));
#40286=CARTESIAN_POINT('Ctrl Pts',(10.3320349999808,-0.0654644734564326,
27.4904247289211));
#40287=CARTESIAN_POINT('Ctrl Pts',(10.3426442028791,-0.230458718638292,
27.4795190426466));
#40288=CARTESIAN_POINT('Ctrl Pts',(10.3532534057773,-0.392668593280588,
27.4264880742357));
#40289=CARTESIAN_POINT('Ctrl Pts',(10.3638626086756,-0.532240908742537,
27.3378223892708));
#40290=CARTESIAN_POINT('Ctrl Pts',(10.3744718115739,-0.671813224204487,
27.2491567043058));
#40291=CARTESIAN_POINT('Ctrl Pts',(10.3850810144721,-0.788747980486091,
27.1248563027868));
#40292=CARTESIAN_POINT('Ctrl Pts',(10.3956902173704,-0.868733300534966,
26.9801345576685));
#40293=CARTESIAN_POINT('Ctrl Pts',(10.4062994202687,-0.94871862058384,26.8354128125502));
#40294=CARTESIAN_POINT('Ctrl Pts',(10.416908623167,-0.991754504399986,26.6702697238326));
#40295=CARTESIAN_POINT('Ctrl Pts',(10.4275178260652,-0.992573704711812,
26.5049174821022));
#40296=CARTESIAN_POINT('Ctrl Pts',(10.4276229581648,-0.992581822593009,
26.5032789208926));
#40297=CARTESIAN_POINT('Ctrl Pts',(10.4277280902643,-0.992585794856245,
26.5016403391444));
#40298=CARTESIAN_POINT('Ctrl Pts',(10.4278332223638,-0.992585626431949,
26.5000017565761));
#40299=CARTESIAN_POINT('Origin',(18.,0.,26.5));
#40300=CARTESIAN_POINT('',(10.9721667776362,-0.9925,26.5));
#40301=CARTESIAN_POINT('',(10.8278332223638,-0.992422357680272,26.4999883264764));
#40302=CARTESIAN_POINT('',(18.,-0.9925,26.5));
#40303=CARTESIAN_POINT('Ctrl Pts',(10.9721667776362,-0.992583538475113,
26.5000383753598));
#40304=CARTESIAN_POINT('Ctrl Pts',(10.970749413197,-0.992612646059146,26.5221334010504));
#40305=CARTESIAN_POINT('Ctrl Pts',(10.9693320487579,-0.991897265306533,
26.5442263779092));
#40306=CARTESIAN_POINT('Ctrl Pts',(10.9679146843187,-0.990427353666401,
26.5662680261881));
#40307=CARTESIAN_POINT('Ctrl Pts',(10.9573291488181,-0.979449371279416,
26.7308852861515));
#40308=CARTESIAN_POINT('Ctrl Pts',(10.9467436133176,-0.926385197682136,
26.8926395428142));
#40309=CARTESIAN_POINT('Ctrl Pts',(10.9361580778171,-0.837954139517956,
27.0319425118404));
#40310=CARTESIAN_POINT('Ctrl Pts',(10.9255725423166,-0.749523081353776,
27.1712454808666));
#40311=CARTESIAN_POINT('Ctrl Pts',(10.914987006816,-0.625725138622696,27.2880971622564));
#40312=CARTESIAN_POINT('Ctrl Pts',(10.9044014713155,-0.48142731992349,27.3680815225639));
#40313=CARTESIAN_POINT('Ctrl Pts',(10.8938159358149,-0.337129501224285,
27.4480658828714));
#40314=CARTESIAN_POINT('Ctrl Pts',(10.8832304003144,-0.172331806556954,
27.4911829220966));
#40315=CARTESIAN_POINT('Ctrl Pts',(10.8726448648139,-0.00739179261613836,
27.4924828179735));
#40316=CARTESIAN_POINT('Ctrl Pts',(10.8620593293134,0.157548221324677,27.4937827138503));
#40317=CARTESIAN_POINT('Ctrl Pts',(10.8514737938128,0.322630554538978,27.4532654663788));
#40318=CARTESIAN_POINT('Ctrl Pts',(10.8408882583123,0.468184939661327,27.3753112215794));
#40319=CARTESIAN_POINT('Ctrl Pts',(10.8303027228118,0.613739324783676,27.29735697678));
#40320=CARTESIAN_POINT('Ctrl Pts',(10.8197171873112,0.739765761814074,27.1819657346527));
#40321=CARTESIAN_POINT('Ctrl Pts',(10.8091316518107,0.830115089366124,27.0442264459477));
#40322=CARTESIAN_POINT('Ctrl Pts',(10.7985461163102,0.920464416918174,26.9064871572428));
#40323=CARTESIAN_POINT('Ctrl Pts',(10.7879605808096,0.975136634991876,26.7463998219603));
#40324=CARTESIAN_POINT('Ctrl Pts',(10.7773750453091,0.988846963069828,26.581664400842));
#40325=CARTESIAN_POINT('Ctrl Pts',(10.7667895098086,1.00255729114778,26.4169289797236));
#40326=CARTESIAN_POINT('Ctrl Pts',(10.756203974308,0.975305729229982,26.2475454727695));
#40327=CARTESIAN_POINT('Ctrl Pts',(10.7456184388075,0.908211509398971,26.097045826974));
#40328=CARTESIAN_POINT('Ctrl Pts',(10.7244473678064,0.774023069736951,25.7960465353831));
#40329=CARTESIAN_POINT('Ctrl Pts',(10.7032762968054,0.480463998422085,25.5705826884271));
#40330=CARTESIAN_POINT('Ctrl Pts',(10.6821052258043,0.155036732944931,25.5185807099911));
#40331=CARTESIAN_POINT('Ctrl Pts',(10.6715196903038,-0.00767689979364622,
25.4925797207731));
#40332=CARTESIAN_POINT('Ctrl Pts',(10.6609341548032,-0.178357581072796,
25.5099441986851));
#40333=CARTESIAN_POINT('Ctrl Pts',(10.6503486193027,-0.333981058544879,
25.5656852547077));
#40334=CARTESIAN_POINT('Ctrl Pts',(10.6397630838022,-0.489604536016962,
25.6214263107303));
#40335=CARTESIAN_POINT('Ctrl Pts',(10.6291775483016,-0.630170809681978,
25.7155439448637));
#40336=CARTESIAN_POINT('Ctrl Pts',(10.6185920128011,-0.739942200305901,
25.8383663957533));
#40337=CARTESIAN_POINT('Ctrl Pts',(10.6080064773006,-0.849713590929822,
25.961188846643));
#40338=CARTESIAN_POINT('Ctrl Pts',(10.5974209418001,-0.928690098512649,
26.1127161142891));
#40339=CARTESIAN_POINT('Ctrl Pts',(10.5868354062995,-0.966459235961256,
26.273453277282));
#40340=CARTESIAN_POINT('Ctrl Pts',(10.5819458634118,-0.983905100403322,
26.3476990489836));
#40341=CARTESIAN_POINT('Ctrl Pts',(10.577056320524,-0.992559003858536,26.423909834233));
#40342=CARTESIAN_POINT('Ctrl Pts',(10.5721667776362,-0.992503945737967,
26.5001013395173));
#40343=CARTESIAN_POINT('Ctrl Pts',(10.4278332223638,-0.992585626431949,
26.5000017565761));
#40344=CARTESIAN_POINT('Ctrl Pts',(10.4383372931626,-0.992568798643581,
26.3362859420382));
#40345=CARTESIAN_POINT('Ctrl Pts',(10.4488413639613,-0.951217054403849,
26.1725619396382));
#40346=CARTESIAN_POINT('Ctrl Pts',(10.4593454347601,-0.873447975304868,
26.028496685744));
#40347=CARTESIAN_POINT('Ctrl Pts',(10.4699546376583,-0.794900528778586,
25.8829895258591));
#40348=CARTESIAN_POINT('Ctrl Pts',(10.4805638405566,-0.679203118918512,
25.7575366008324));
#40349=CARTESIAN_POINT('Ctrl Pts',(10.4911730434549,-0.540516181474807,
25.6674923432889));
#40350=CARTESIAN_POINT('Ctrl Pts',(10.5017822463531,-0.401829244031103,
25.5774480857455));
#40351=CARTESIAN_POINT('Ctrl Pts',(10.5123914492514,-0.24015277900377,25.5228124956853));
#40352=CARTESIAN_POINT('Ctrl Pts',(10.5230006521497,-0.0752746900067089,
25.5102725314703));
#40353=CARTESIAN_POINT('Ctrl Pts',(10.533609855048,0.0896033989903517,25.4977325672554));
#40354=CARTESIAN_POINT('Ctrl Pts',(10.5442190579462,0.257683111957139,25.5272882288857));
#40355=CARTESIAN_POINT('Ctrl Pts',(10.5548282608445,0.408392839046391,25.5953221402432));
#40356=CARTESIAN_POINT('Ctrl Pts',(10.5654374637428,0.559102566135641,25.6633560516006));
#40357=CARTESIAN_POINT('Ctrl Pts',(10.5760466666411,0.692442307347355,25.7698682126851));
#40358=CARTESIAN_POINT('Ctrl Pts',(10.5866558695393,0.792092346966023,25.9018223885868));
#40359=CARTESIAN_POINT('Ctrl Pts',(10.5972650724376,0.891742386584692,26.0337765644886));
#40360=CARTESIAN_POINT('Ctrl Pts',(10.6078742753359,0.957702724610315,26.1911727552075));
#40361=CARTESIAN_POINT('Ctrl Pts',(10.6184834782341,0.981900344286195,26.3547469284009));
#40362=CARTESIAN_POINT('Ctrl Pts',(10.6290926811324,1.00609796396208,26.5183211015943));
#40363=CARTESIAN_POINT('Ctrl Pts',(10.6397018840307,0.988532865288214,26.6880732572622));
#40364=CARTESIAN_POINT('Ctrl Pts',(10.650311086929,0.93135487557259,26.8432270919747));
#40365=CARTESIAN_POINT('Ctrl Pts',(10.6609202898272,0.874176885856967,26.9983809266871));
#40366=CARTESIAN_POINT('Ctrl Pts',(10.6715294927255,0.777386005099581,27.1389364404442));
#40367=CARTESIAN_POINT('Ctrl Pts',(10.6821386956238,0.652828661405759,27.2476907647988));
#40368=CARTESIAN_POINT('Ctrl Pts',(10.6927478985221,0.528271317711936,27.3564450891534));
#40369=CARTESIAN_POINT('Ctrl Pts',(10.7033571014203,0.375947511081676,27.4333982241057));
#40370=CARTESIAN_POINT('Ctrl Pts',(10.7139663043186,0.214500454696508,27.4691317226535));
#40371=CARTESIAN_POINT('Ctrl Pts',(10.7245755072169,0.0530533983113431,
27.5048652212012));
#40372=CARTESIAN_POINT('Ctrl Pts',(10.7351847101151,-0.11751690782873,27.4993790833445));
#40373=CARTESIAN_POINT('Ctrl Pts',(10.7457939130134,-0.27633402523292,27.4533447683901));
#40374=CARTESIAN_POINT('Ctrl Pts',(10.7564031159117,-0.43515114263711,27.4073104534357));
#40375=CARTESIAN_POINT('Ctrl Pts',(10.76701231881,-0.582215071305418,27.3207279613836));
#40376=CARTESIAN_POINT('Ctrl Pts',(10.7776215217082,-0.699526364965285,
27.2041942953736));
#40377=CARTESIAN_POINT('Ctrl Pts',(10.7882307246065,-0.816837658625152,
27.0876606293635));
#40378=CARTESIAN_POINT('Ctrl Pts',(10.7988399275048,-0.904396317276578,
26.9411757893955));
#40379=CARTESIAN_POINT('Ctrl Pts',(10.809449130403,-0.951485862811279,26.782668345926));
#40380=CARTESIAN_POINT('Ctrl Pts',(10.8155771610566,-0.978685472552665,
26.6911121299014));
#40381=CARTESIAN_POINT('Ctrl Pts',(10.8217051917102,-0.992383022265051,
26.5955447087458));
#40382=CARTESIAN_POINT('Ctrl Pts',(10.8278332223638,-0.992422357680272,
26.4999883264764));
#40383=CARTESIAN_POINT('Origin',(18.,0.,26.5));
#40384=CARTESIAN_POINT('',(11.3721667776362,-0.9925,26.5));
#40385=CARTESIAN_POINT('',(11.2278332223638,-0.992543914931681,26.5000214785174));
#40386=CARTESIAN_POINT('',(18.,-0.9925,26.5));
#40387=CARTESIAN_POINT('Ctrl Pts',(11.3721667776362,-0.9925,26.5));
#40388=CARTESIAN_POINT('Ctrl Pts',(11.3554259338597,-0.992500000000001,
26.7609923249229));
#40389=CARTESIAN_POINT('Ctrl Pts',(11.3386850900831,-0.884539443097409,
27.0203491301747));
#40390=CARTESIAN_POINT('Ctrl Pts',(11.3219442463066,-0.699346033936908,
27.2042523516586));
#40391=CARTESIAN_POINT('Ctrl Pts',(11.3052034025301,-0.514152624776407,
27.3881555731426));
#40392=CARTESIAN_POINT('Ctrl Pts',(11.2884625587535,-0.254047408344448,
27.4943003359057));
#40393=CARTESIAN_POINT('Ctrl Pts',(11.271721714977,0.00693853867348876,
27.4924757461425));
#40394=CARTESIAN_POINT('Ctrl Pts',(11.2549808712005,0.267924485691426,27.4906511563793));
#40395=CARTESIAN_POINT('Ctrl Pts',(11.238240027424,0.52652020388806,27.3808800818309));
#40396=CARTESIAN_POINT('Ctrl Pts',(11.2214991836474,0.709124249559321,27.1944055361868));
#40397=CARTESIAN_POINT('Ctrl Pts',(11.2047583398709,0.891728295230581,27.0079309905428));
#40398=CARTESIAN_POINT('Ctrl Pts',(11.1880174960943,0.996052076106193,26.7470900753838));
#40399=CARTESIAN_POINT('Ctrl Pts',(11.1712766523178,0.992402985755318,26.486123261769));
#40400=CARTESIAN_POINT('Ctrl Pts',(11.1545358085413,0.988753895404444,26.2251564481542));
#40401=CARTESIAN_POINT('Ctrl Pts',(11.1377949647647,0.877177668191511,25.9673344556903));
#40402=CARTESIAN_POINT('Ctrl Pts',(11.1210541209882,0.689431099871663,25.7860385104715));
#40403=CARTESIAN_POINT('Ctrl Pts',(11.1043132772117,0.501684531551814,25.6047425652527));
#40404=CARTESIAN_POINT('Ctrl Pts',(11.0875724334351,0.240120666075684,25.5022448650135));
#40405=CARTESIAN_POINT('Ctrl Pts',(11.0708315896586,-0.0208142595729385,
25.5077182776054));
#40406=CARTESIAN_POINT('Ctrl Pts',(11.0540907458821,-0.281749185221561,
25.5131916901973));
#40407=CARTESIAN_POINT('Ctrl Pts',(11.0373499021056,-0.538784851090619,
25.6265676168678));
#40408=CARTESIAN_POINT('Ctrl Pts',(11.020609058329,-0.718763835149583,25.8155770318867));
#40409=CARTESIAN_POINT('Ctrl Pts',(11.0044616314314,-0.892363059118819,
25.9978865828696));
#40410=CARTESIAN_POINT('Ctrl Pts',(10.9883142045338,-0.9925,26.248259135335));
#40411=CARTESIAN_POINT('Ctrl Pts',(10.9721667776362,-0.9925,26.5));
#40412=CARTESIAN_POINT('Ctrl Pts',(10.8278332223638,-0.992422357680272,
26.4999883264764));
#40413=CARTESIAN_POINT('Ctrl Pts',(10.8323143946085,-0.992451122022502,
26.4301119449382));
#40414=CARTESIAN_POINT('Ctrl Pts',(10.8367955668532,-0.985176313957699,
26.360241466317));
#40415=CARTESIAN_POINT('Ctrl Pts',(10.8412767390979,-0.970536872194566,
26.2919497161044));
#40416=CARTESIAN_POINT('Ctrl Pts',(10.8518859419961,-0.935877903625177,
26.1302685767232));
#40417=CARTESIAN_POINT('Ctrl Pts',(10.8624951448944,-0.859939534068422,
25.9774363449317));
#40418=CARTESIAN_POINT('Ctrl Pts',(10.8731043477927,-0.752016011374463,
25.8521584610766));
#40419=CARTESIAN_POINT('Ctrl Pts',(10.883713550691,-0.644092488680505,25.7268805772214));
#40420=CARTESIAN_POINT('Ctrl Pts',(10.8943227535892,-0.504183812849344,
25.6291570413026));
#40421=CARTESIAN_POINT('Ctrl Pts',(10.9049319564875,-0.34941368454973,25.5709484309428));
#40422=CARTESIAN_POINT('Ctrl Pts',(10.9155411593858,-0.194643556250115,
25.512739820583));
#40423=CARTESIAN_POINT('Ctrl Pts',(10.926150362284,-0.0250119754820468,
25.4940461357822));
#40424=CARTESIAN_POINT('Ctrl Pts',(10.9367595651823,0.138719511726088,25.5171553337456));
#40425=CARTESIAN_POINT('Ctrl Pts',(10.9473687680806,0.302450998934223,25.540264531709));
#40426=CARTESIAN_POINT('Ctrl Pts',(10.9579779709789,0.460282392582425,25.6051766124364));
#40427=CARTESIAN_POINT('Ctrl Pts',(10.9685871738771,0.592896394976983,25.7039468574639));
#40428=CARTESIAN_POINT('Ctrl Pts',(10.9791963767754,0.72551039737154,25.8027171024914));
#40429=CARTESIAN_POINT('Ctrl Pts',(10.9898055796737,0.832907008512454,25.935345511819));
#40430=CARTESIAN_POINT('Ctrl Pts',(11.0004147825719,0.901941743891598,26.0855994310525));
#40431=CARTESIAN_POINT('Ctrl Pts',(11.0110239854702,0.970976479270744,26.235853350286));
#40432=CARTESIAN_POINT('Ctrl Pts',(11.0216331883685,1.00164933888812,26.4037327794254));
#40433=CARTESIAN_POINT('Ctrl Pts',(11.0322423912668,0.990206210544303,26.5686906217598));
#40434=CARTESIAN_POINT('Ctrl Pts',(11.042851594165,0.978763082200488,26.7336484640941));
#40435=CARTESIAN_POINT('Ctrl Pts',(11.0534607970633,0.925203965895484,26.8956847196234));
#40436=CARTESIAN_POINT('Ctrl Pts',(11.0640699999616,0.836084068232749,27.034967449258));
#40437=CARTESIAN_POINT('Ctrl Pts',(11.0746792028599,0.746964170570011,27.1742501788927));
#40438=CARTESIAN_POINT('Ctrl Pts',(11.0852884057581,0.622283491549541,27.2907793826328));
#40439=CARTESIAN_POINT('Ctrl Pts',(11.0958976086564,0.477301947070334,27.3702928198262));
#40440=CARTESIAN_POINT('Ctrl Pts',(11.1065068115547,0.332320402591129,27.4498062570197));
#40441=CARTESIAN_POINT('Ctrl Pts',(11.1171160144529,0.167037992653186,27.4923039276666));
#40442=CARTESIAN_POINT('Ctrl Pts',(11.1277252173512,0.00168395963031208,
27.4925844574636));
#40443=CARTESIAN_POINT('Ctrl Pts',(11.1383344202495,-0.163670073392562,
27.4928649872605));
#40444=CARTESIAN_POINT('Ctrl Pts',(11.1489436231478,-0.329095729500368,
27.4509283762076));
#40445=CARTESIAN_POINT('Ctrl Pts',(11.159552826046,-0.474346234136107,27.3719073294102));
#40446=CARTESIAN_POINT('Ctrl Pts',(11.1701620289443,-0.619596738771846,
27.2928862826127));
#40447=CARTESIAN_POINT('Ctrl Pts',(11.1807712318426,-0.744672091935519,
27.1767808000708));
#40448=CARTESIAN_POINT('Ctrl Pts',(11.1913804347409,-0.834264072775994,
27.0378012623576));
#40449=CARTESIAN_POINT('Ctrl Pts',(11.2019896376391,-0.92385605361647,26.8988217246444));
#40450=CARTESIAN_POINT('Ctrl Pts',(11.2125988405374,-0.977964662133747,
26.7369681317599));
#40451=CARTESIAN_POINT('Ctrl Pts',(11.2232080434357,-0.989967438281312,
26.5720500663497));
#40452=CARTESIAN_POINT('Ctrl Pts',(11.224749769745,-0.991711678253884,26.5480842205861));
#40453=CARTESIAN_POINT('Ctrl Pts',(11.2262914960544,-0.992566734892839,
26.5240536598473));
#40454=CARTESIAN_POINT('Ctrl Pts',(11.2278332223638,-0.992543914931681,
26.5000214785174));
#40455=CARTESIAN_POINT('Origin',(18.,0.,26.5));
#40456=CARTESIAN_POINT('',(11.7721667776362,-0.992366447419476,26.5000655238227));
#40457=CARTESIAN_POINT('',(11.6278332223638,-0.992471224471742,26.4999749790724));
#40458=CARTESIAN_POINT('',(18.,-0.9925,26.5));
#40459=CARTESIAN_POINT('Ctrl Pts',(11.7721667776362,-0.9925,26.5));
#40460=CARTESIAN_POINT('Ctrl Pts',(11.7554259338597,-0.992499999999996,
26.7609923249229));
#40461=CARTESIAN_POINT('Ctrl Pts',(11.7386850900831,-0.8845394430974,27.0203491301747));
#40462=CARTESIAN_POINT('Ctrl Pts',(11.7219442463066,-0.699346033936895,
27.2042523516586));
#40463=CARTESIAN_POINT('Ctrl Pts',(11.7052034025301,-0.514152624776391,
27.3881555731426));
#40464=CARTESIAN_POINT('Ctrl Pts',(11.6884625587535,-0.25404740834443,27.4943003359057));
#40465=CARTESIAN_POINT('Ctrl Pts',(11.671721714977,0.00693853867350669,
27.4924757461425));
#40466=CARTESIAN_POINT('Ctrl Pts',(11.6549808712005,0.267924485691444,27.4906511563793));
#40467=CARTESIAN_POINT('Ctrl Pts',(11.6382400274239,0.526520203888076,27.3808800818308));
#40468=CARTESIAN_POINT('Ctrl Pts',(11.6214991836474,0.709124249559333,27.1944055361868));
#40469=CARTESIAN_POINT('Ctrl Pts',(11.6047583398709,0.89172829523059,27.0079309905428));
#40470=CARTESIAN_POINT('Ctrl Pts',(11.5880174960943,0.996052076106197,26.7470900753838));
#40471=CARTESIAN_POINT('Ctrl Pts',(11.5712766523178,0.992402985755318,26.486123261769));
#40472=CARTESIAN_POINT('Ctrl Pts',(11.5545358085413,0.988753895404439,26.2251564481542));
#40473=CARTESIAN_POINT('Ctrl Pts',(11.5377949647647,0.877177668191501,25.9673344556903));
#40474=CARTESIAN_POINT('Ctrl Pts',(11.5210541209882,0.68943109987165,25.7860385104715));
#40475=CARTESIAN_POINT('Ctrl Pts',(11.5043132772117,0.501684531551798,25.6047425652527));
#40476=CARTESIAN_POINT('Ctrl Pts',(11.4875724334351,0.240120666075666,25.5022448650134));
#40477=CARTESIAN_POINT('Ctrl Pts',(11.4708315896586,-0.0208142595729564,
25.5077182776054));
#40478=CARTESIAN_POINT('Ctrl Pts',(11.4540907458821,-0.281749185221578,
25.5131916901973));
#40479=CARTESIAN_POINT('Ctrl Pts',(11.4373499021055,-0.538784851090635,
25.6265676168679));
#40480=CARTESIAN_POINT('Ctrl Pts',(11.420609058329,-0.718763835149595,25.8155770318867));
#40481=CARTESIAN_POINT('Ctrl Pts',(11.4044616314314,-0.892363059118823,
25.9978865828696));
#40482=CARTESIAN_POINT('Ctrl Pts',(11.3883142045338,-0.9925,26.248259135335));
#40483=CARTESIAN_POINT('Ctrl Pts',(11.3721667776362,-0.9925,26.5));
#40484=CARTESIAN_POINT('Ctrl Pts',(11.2278332223638,-0.992543914931681,
26.5000214785174));
#40485=CARTESIAN_POINT('Ctrl Pts',(11.2369006989527,-0.992409702093583,
26.3586791142707));
#40486=CARTESIAN_POINT('Ctrl Pts',(11.2459681755416,-0.961909195313563,
26.217280692776));
#40487=CARTESIAN_POINT('Ctrl Pts',(11.2550356521305,-0.903342642445217,
26.0886621689434));
#40488=CARTESIAN_POINT('Ctrl Pts',(11.2656448550288,-0.834818126683708,
25.9381748748832));
#40489=CARTESIAN_POINT('Ctrl Pts',(11.276254057927,-0.727872151382838,25.8051828246989));
#40490=CARTESIAN_POINT('Ctrl Pts',(11.2868632608253,-0.595594046835387,
25.7059631795109));
#40491=CARTESIAN_POINT('Ctrl Pts',(11.2974724637236,-0.463315942287936,
25.6067435343229));
#40492=CARTESIAN_POINT('Ctrl Pts',(11.3080816666219,-0.305705708493902,
25.5412962941313));
#40493=CARTESIAN_POINT('Ctrl Pts',(11.3186908695201,-0.142053574953264,
25.5176316766298));
#40494=CARTESIAN_POINT('Ctrl Pts',(11.3293000724184,0.0215985585873745,
25.4939670591282));
#40495=CARTESIAN_POINT('Ctrl Pts',(11.3399092753167,0.191292591874618,25.5120850643167));
#40496=CARTESIAN_POINT('Ctrl Pts',(11.3505184782149,0.346259335192242,25.5697681935611));
#40497=CARTESIAN_POINT('Ctrl Pts',(11.3611276811132,0.501226078509868,25.6274513228055));
#40498=CARTESIAN_POINT('Ctrl Pts',(11.3717368840115,0.641465531857871,25.7246995761059));
#40499=CARTESIAN_POINT('Ctrl Pts',(11.3823460869098,0.749813510050352,25.8496105466229));
#40500=CARTESIAN_POINT('Ctrl Pts',(11.392955289808,0.858161488242832,25.9745215171399));
#40501=CARTESIAN_POINT('Ctrl Pts',(11.4035644927063,0.934617991279787,26.1270952048736));
#40502=CARTESIAN_POINT('Ctrl Pts',(11.4141736956046,0.969825355925495,26.288657813198));
#40503=CARTESIAN_POINT('Ctrl Pts',(11.4247828985028,1.0050327205712,26.4502204215225));
#40504=CARTESIAN_POINT('Ctrl Pts',(11.4353921014011,0.998990946825663,26.6207719504377));
#40505=CARTESIAN_POINT('Ctrl Pts',(11.4460013042994,0.952439499375482,26.7794382596347));
#40506=CARTESIAN_POINT('Ctrl Pts',(11.4566105071977,0.9058880519253,26.9381045688316));
#40507=CARTESIAN_POINT('Ctrl Pts',(11.4672197100959,0.818826930770477,27.0848856583103));
#40508=CARTESIAN_POINT('Ctrl Pts',(11.4778289129942,0.70191171941707,27.2018166990484));
#40509=CARTESIAN_POINT('Ctrl Pts',(11.4884381158925,0.584996508063663,27.3187477397865));
#40510=CARTESIAN_POINT('Ctrl Pts',(11.4990473187907,0.438227206511674,27.4058287317839));
#40511=CARTESIAN_POINT('Ctrl Pts',(11.509656521689,0.279567201035806,27.4524016595026));
#40512=CARTESIAN_POINT('Ctrl Pts',(11.5202657245873,0.120907195559937,27.4989745872213));
#40513=CARTESIAN_POINT('Ctrl Pts',(11.5308749274856,-0.0496435138398082,
27.5050394506614));
#40514=CARTESIAN_POINT('Ctrl Pts',(11.5414841303839,-0.211210887156589,
27.4698539591427));
#40515=CARTESIAN_POINT('Ctrl Pts',(11.5520933332821,-0.372778260473371,
27.434668467624));
#40516=CARTESIAN_POINT('Ctrl Pts',(11.5627025361804,-0.52536229770719,27.3582326211465));
#40517=CARTESIAN_POINT('Ctrl Pts',(11.5733117390787,-0.650287935536204,
27.2499015547486));
#40518=CARTESIAN_POINT('Ctrl Pts',(11.5839209419769,-0.775213573365219,
27.1415704883507));
#40519=CARTESIAN_POINT('Ctrl Pts',(11.5945301448752,-0.87248081178943,27.0013442020323));
#40520=CARTESIAN_POINT('Ctrl Pts',(11.6051393477735,-0.930184920342645,
26.8463852694405));
#40521=CARTESIAN_POINT('Ctrl Pts',(11.6127039726369,-0.971329381285666,
26.7358957062249));
#40522=CARTESIAN_POINT('Ctrl Pts',(11.6202685975004,-0.992359773820853,
26.617916001154));
#40523=CARTESIAN_POINT('Ctrl Pts',(11.6278332223638,-0.992471224471742,
26.4999749790724));
#40524=CARTESIAN_POINT('Origin',(18.,0.,26.5));
#40525=CARTESIAN_POINT('',(12.1721667776362,-0.992619537425882,26.499861786204));
#40526=CARTESIAN_POINT('',(12.0278332223638,-0.992474254593845,26.5000252858765));
#40527=CARTESIAN_POINT('',(18.,-0.9925,26.5));
#40528=CARTESIAN_POINT('Ctrl Pts',(12.1721667776362,-0.992619537425882,
26.499861786204));
#40529=CARTESIAN_POINT('Ctrl Pts',(12.1624142267167,-0.992445382879524,
26.6520503547924));
#40530=CARTESIAN_POINT('Ctrl Pts',(12.1526616757972,-0.956798863523656,
26.8045819639399));
#40531=CARTESIAN_POINT('Ctrl Pts',(12.1429091248777,-0.889466903262642,
26.9405929119523));
#40532=CARTESIAN_POINT('Ctrl Pts',(12.1323235893772,-0.81638398766988,27.0882208228991));
#40533=CARTESIAN_POINT('Ctrl Pts',(12.1217380538767,-0.705971847579991,
27.2163854267011));
#40534=CARTESIAN_POINT('Ctrl Pts',(12.1111525183761,-0.570822728387213,
27.3115718104357));
#40535=CARTESIAN_POINT('Ctrl Pts',(12.1005669828756,-0.435673609194435,
27.4067581941702));
#40536=CARTESIAN_POINT('Ctrl Pts',(12.0899814473751,-0.275787510898768,
27.4689663578372));
#40537=CARTESIAN_POINT('Ctrl Pts',(12.0793959118745,-0.11202748104491,27.4872537945506));
#40538=CARTESIAN_POINT('Ctrl Pts',(12.0582248408735,0.21549257866281,27.5238286679774));
#40539=CARTESIAN_POINT('Ctrl Pts',(12.0370537698724,0.558508364603297,27.3847206335896));
#40540=CARTESIAN_POINT('Ctrl Pts',(12.0158826988714,0.768036748408632,27.1303489227862));
#40541=CARTESIAN_POINT('Ctrl Pts',(12.0052971633708,0.872800940311296,27.0031630673845));
#40542=CARTESIAN_POINT('Ctrl Pts',(11.9947116278703,0.944193281680175,26.8471612928789));
#40543=CARTESIAN_POINT('Ctrl Pts',(11.9841260923698,0.974865815542366,26.6847269131019));
#40544=CARTESIAN_POINT('Ctrl Pts',(11.9735405568692,1.00553834940456,26.522292533325));
#40545=CARTESIAN_POINT('Ctrl Pts',(11.9629550213687,0.99549107576006,26.3534255482768));
#40546=CARTESIAN_POINT('Ctrl Pts',(11.9523694858682,0.945102312316298,26.1965941574118));
#40547=CARTESIAN_POINT('Ctrl Pts',(11.9417839503676,0.894713548872537,26.0397627665468));
#40548=CARTESIAN_POINT('Ctrl Pts',(11.9311984148671,0.803983295629513,25.894966969865));
#40549=CARTESIAN_POINT('Ctrl Pts',(11.9206128793666,0.684457208950646,25.7810527130143));
#40550=CARTESIAN_POINT('Ctrl Pts',(11.910027343866,0.564931122271776,25.6671384561637));
#40551=CARTESIAN_POINT('Ctrl Pts',(11.8994418083655,0.416609202157062,25.5841057391443));
#40552=CARTESIAN_POINT('Ctrl Pts',(11.888856272865,0.257283901945971,25.541416786935));
#40553=CARTESIAN_POINT('Ctrl Pts',(11.8782707373644,0.0979586017348822,
25.4987278347256));
#40554=CARTESIAN_POINT('Ctrl Pts',(11.8676852018639,-0.0723700785725825,
25.4963826473263));
#40555=CARTESIAN_POINT('Ctrl Pts',(11.8570996663634,-0.232761627146138,
25.5350337730709));
#40556=CARTESIAN_POINT('Ctrl Pts',(11.8465141308628,-0.393153175719694,
25.5736848988155));
#40557=CARTESIAN_POINT('Ctrl Pts',(11.8359285953623,-0.543607592559341,
25.653332337704));
#40558=CARTESIAN_POINT('Ctrl Pts',(11.8253430598618,-0.6659545777768,25.7640417972626));
#40559=CARTESIAN_POINT('Ctrl Pts',(11.8147575243612,-0.788301562994261,
25.8747512568212));
#40560=CARTESIAN_POINT('Ctrl Pts',(11.8041719888607,-0.882541116589533,
26.0165227370498));
#40561=CARTESIAN_POINT('Ctrl Pts',(11.7935864533602,-0.93697823267869,26.1722659833465));
#40562=CARTESIAN_POINT('Ctrl Pts',(11.7864465614522,-0.973695801160667,
26.2773140410383));
#40563=CARTESIAN_POINT('Ctrl Pts',(11.7793066695442,-0.992305503429818,
26.3887184649872));
#40564=CARTESIAN_POINT('Ctrl Pts',(11.7721667776362,-0.992366447419476,
26.5000655238227));
#40565=CARTESIAN_POINT('Ctrl Pts',(11.6278332223638,-0.992471224471742,
26.4999749790724));
#40566=CARTESIAN_POINT('Ctrl Pts',(11.6308778003986,-0.992516080655597,
26.4525065782307));
#40567=CARTESIAN_POINT('Ctrl Pts',(11.6339223784335,-0.989172345930418,
26.4050444435199));
#40568=CARTESIAN_POINT('Ctrl Pts',(11.6369669564683,-0.982387545983623,
26.3580794221597));
#40569=CARTESIAN_POINT('Ctrl Pts',(11.6475761593666,-0.958745084389168,
26.1944240863357));
#40570=CARTESIAN_POINT('Ctrl Pts',(11.6581853622648,-0.893319182518039,
26.036804993553));
#40571=CARTESIAN_POINT('Ctrl Pts',(11.6687945651631,-0.794117446424462,
25.9045134575807));
#40572=CARTESIAN_POINT('Ctrl Pts',(11.6794037680614,-0.694915710330884,
25.7722219216083));
#40573=CARTESIAN_POINT('Ctrl Pts',(11.6900129709597,-0.561938140014856,
25.6652579424464));
#40574=CARTESIAN_POINT('Ctrl Pts',(11.7006221738579,-0.411460124377188,
25.596713053916));
#40575=CARTESIAN_POINT('Ctrl Pts',(11.7112313767562,-0.260982108739517,
25.5281681653856));
#40576=CARTESIAN_POINT('Ctrl Pts',(11.7218405796545,-0.093003647780212,
25.4980423674867));
#40577=CARTESIAN_POINT('Ctrl Pts',(11.7324497825527,0.0719160410885499,
25.5100228164486));
#40578=CARTESIAN_POINT('Ctrl Pts',(11.743058985451,0.236835729957307,25.5220032654105));
#40579=CARTESIAN_POINT('Ctrl Pts',(11.7536681883493,0.398696646735515,25.5760899612332));
#40580=CARTESIAN_POINT('Ctrl Pts',(11.7642773912476,0.537688312391664,25.6656631258085));
#40581=CARTESIAN_POINT('Ctrl Pts',(11.7748865941458,0.676679978047811,25.7552362903837));
#40582=CARTESIAN_POINT('Ctrl Pts',(11.7854957970441,0.792802392581904,25.8802959237115));
#40583=CARTESIAN_POINT('Ctrl Pts',(11.7961049999424,0.871843103080623,26.0255357289226));
#40584=CARTESIAN_POINT('Ctrl Pts',(11.8067142028407,0.950883813579343,26.1707755341337));
#40585=CARTESIAN_POINT('Ctrl Pts',(11.8173234057389,0.992842820042693,26.3361955112281));
#40586=CARTESIAN_POINT('Ctrl Pts',(11.8279326086372,0.99258467634649,26.5015495807145));
#40587=CARTESIAN_POINT('Ctrl Pts',(11.8385418115355,0.992326532650287,26.666903650201));
#40588=CARTESIAN_POINT('Ctrl Pts',(11.8491510144337,0.949851238794532,26.8321918120795));
#40589=CARTESIAN_POINT('Ctrl Pts',(11.859760217332,0.870357430342617,26.9771841199848));
#40590=CARTESIAN_POINT('Ctrl Pts',(11.8703694202303,0.790863621890701,27.1221764278901));
#40591=CARTESIAN_POINT('Ctrl Pts',(11.8809786231286,0.674351298842628,27.2468728818222));
#40592=CARTESIAN_POINT('Ctrl Pts',(11.8915878260268,0.535080635789019,27.3360116351594));
#40593=CARTESIAN_POINT('Ctrl Pts',(11.9021970289251,0.395809972735412,27.4251503884966));
#40594=CARTESIAN_POINT('Ctrl Pts',(11.9128062318234,0.233780969676272,27.4787314412388));
#40595=CARTESIAN_POINT('Ctrl Pts',(11.9234154347217,0.0688246780568229,
27.4901969019385));
#40596=CARTESIAN_POINT('Ctrl Pts',(11.9340246376199,-0.0961316135626239,
27.5016623626382));
#40597=CARTESIAN_POINT('Ctrl Pts',(11.9446338405182,-0.264015193742381,
27.4710122312954));
#40598=CARTESIAN_POINT('Ctrl Pts',(11.9552430434165,-0.414278457717283,
27.4019978383509));
#40599=CARTESIAN_POINT('Ctrl Pts',(11.9658522463147,-0.564541721692185,
27.3329834454063));
#40600=CARTESIAN_POINT('Ctrl Pts',(11.976461449213,-0.697184669462232,27.22560479086));
#40601=CARTESIAN_POINT('Ctrl Pts',(11.9870706521113,-0.795972867244521,
27.0930041614768));
#40602=CARTESIAN_POINT('Ctrl Pts',(11.9976798550096,-0.894761065026811,
26.9604035320936));
#40603=CARTESIAN_POINT('Ctrl Pts',(12.0082890579078,-0.959694512821341,
26.8025809278734));
#40604=CARTESIAN_POINT('Ctrl Pts',(12.0188982608061,-0.982825877006247,
26.6388525707546));
#40605=CARTESIAN_POINT('Ctrl Pts',(12.0218765813253,-0.989319542670898,
26.5928891246537));
#40606=CARTESIAN_POINT('Ctrl Pts',(12.0248549018446,-0.992518816247691,
26.5464602504224));
#40607=CARTESIAN_POINT('Ctrl Pts',(12.0278332223638,-0.992474254593845,
26.5000252858765));
#40608=CARTESIAN_POINT('Origin',(18.,0.,26.5));
#40609=CARTESIAN_POINT('',(12.5721667776362,-0.992298354748071,26.4996276611265));
#40610=CARTESIAN_POINT('',(12.4278332223638,-0.992540878678463,26.4999779426563));
#40611=CARTESIAN_POINT('',(18.,-0.9925,26.5));
#40612=CARTESIAN_POINT('Ctrl Pts',(12.5721667776362,-0.992298354748071,
26.4996276611265));
#40613=CARTESIAN_POINT('Ctrl Pts',(12.5666928548903,-0.992202803623357,
26.5847133847472));
#40614=CARTESIAN_POINT('Ctrl Pts',(12.5612189321444,-0.981239055656051,
26.6698717450131));
#40615=CARTESIAN_POINT('Ctrl Pts',(12.5557450093985,-0.959533788525683,
26.7525515777318));
#40616=CARTESIAN_POINT('Ctrl Pts',(12.545159473898,-0.91755989038677,26.9124388003046));
#40617=CARTESIAN_POINT('Ctrl Pts',(12.5345739383974,-0.835416712401015,
27.0630572532426));
#40618=CARTESIAN_POINT('Ctrl Pts',(12.5239884028969,-0.722001864471279,
27.1825932310416));
#40619=CARTESIAN_POINT('Ctrl Pts',(12.5028173318958,-0.495172168611806,
27.4216651866396));
#40620=CARTESIAN_POINT('Ctrl Pts',(12.4816462608948,-0.143255792976409,
27.5364072416815));
#40621=CARTESIAN_POINT('Ctrl Pts',(12.4604751898937,0.180898312867456,27.4769831174414));
#40622=CARTESIAN_POINT('Ctrl Pts',(12.4498896543932,0.342975365789387,27.4472710553214));
#40623=CARTESIAN_POINT('Ctrl Pts',(12.4393041188926,0.498111851263434,27.3740174483809));
#40624=CARTESIAN_POINT('Ctrl Pts',(12.4287185833921,0.626262354207043,27.2695991517929));
#40625=CARTESIAN_POINT('Ctrl Pts',(12.4181330478916,0.754412857150651,27.1651808552049));
#40626=CARTESIAN_POINT('Ctrl Pts',(12.407547512391,0.855577377563819,27.0295978689694));
#40627=CARTESIAN_POINT('Ctrl Pts',(12.3969619768905,0.918141159608453,26.8772138612182));
#40628=CARTESIAN_POINT('Ctrl Pts',(12.38637644139,0.980704941653088,26.724829853467));
#40629=CARTESIAN_POINT('Ctrl Pts',(12.3757909058894,1.00466798532919,26.5556448242001));
#40630=CARTESIAN_POINT('Ctrl Pts',(12.3652053703889,0.986710013514384,26.3915093479651));
#40631=CARTESIAN_POINT('Ctrl Pts',(12.3546198348884,0.96875204169958,26.2273738717301));
#40632=CARTESIAN_POINT('Ctrl Pts',(12.3440342993879,0.908873054393874,26.0682879485269));
#40633=CARTESIAN_POINT('Ctrl Pts',(12.3334487638873,0.814577187513826,25.932954333274));
#40634=CARTESIAN_POINT('Ctrl Pts',(12.3228632283868,0.720281320633778,25.7976207180211));
#40635=CARTESIAN_POINT('Ctrl Pts',(12.3122776928863,0.591568574179388,25.6860394107184));
#40636=CARTESIAN_POINT('Ctrl Pts',(12.3016921573857,0.444028354131184,25.6122068850723));
#40637=CARTESIAN_POINT('Ctrl Pts',(12.2911066218852,0.296488134082977,25.5383743594262));
#40638=CARTESIAN_POINT('Ctrl Pts',(12.2805210863847,0.130120440440954,25.5022906154369));
#40639=CARTESIAN_POINT('Ctrl Pts',(12.2699355508841,-0.0347793480614057,
25.5080723953903));
#40640=CARTESIAN_POINT('Ctrl Pts',(12.2593500153836,-0.199679136563763,
25.5138541753437));
#40641=CARTESIAN_POINT('Ctrl Pts',(12.2487644798831,-0.363111019926459,
25.5615014792399));
#40642=CARTESIAN_POINT('Ctrl Pts',(12.2381789443825,-0.505117790383664,
25.6454862130876));
#40643=CARTESIAN_POINT('Ctrl Pts',(12.227593408882,-0.647124560840869,25.7294709469352));
#40644=CARTESIAN_POINT('Ctrl Pts',(12.2170078733815,-0.767706218392585,
25.8497931107343));
#40645=CARTESIAN_POINT('Ctrl Pts',(12.2064223378809,-0.852291934685505,
25.9913987410154));
#40646=CARTESIAN_POINT('Ctrl Pts',(12.1958368023804,-0.936877650978427,
26.1330043712965));
#40647=CARTESIAN_POINT('Ctrl Pts',(12.1852512668799,-0.985467426012552,
26.2958934680595));
#40648=CARTESIAN_POINT('Ctrl Pts',(12.1746657313793,-0.991885467981796,
26.4608836254868));
#40649=CARTESIAN_POINT('Ctrl Pts',(12.1738327467983,-0.992390509035276,
26.473866838018));
#40650=CARTESIAN_POINT('Ctrl Pts',(12.1729997622173,-0.992634412308672,
26.4868630608355));
#40651=CARTESIAN_POINT('Ctrl Pts',(12.1721667776362,-0.992619537425882,
26.499861786204));
#40652=CARTESIAN_POINT('Ctrl Pts',(12.0278332223638,-0.992474254593845,
26.5000252858765));
#40653=CARTESIAN_POINT('Ctrl Pts',(12.0354641047429,-0.992360081274713,
26.3810522772844));
#40654=CARTESIAN_POINT('Ctrl Pts',(12.0430949871219,-0.970951506468747,
26.2620392883616));
#40655=CARTESIAN_POINT('Ctrl Pts',(12.0507258695009,-0.929098865159217,
26.15071209629));
#40656=CARTESIAN_POINT('Ctrl Pts',(12.0613350723992,-0.870911208551999,
25.9959340889619));
#40657=CARTESIAN_POINT('Ctrl Pts',(12.0719442752975,-0.773206614762282,
25.8560121843233));
#40658=CARTESIAN_POINT('Ctrl Pts',(12.0825534781957,-0.647943343047954,
25.748071702143));
#40659=CARTESIAN_POINT('Ctrl Pts',(12.093162681094,-0.522680071333622,25.6401312199627));
#40660=CARTESIAN_POINT('Ctrl Pts',(12.1037718839923,-0.369858121694682,
25.5641721602407));
#40661=CARTESIAN_POINT('Ctrl Pts',(12.1143810868906,-0.208181676024677,
25.5294913031375));
#40662=CARTESIAN_POINT('Ctrl Pts',(12.1249902897888,-0.0465052303546761,
25.4948104460343));
#40663=CARTESIAN_POINT('Ctrl Pts',(12.1355994926871,0.124025711346386,25.5014077915499));
#40664=CARTESIAN_POINT('Ctrl Pts',(12.1462086955854,0.28253952847956,25.5484758774656));
#40665=CARTESIAN_POINT('Ctrl Pts',(12.1568178984836,0.441053345612737,25.5955439633813));
#40666=CARTESIAN_POINT('Ctrl Pts',(12.1674271013819,0.587550038178023,25.6830827896971));
#40667=CARTESIAN_POINT('Ctrl Pts',(12.1780363042802,0.704099585055956,25.8003783056235));
#40668=CARTESIAN_POINT('Ctrl Pts',(12.1886455071785,0.820649131933889,25.9176738215499));
#40669=CARTESIAN_POINT('Ctrl Pts',(12.1992547100767,0.907251533124466,26.064726027087));
#40670=CARTESIAN_POINT('Ctrl Pts',(12.209863912975,0.953307348768988,26.2235369107796));
#40671=CARTESIAN_POINT('Ctrl Pts',(12.2204731158733,0.999363164413512,26.3823477944721));
#40672=CARTESIAN_POINT('Ctrl Pts',(12.2310823187716,1.00487239451198,26.5529173563202));
#40673=CARTESIAN_POINT('Ctrl Pts',(12.2416915216698,0.969160753452287,26.7143692489282));
#40674=CARTESIAN_POINT('Ctrl Pts',(12.2523007245681,0.933449112392596,26.8758211415363));
#40675=CARTESIAN_POINT('Ctrl Pts',(12.2629099274664,0.856516600174747,27.0281553649044));
#40676=CARTESIAN_POINT('Ctrl Pts',(12.2735191303646,0.747779139743386,27.1527274309257));
#40677=CARTESIAN_POINT('Ctrl Pts',(12.2841283332629,0.639041679312023,27.2772994969471));
#40678=CARTESIAN_POINT('Ctrl Pts',(12.2947375361612,0.498499270667149,27.3741094056218));
#40679=CARTESIAN_POINT('Ctrl Pts',(12.3053467390595,0.343353178295059,27.4313083999798));
#40680=CARTESIAN_POINT('Ctrl Pts',(12.3159559419577,0.188207085922968,27.4885073943378));
#40681=CARTESIAN_POINT('Ctrl Pts',(12.326565144856,0.0184573098236633,27.5060954743792));
#40682=CARTESIAN_POINT('Ctrl Pts',(12.3371743477543,-0.145120137813161,
27.4819200000608));
#40683=CARTESIAN_POINT('Ctrl Pts',(12.3477835506525,-0.308697585449984,
27.4577445257424));
#40684=CARTESIAN_POINT('Ctrl Pts',(12.3583927535508,-0.46610270462433,27.3918054970643));
#40685=CARTESIAN_POINT('Ctrl Pts',(12.3690019564491,-0.598070370221847,
27.2921733226895));
#40686=CARTESIAN_POINT('Ctrl Pts',(12.3796111593474,-0.730038035819365,
27.1925411483148));
#40687=CARTESIAN_POINT('Ctrl Pts',(12.3902203622456,-0.836568247840052,
27.0592158282434));
#40688=CARTESIAN_POINT('Ctrl Pts',(12.4008295651439,-0.904622562084627,
26.9085153131594));
#40689=CARTESIAN_POINT('Ctrl Pts',(12.4098307842172,-0.962362224269649,
26.7806557214693));
#40690=CARTESIAN_POINT('Ctrl Pts',(12.4188320032905,-0.992405321125612,
26.6402887354989));
#40691=CARTESIAN_POINT('Ctrl Pts',(12.4278332223638,-0.992540878678463,
26.4999779426563));
#40692=CARTESIAN_POINT('Origin',(18.,0.,26.5));
#40693=CARTESIAN_POINT('',(12.9721667776362,-0.993584665131883,26.5006674583246));
#40694=CARTESIAN_POINT('',(12.8278332223638,-0.992423719932019,26.5000125385131));
#40695=CARTESIAN_POINT('',(18.,-0.9925,26.5));
#40696=CARTESIAN_POINT('Ctrl Pts',(12.9721667776362,-0.993584665131883,
26.5006674583246));
#40697=CARTESIAN_POINT('Ctrl Pts',(12.9709714830639,-0.993603791415993,
26.519301517892));
#40698=CARTESIAN_POINT('Ctrl Pts',(12.9697761884916,-0.993073070228261,
26.537921851123));
#40699=CARTESIAN_POINT('Ctrl Pts',(12.9685808939192,-0.991982052232969,
26.5564961893539));
#40700=CARTESIAN_POINT('Ctrl Pts',(12.9474098229182,-0.972657929145171,
26.8854850784429));
#40701=CARTESIAN_POINT('Ctrl Pts',(12.9262387519171,-0.777560099683024,
27.2000446301572));
#40702=CARTESIAN_POINT('Ctrl Pts',(12.9050676809161,-0.491426019562643,
27.3635512021071));
#40703=CARTESIAN_POINT('Ctrl Pts',(12.8944821454155,-0.348358979502456,
27.445304488082));
#40704=CARTESIAN_POINT('Ctrl Pts',(12.883896609915,-0.182532876777712,27.4892945291159));
#40705=CARTESIAN_POINT('Ctrl Pts',(12.8733110744145,-0.0172511009544274,
27.4920634003193));
#40706=CARTESIAN_POINT('Ctrl Pts',(12.8627255389139,0.148030674868862,27.4948322715228));
#40707=CARTESIAN_POINT('Ctrl Pts',(12.8521400034134,0.312768123790687,27.4563799728959));
#40708=CARTESIAN_POINT('Ctrl Pts',(12.8415544679129,0.458822861540175,27.3802017199428));
#40709=CARTESIAN_POINT('Ctrl Pts',(12.8309689324123,0.604877599289659,27.3040234669898));
#40710=CARTESIAN_POINT('Ctrl Pts',(12.8203833969118,0.732249625866807,27.1901192597107));
#40711=CARTESIAN_POINT('Ctrl Pts',(12.8097978614113,0.824316265337188,27.0530547595393));
#40712=CARTESIAN_POINT('Ctrl Pts',(12.7992123259107,0.916382904807572,26.9159902593679));
#40713=CARTESIAN_POINT('Ctrl Pts',(12.7886267904102,0.973144157171193,26.7557654663044));
#40714=CARTESIAN_POINT('Ctrl Pts',(12.7780412549097,0.988282106757489,26.5915164467931));
#40715=CARTESIAN_POINT('Ctrl Pts',(12.7674557194091,1.00342005634378,26.4272674272819));
#40716=CARTESIAN_POINT('Ctrl Pts',(12.7568701839086,0.976934703152756,26.2589941813229));
#40717=CARTESIAN_POINT('Ctrl Pts',(12.7462846484081,0.91172322008537,26.1074461003344));
#40718=CARTESIAN_POINT('Ctrl Pts',(12.7356991129075,0.846511737017982,25.9558980193459));
#40719=CARTESIAN_POINT('Ctrl Pts',(12.725113577407,0.742574124074235,25.8210751033278));
#40720=CARTESIAN_POINT('Ctrl Pts',(12.7145280419065,0.612773646105535,25.7192065353265));
#40721=CARTESIAN_POINT('Ctrl Pts',(12.7039425064059,0.482973168136835,25.6173379673251));
#40722=CARTESIAN_POINT('Ctrl Pts',(12.6933569709054,0.327309825143181,25.5484237473404));
#40723=CARTESIAN_POINT('Ctrl Pts',(12.6827714354049,0.164605080401317,25.5211011483858));
#40724=CARTESIAN_POINT('Ctrl Pts',(12.6721858999044,0.00190033565945694,
25.4937785494312));
#40725=CARTESIAN_POINT('Ctrl Pts',(12.6616003644038,-0.167845810830615,
25.5080475715067));
#40726=CARTESIAN_POINT('Ctrl Pts',(12.6510148289033,-0.323789974945903,
25.5617906232108));
#40727=CARTESIAN_POINT('Ctrl Pts',(12.6404292934027,-0.479734139061194,
25.6155336749149));
#40728=CARTESIAN_POINT('Ctrl Pts',(12.6298437579022,-0.621876320801701,
25.7087507562476));
#40729=CARTESIAN_POINT('Ctrl Pts',(12.6192582224017,-0.73313048178971,25.8307567191078));
#40730=CARTESIAN_POINT('Ctrl Pts',(12.6086726869012,-0.844384642777722,
25.9527626819681));
#40731=CARTESIAN_POINT('Ctrl Pts',(12.5980871514006,-0.924750783013234,
26.1035575263558));
#40732=CARTESIAN_POINT('Ctrl Pts',(12.5875016159001,-0.964031543984952,
26.2635329446535));
#40733=CARTESIAN_POINT('Ctrl Pts',(12.5823900031455,-0.982999695268774,
26.3407829230373));
#40734=CARTESIAN_POINT('Ctrl Pts',(12.5772783903908,-0.992387581500161,
26.4201736223531));
#40735=CARTESIAN_POINT('Ctrl Pts',(12.5721667776362,-0.992298354748071,
26.4996276611265));
#40736=CARTESIAN_POINT('Ctrl Pts',(12.4278332223638,-0.992540878678463,
26.4999779426563));
#40737=CARTESIAN_POINT('Ctrl Pts',(12.4294412061888,-0.992565094770813,
26.47491272832));
#40738=CARTESIAN_POINT('Ctrl Pts',(12.4310491900138,-0.991634886822353,
26.4498493072463));
#40739=CARTESIAN_POINT('Ctrl Pts',(12.4326571738387,-0.98973765036095,26.4248593027964));
#40740=CARTESIAN_POINT('Ctrl Pts',(12.443266376737,-0.977220007924238,26.2599795176142));
#40741=CARTESIAN_POINT('Ctrl Pts',(12.4538755796353,-0.922606306582356,
26.0982956573466));
#40742=CARTESIAN_POINT('Ctrl Pts',(12.4644847825335,-0.832580825695646,
25.9595965307271));
#40743=CARTESIAN_POINT('Ctrl Pts',(12.4750939854318,-0.742555344808936,
25.8208974041076));
#40744=CARTESIAN_POINT('Ctrl Pts',(12.4857031883301,-0.617118084377399,
25.7051830111362));
#40745=CARTESIAN_POINT('Ctrl Pts',(12.4963123912284,-0.47162155980136,25.6266158661569));
#40746=CARTESIAN_POINT('Ctrl Pts',(12.5069215941266,-0.326125035225322,
25.5480487211777));
#40747=CARTESIAN_POINT('Ctrl Pts',(12.5175307970249,-0.160569246504779,
25.5066288241905));
#40748=CARTESIAN_POINT('Ctrl Pts',(12.5281399999232,0.00478310461436772,
25.5074256386403));
#40749=CARTESIAN_POINT('Ctrl Pts',(12.5387492028215,0.170135455733517,25.5082224530901));
#40750=CARTESIAN_POINT('Ctrl Pts',(12.5493584057197,0.335284369251272,25.5512359789769));
#40751=CARTESIAN_POINT('Ctrl Pts',(12.559967608618,0.480016941685798,25.6312017054501));
#40752=CARTESIAN_POINT('Ctrl Pts',(12.5705768115163,0.624749514120321,25.7111674319232));
#40753=CARTESIAN_POINT('Ctrl Pts',(12.5811860144145,0.749065745471615,25.8280853589828));
#40754=CARTESIAN_POINT('Ctrl Pts',(12.5917952173128,0.837750325314641,25.9676456693578));
#40755=CARTESIAN_POINT('Ctrl Pts',(12.6024044202111,0.92643490515767,26.1072059797328));
#40756=CARTESIAN_POINT('Ctrl Pts',(12.6130136231094,0.979487833492432,26.2694086734232));
#40757=CARTESIAN_POINT('Ctrl Pts',(12.6236228260076,0.990415857066348,26.4344014406425));
#40758=CARTESIAN_POINT('Ctrl Pts',(12.6342320289059,1.00134388064026,26.5993942078617));
#40759=CARTESIAN_POINT('Ctrl Pts',(12.6448412318042,0.970146999453333,26.7671770486098));
#40760=CARTESIAN_POINT('Ctrl Pts',(12.6554504347025,0.900643461745485,26.9172146878207));
#40761=CARTESIAN_POINT('Ctrl Pts',(12.6660596376007,0.831139924037638,27.0672523270317));
#40762=CARTESIAN_POINT('Ctrl Pts',(12.676668840499,0.723329729808879,27.1995447647054));
#40763=CARTESIAN_POINT('Ctrl Pts',(12.6872780433973,0.590407982822753,27.2979004666858));
#40764=CARTESIAN_POINT('Ctrl Pts',(12.6978872462955,0.457486235836628,27.3962561686662));
#40765=CARTESIAN_POINT('Ctrl Pts',(12.7084964491938,0.299452936093136,27.4606751349532));
#40766=CARTESIAN_POINT('Ctrl Pts',(12.7191056520921,0.135650092973945,27.4832730003384));
#40767=CARTESIAN_POINT('Ctrl Pts',(12.7297148549904,-0.0281527501452476,
27.5058708657235));
#40768=CARTESIAN_POINT('Ctrl Pts',(12.7403240578886,-0.19772513664014,27.4866476302068));
#40769=CARTESIAN_POINT('Ctrl Pts',(12.7509332607869,-0.352312765386994,
27.4279560637571));
#40770=CARTESIAN_POINT('Ctrl Pts',(12.7615424636852,-0.506900394133848,
27.3692644973074));
#40771=CARTESIAN_POINT('Ctrl Pts',(12.7721516665834,-0.646503265132669,
27.2711045999246));
#40772=CARTESIAN_POINT('Ctrl Pts',(12.7827608694817,-0.754035105775395,
27.1454903563777));
#40773=CARTESIAN_POINT('Ctrl Pts',(12.79337007238,-0.861566946418121,27.0198761128307));
#40774=CARTESIAN_POINT('Ctrl Pts',(12.8039792752783,-0.937027756704759,
26.8668075231194));
#40775=CARTESIAN_POINT('Ctrl Pts',(12.8145884781765,-0.971181738212568,
26.7050189559057));
#40776=CARTESIAN_POINT('Ctrl Pts',(12.8190033929056,-0.985394579409199,
26.6376922457618));
#40777=CARTESIAN_POINT('Ctrl Pts',(12.8234183076347,-0.992454210461741,
26.5688554746092));
#40778=CARTESIAN_POINT('Ctrl Pts',(12.8278332223638,-0.992423719932019,
26.5000125385131));
#40779=CARTESIAN_POINT('Origin',(18.,0.,26.5));
#40780=CARTESIAN_POINT('',(13.3721667776362,-0.990996827870586,26.5001850440327));
#40781=CARTESIAN_POINT('',(13.2278332223638,-0.992585204636762,26.4999971408611));
#40782=CARTESIAN_POINT('',(18.,-0.9925,26.5));
#40783=CARTESIAN_POINT('Ctrl Pts',(13.3721667776362,-0.990996827870586,
26.5001850440327));
#40784=CARTESIAN_POINT('Ctrl Pts',(13.3646645757369,-0.991718635376042,
26.6170275101808));
#40785=CARTESIAN_POINT('Ctrl Pts',(13.3571623738377,-0.972510103653976,
26.7338149156839));
#40786=CARTESIAN_POINT('Ctrl Pts',(13.3496601719384,-0.932335445090473,
26.843468818369));
#40787=CARTESIAN_POINT('Ctrl Pts',(13.3390746364379,-0.875649384097233,
26.9981894317609));
#40788=CARTESIAN_POINT('Ctrl Pts',(13.3284891009373,-0.777221983820787,
27.1387079961211));
#40789=CARTESIAN_POINT('Ctrl Pts',(13.3179035654368,-0.652640928626889,
27.247360160176));
#40790=CARTESIAN_POINT('Ctrl Pts',(13.3073180299363,-0.528059873432998,
27.3560123242309));
#40791=CARTESIAN_POINT('Ctrl Pts',(13.2967324944357,-0.377325163321658,
27.4327980879805));
#40792=CARTESIAN_POINT('Ctrl Pts',(13.2861469589352,-0.216557357470861,
27.4686983002914));
#40793=CARTESIAN_POINT('Ctrl Pts',(13.2755614234347,-0.0557895516200603,
27.5045985126023));
#40794=CARTESIAN_POINT('Ctrl Pts',(13.2649758879341,0.115011349970196,27.4996131734745));
#40795=CARTESIAN_POINT('Ctrl Pts',(13.2543903524336,0.273747971638755,27.4541639902932));
#40796=CARTESIAN_POINT('Ctrl Pts',(13.2438048169331,0.432484593307314,27.4087148071119));
#40797=CARTESIAN_POINT('Ctrl Pts',(13.2332192814326,0.579156935054173,27.3228017798771));
#40798=CARTESIAN_POINT('Ctrl Pts',(13.222633745932,0.696600166892606,27.2069830196376));
#40799=CARTESIAN_POINT('Ctrl Pts',(13.2120482104315,0.814043398731035,27.091164259398));
#40800=CARTESIAN_POINT('Ctrl Pts',(13.201462674931,0.902257520661038,26.9454397661536));
#40801=CARTESIAN_POINT('Ctrl Pts',(13.1908771394304,0.95008317966956,26.7875408595217));
#40802=CARTESIAN_POINT('Ctrl Pts',(13.1802916039299,0.997908838678084,26.6296419528898));
#40803=CARTESIAN_POINT('Ctrl Pts',(13.1697060684293,1.00534603476512,26.4595686328704));
#40804=CARTESIAN_POINT('Ctrl Pts',(13.1591205329288,0.971768544810025,26.2980201219027));
#40805=CARTESIAN_POINT('Ctrl Pts',(13.1485349974283,0.938191054854925,26.1364716109351));
#40806=CARTESIAN_POINT('Ctrl Pts',(13.1379494619278,0.863598878857685,25.9834479090192));
#40807=CARTESIAN_POINT('Ctrl Pts',(13.1273639264272,0.756814616848371,25.8576843222292));
#40808=CARTESIAN_POINT('Ctrl Pts',(13.1167783909267,0.65003035483906,25.7319207354392));
#40809=CARTESIAN_POINT('Ctrl Pts',(13.1061928554262,0.511054006817676,25.6334172637753));
#40810=CARTESIAN_POINT('Ctrl Pts',(13.0956073199256,0.357186261541762,25.5739898720119));
#40811=CARTESIAN_POINT('Ctrl Pts',(13.0850217844251,0.203318516265847,25.5145624802486));
#40812=CARTESIAN_POINT('Ctrl Pts',(13.0744362489246,0.034559373735403,25.4942111683859));
#40813=CARTESIAN_POINT('Ctrl Pts',(13.063850713424,-0.129140779817654,25.5157797343396));
#40814=CARTESIAN_POINT('Ctrl Pts',(13.0532651779235,-0.292840933370716,
25.5373483002933));
#40815=CARTESIAN_POINT('Ctrl Pts',(13.042679642423,-0.451482097946389,25.6008367440633));
#40816=CARTESIAN_POINT('Ctrl Pts',(13.0320941069224,-0.584629033760132,
25.6978264658149));
#40817=CARTESIAN_POINT('Ctrl Pts',(13.0215085714219,-0.717775969573874,
25.7948161875666));
#40818=CARTESIAN_POINT('Ctrl Pts',(13.0109230359214,-0.825428676625686,
25.9253071872998));
#40819=CARTESIAN_POINT('Ctrl Pts',(13.0003375004208,-0.896395712676435,
26.0746035766105));
#40820=CARTESIAN_POINT('Ctrl Pts',(12.9909472594926,-0.959349312562228,
26.2070417574913));
#40821=CARTESIAN_POINT('Ctrl Pts',(12.9815570185644,-0.993434408935617,
26.3542781808535));
#40822=CARTESIAN_POINT('Ctrl Pts',(12.9721667776362,-0.993584665131883,
26.5006674583246));
#40823=CARTESIAN_POINT('Ctrl Pts',(12.8278332223638,-0.992423719932019,
26.5000125385131));
#40824=CARTESIAN_POINT('Ctrl Pts',(12.834027510533,-0.99238094059445,26.4034233605202));
#40825=CARTESIAN_POINT('Ctrl Pts',(12.8402217987022,-0.97838116847057,26.306822046759));
#40826=CARTESIAN_POINT('Ctrl Pts',(12.8464160868713,-0.950598647581288,
26.2143622011447));
#40827=CARTESIAN_POINT('Ctrl Pts',(12.8570252897696,-0.903014422713221,
26.0560025583136));
#40828=CARTESIAN_POINT('Ctrl Pts',(12.8676344926679,-0.814998820248106,
25.9097918173675));
#40829=CARTESIAN_POINT('Ctrl Pts',(12.8782436955662,-0.697324244555001,
25.7936250012394));
#40830=CARTESIAN_POINT('Ctrl Pts',(12.8888528984644,-0.579649668861895,
25.6774581851113));
#40831=CARTESIAN_POINT('Ctrl Pts',(12.8994621013627,-0.432316119940802,
25.5913352938011));
#40832=CARTESIAN_POINT('Ctrl Pts',(12.910071304261,-0.273356043422418,25.5457970790012));
#40833=CARTESIAN_POINT('Ctrl Pts',(12.9206805071593,-0.114395966904035,
25.5002588642012));
#40834=CARTESIAN_POINT('Ctrl Pts',(12.9312897100575,0.0561906372116295,
25.4953053259114));
#40835=CARTESIAN_POINT('Ctrl Pts',(12.9418989129558,0.217525335692179,25.53154273752));
#40836=CARTESIAN_POINT('Ctrl Pts',(12.9525081158541,0.378860034172724,25.5677801491285));
#40837=CARTESIAN_POINT('Ctrl Pts',(12.9631173187524,0.530942827018157,25.6452085106354));
#40838=CARTESIAN_POINT('Ctrl Pts',(12.9737265216506,0.655159999202703,25.7543512111168));
#40839=CARTESIAN_POINT('Ctrl Pts',(12.9843357245489,0.779377171387251,25.8634939115982));
#40840=CARTESIAN_POINT('Ctrl Pts',(12.9949449274472,0.875728722910919,26.0043509510541));
#40841=CARTESIAN_POINT('Ctrl Pts',(13.0055541303454,0.932421996045665,26.1596825567085));
#40842=CARTESIAN_POINT('Ctrl Pts',(13.0161633332437,0.989115269180413,26.3150141623629));
#40843=CARTESIAN_POINT('Ctrl Pts',(13.026772536142,1.00615026392623,26.4848203342157));
#40844=CARTESIAN_POINT('Ctrl Pts',(13.0373817390403,0.981442033447716,26.648318157689));
#40845=CARTESIAN_POINT('Ctrl Pts',(13.0479909419385,0.956733802969197,26.8118159811624));
#40846=CARTESIAN_POINT('Ctrl Pts',(13.0586001448368,0.890282347266338,26.9690054562562));
#40847=CARTESIAN_POINT('Ctrl Pts',(13.0692093477351,0.790220791963399,27.1006478509634));
#40848=CARTESIAN_POINT('Ctrl Pts',(13.0798185506333,0.69015923666046,27.2322902456707));
#40849=CARTESIAN_POINT('Ctrl Pts',(13.0904277535316,0.556487581757443,27.3383855599913));
#40850=CARTESIAN_POINT('Ctrl Pts',(13.1010369564299,0.405566166546082,27.4059485777192));
#40851=CARTESIAN_POINT('Ctrl Pts',(13.1116461593282,0.254644751334718,27.473511595447));
#40852=CARTESIAN_POINT('Ctrl Pts',(13.1222553622264,0.0864735758150087,
27.5025423165822));
#40853=CARTESIAN_POINT('Ctrl Pts',(13.1328645651247,-0.0783645558831055,
27.4894876135149));
#40854=CARTESIAN_POINT('Ctrl Pts',(13.143473768023,-0.243202687581215,27.4764329104477));
#40855=CARTESIAN_POINT('Ctrl Pts',(13.1540829709213,-0.404707775457734,
27.4212927831782));
#40856=CARTESIAN_POINT('Ctrl Pts',(13.1646921738195,-0.543112891087042,
27.3308159413813));
#40857=CARTESIAN_POINT('Ctrl Pts',(13.1753013767178,-0.681518006716351,
27.2403390995845));
#40858=CARTESIAN_POINT('Ctrl Pts',(13.1859105796161,-0.796823150098447,
27.1145255432603));
#40859=CARTESIAN_POINT('Ctrl Pts',(13.1965197825143,-0.874915895759271,
26.9687738434107));
#40860=CARTESIAN_POINT('Ctrl Pts',(13.2069575957975,-0.951747068260401,
26.8253767340029));
#40861=CARTESIAN_POINT('Ctrl Pts',(13.2173954090807,-0.992558449567449,
26.6626804713408));
#40862=CARTESIAN_POINT('Ctrl Pts',(13.2278332223638,-0.992585204636762,
26.4999971408611));
#40863=CARTESIAN_POINT('Origin',(18.,0.,26.5));
#40864=CARTESIAN_POINT('',(13.7721667776362,-0.992441988512883,26.5000464541839));
#40865=CARTESIAN_POINT('',(13.6278332223638,-0.992417767911371,26.4999920932966));
#40866=CARTESIAN_POINT('',(18.,-0.9925,26.5));
#40867=CARTESIAN_POINT('Ctrl Pts',(13.7721667776362,-0.992441988512883,
26.5000464541839));
#40868=CARTESIAN_POINT('Ctrl Pts',(13.7689432039105,-0.992296790322603,
26.5505240435116));
#40869=CARTESIAN_POINT('Ctrl Pts',(13.7657196301848,-0.988377443742599,
26.6009707314814));
#40870=CARTESIAN_POINT('Ctrl Pts',(13.7624960564592,-0.980698963259128,
26.6507213793718));
#40871=CARTESIAN_POINT('Ctrl Pts',(13.7519105209586,-0.955484454560221,
26.8140920028575));
#40872=CARTESIAN_POINT('Ctrl Pts',(13.7413249854581,-0.889734192649526,
26.969957038724));
#40873=CARTESIAN_POINT('Ctrl Pts',(13.7307394499576,-0.789959661753805,
27.1010301314111));
#40874=CARTESIAN_POINT('Ctrl Pts',(13.720153914457,-0.690185130858087,27.2321032240983));
#40875=CARTESIAN_POINT('Ctrl Pts',(13.7095683789565,-0.556386330977346,
27.3383843736063));
#40876=CARTESIAN_POINT('Ctrl Pts',(13.698982843456,-0.405729575639403,27.4059527492093));
#40877=CARTESIAN_POINT('Ctrl Pts',(13.6883973079554,-0.255072820301461,
27.4735211248124));
#40878=CARTESIAN_POINT('Ctrl Pts',(13.6778117724549,-0.0875581095063172,
27.5023767265106));
#40879=CARTESIAN_POINT('Ctrl Pts',(13.6672262369544,0.0768858145131292,
27.4895278440233));
#40880=CARTESIAN_POINT('Ctrl Pts',(13.6566407014538,0.24132973853258,27.476678961536));
#40881=CARTESIAN_POINT('Ctrl Pts',(13.6460551659533,0.402702875776333,27.4221255948632));
#40882=CARTESIAN_POINT('Ctrl Pts',(13.6354696304528,0.541044341020947,27.3322312270245));
#40883=CARTESIAN_POINT('Ctrl Pts',(13.6248840949522,0.679385806265562,27.2423368591858));
#40884=CARTESIAN_POINT('Ctrl Pts',(13.6142985594517,0.794695599511036,27.1171014901811));
#40885=CARTESIAN_POINT('Ctrl Pts',(13.6037130239512,0.873152901183207,26.9719470171468));
#40886=CARTESIAN_POINT('Ctrl Pts',(13.5931274884506,0.951610202855376,26.8267925441124));
#40887=CARTESIAN_POINT('Ctrl Pts',(13.5825419529501,0.993215012954245,26.6617189670485));
#40888=CARTESIAN_POINT('Ctrl Pts',(13.5719564174496,0.992636462924212,26.4967370781788));
#40889=CARTESIAN_POINT('Ctrl Pts',(13.561370881949,0.992057912894179,26.3317551893091));
#40890=CARTESIAN_POINT('Ctrl Pts',(13.5507853464485,0.949296002735245,26.1668649886337));
#40891=CARTESIAN_POINT('Ctrl Pts',(13.540199810948,0.869961747212413,26.0222518017221));
#40892=CARTESIAN_POINT('Ctrl Pts',(13.5296142754474,0.790627491689576,25.8776386148105));
#40893=CARTESIAN_POINT('Ctrl Pts',(13.5190287399469,0.674720890802834,25.7533024416627));
#40894=CARTESIAN_POINT('Ctrl Pts',(13.5084432044464,0.535661944560877,25.6642768679175));
#40895=CARTESIAN_POINT('Ctrl Pts',(13.4978576689459,0.396602998318923,25.5752512941722));
#40896=CARTESIAN_POINT('Ctrl Pts',(13.4872721334453,0.234391706721755,25.5215363198295));
#40897=CARTESIAN_POINT('Ctrl Pts',(13.4766865979448,0.0700781368495305,
25.5098674125159));
#40898=CARTESIAN_POINT('Ctrl Pts',(13.4661010624443,-0.0942354330226944,
25.4981985052023));
#40899=CARTESIAN_POINT('Ctrl Pts',(13.4555155269437,-0.260651281169975,
25.5285756649179));
#40900=CARTESIAN_POINT('Ctrl Pts',(13.4449299914432,-0.411140528373641,
25.596976823849));
#40901=CARTESIAN_POINT('Ctrl Pts',(13.4343444559427,-0.561629775577303,
25.66537798278));
#40902=CARTESIAN_POINT('Ctrl Pts',(13.4237589204421,-0.69619242183735,25.7718031409266));
#40903=CARTESIAN_POINT('Ctrl Pts',(13.4131733849416,-0.794833058535104,
25.9037948168427));
#40904=CARTESIAN_POINT('Ctrl Pts',(13.3995045158398,-0.922205542531897,
26.0742327640333));
#40905=CARTESIAN_POINT('Ctrl Pts',(13.385835646738,-0.989681708330851,26.287300294095));
#40906=CARTESIAN_POINT('Ctrl Pts',(13.3721667776362,-0.990996827870586,
26.5001850440327));
#40907=CARTESIAN_POINT('Ctrl Pts',(13.2278332223638,-0.992585204636762,
26.4999971408611));
#40908=CARTESIAN_POINT('Ctrl Pts',(13.2280046119789,-0.992585643956848,
26.497325869337));
#40909=CARTESIAN_POINT('Ctrl Pts',(13.228176001594,-0.992575086980314,26.4946546012997));
#40910=CARTESIAN_POINT('Ctrl Pts',(13.2283473912092,-0.992553512612486,
26.4919834222468));
#40911=CARTESIAN_POINT('Ctrl Pts',(13.2389565941074,-0.991218035865332,
26.3266345443076));
#40912=CARTESIAN_POINT('Ctrl Pts',(13.2495657970057,-0.947666734431473,
26.1616266318042));
#40913=CARTESIAN_POINT('Ctrl Pts',(13.260174999904,-0.867229938578543,26.0171553308244));
#40914=CARTESIAN_POINT('Ctrl Pts',(13.2707842028023,-0.786793142725617,
25.8726840298445));
#40915=CARTESIAN_POINT('Ctrl Pts',(13.2813934057005,-0.669470852453621,
25.7487493403882));
#40916=CARTESIAN_POINT('Ctrl Pts',(13.2920026085988,-0.529622375850176,
25.6605198752102));
#40917=CARTESIAN_POINT('Ctrl Pts',(13.3026118114971,-0.389773899246729,
25.5722904100322));
#40918=CARTESIAN_POINT('Ctrl Pts',(13.3132210143953,-0.227399236311832,
25.5197661691326));
#40919=CARTESIAN_POINT('Ctrl Pts',(13.3238302172936,-0.0623717444893147,
25.5093756986589));
#40920=CARTESIAN_POINT('Ctrl Pts',(13.3344394201919,0.102655747333203,25.4989852281851));
#40921=CARTESIAN_POINT('Ctrl Pts',(13.3450486230902,0.270336068043336,25.5307285281372));
#40922=CARTESIAN_POINT('Ctrl Pts',(13.3556578259884,0.420146490206049,25.6007204729975));
#40923=CARTESIAN_POINT('Ctrl Pts',(13.3662670288867,0.56995691236876,25.6707124178578));
#40924=CARTESIAN_POINT('Ctrl Pts',(13.376876231785,0.701897435984052,25.7789530076263));
#40925=CARTESIAN_POINT('Ctrl Pts',(13.3874854346832,0.799819598356204,25.9121944615746));
#40926=CARTESIAN_POINT('Ctrl Pts',(13.3980946375815,0.897741760728361,26.0454359155229));
#40927=CARTESIAN_POINT('Ctrl Pts',(13.4087038404798,0.961645561857379,26.2036782336511));
#40928=CARTESIAN_POINT('Ctrl Pts',(13.4193130433781,0.983709688621481,26.3675538244022));
#40929=CARTESIAN_POINT('Ctrl Pts',(13.4299222462763,1.00577381538558,26.5314294151533));
#40930=CARTESIAN_POINT('Ctrl Pts',(13.4405314491746,0.985998267784771,26.7009382785275));
#40931=CARTESIAN_POINT('Ctrl Pts',(13.4511406520729,0.926803414360631,26.8553338881218));
#40932=CARTESIAN_POINT('Ctrl Pts',(13.4617498549712,0.867608560936492,27.0097294977161));
#40933=CARTESIAN_POINT('Ctrl Pts',(13.4723590578694,0.768994401689023,27.1490118535305));
#40934=CARTESIAN_POINT('Ctrl Pts',(13.4829682607677,0.643030519398727,27.256133911447));
#40935=CARTESIAN_POINT('Ctrl Pts',(13.493577463666,0.517066637108437,27.3632559693634));
#40936=CARTESIAN_POINT('Ctrl Pts',(13.5041866665642,0.363753031775324,27.4382177293818));
#40937=CARTESIAN_POINT('Ctrl Pts',(13.5147958694625,0.201854060009683,27.4718444728329));
#40938=CARTESIAN_POINT('Ctrl Pts',(13.5254050723608,0.0399550882440378,
27.505471216284));
#40939=CARTESIAN_POINT('Ctrl Pts',(13.5360142752591,-0.13052924995413,27.4977629431677));
#40940=CARTESIAN_POINT('Ctrl Pts',(13.5466234781573,-0.288733037881145,
27.4496630843379));
#40941=CARTESIAN_POINT('Ctrl Pts',(13.5572326810556,-0.446936825808157,
27.4015632255082));
#40942=CARTESIAN_POINT('Ctrl Pts',(13.5678418839539,-0.592860063464017,
27.313071780965));
#40943=CARTESIAN_POINT('Ctrl Pts',(13.5784510868521,-0.708642916014393,
27.1950193943343));
#40944=CARTESIAN_POINT('Ctrl Pts',(13.5890602897504,-0.824425768564771,
27.0769670077037));
#40945=CARTESIAN_POINT('Ctrl Pts',(13.5996694926487,-0.910068236009666,
26.9293536789855));
#40946=CARTESIAN_POINT('Ctrl Pts',(13.610278695547,-0.955088366687774,26.7702460966155));
#40947=CARTESIAN_POINT('Ctrl Pts',(13.6161302044859,-0.979919232834984,
26.6824902633621));
#40948=CARTESIAN_POINT('Ctrl Pts',(13.6219817134249,-0.992392470420054,
26.5912377893801));
#40949=CARTESIAN_POINT('Ctrl Pts',(13.6278332223638,-0.992417767911371,
26.4999920932966));
#40950=CARTESIAN_POINT('Origin',(18.,0.,26.5));
#40951=CARTESIAN_POINT('',(14.1721667776362,-0.992571522832967,26.4995949047598));
#40952=CARTESIAN_POINT('',(14.0278332223638,-0.992555916844723,26.5000186768892));
#40953=CARTESIAN_POINT('',(18.,-0.9925,26.5));
#40954=CARTESIAN_POINT('Ctrl Pts',(14.1721667776362,-0.992571522832967,
26.4995949047598));
#40955=CARTESIAN_POINT('Ctrl Pts',(14.1626362965836,-0.992457550700201,
26.64806001));
#40956=CARTESIAN_POINT('Ctrl Pts',(14.1531058155309,-0.958639467274736,
26.7971838773033));
#40957=CARTESIAN_POINT('Ctrl Pts',(14.1435753344783,-0.894147088982726,
26.9311239446055));
#40958=CARTESIAN_POINT('Ctrl Pts',(14.1329897989778,-0.822515200082955,
27.0798916017197));
#40959=CARTESIAN_POINT('Ctrl Pts',(14.1224042634772,-0.713041613705988,
27.2099275889229));
#40960=CARTESIAN_POINT('Ctrl Pts',(14.1118187279767,-0.579034442518051,
27.3060991855525));
#40961=CARTESIAN_POINT('Ctrl Pts',(14.1012331924762,-0.445027271330115,
27.4022707821822));
#40962=CARTESIAN_POINT('Ctrl Pts',(14.0906476569756,-0.286486515331208,
27.4645779882383));
#40963=CARTESIAN_POINT('Ctrl Pts',(14.0800621214751,-0.122774913851459,
27.4850198549848));
#40964=CARTESIAN_POINT('Ctrl Pts',(14.0694765859746,0.0409366876282946,
27.5054617217313));
#40965=CARTESIAN_POINT('Ctrl Pts',(14.0588910504741,0.209819134588893,27.4840382491683));
#40966=CARTESIAN_POINT('Ctrl Pts',(14.0483055149735,0.363365302276931,27.4236317626303));
#40967=CARTESIAN_POINT('Ctrl Pts',(14.037719979473,0.516911469964969,27.3632252760923));
#40968=CARTESIAN_POINT('Ctrl Pts',(14.0271344439725,0.655121358380448,27.2638357755792));
#40969=CARTESIAN_POINT('Ctrl Pts',(14.0165489084719,0.761020962357605,27.1373263599113));
#40970=CARTESIAN_POINT('Ctrl Pts',(14.0059633729714,0.866920566334765,27.0108169442434));
#40971=CARTESIAN_POINT('Ctrl Pts',(13.9953778374708,0.940509885873604,26.8571876134207));
#40972=CARTESIAN_POINT('Ctrl Pts',(13.9847923019703,0.973068007556158,26.6954876856514));
#40973=CARTESIAN_POINT('Ctrl Pts',(13.9742067664698,1.00562612923871,26.5337877578821));
#40974=CARTESIAN_POINT('Ctrl Pts',(13.9636212309693,0.997153053064983,26.3640172331663));
#40975=CARTESIAN_POINT('Ctrl Pts',(13.9530356954687,0.948218849432393,26.2063200961427));
#40976=CARTESIAN_POINT('Ctrl Pts',(13.9424501599682,0.899284645799801,26.0486229591191));
#40977=CARTESIAN_POINT('Ctrl Pts',(13.9318646244677,0.809889314708351,25.9029992097878));
#40978=CARTESIAN_POINT('Ctrl Pts',(13.9212790889671,0.691785171387141,25.7881666187154));
#40979=CARTESIAN_POINT('Ctrl Pts',(13.9106935534666,0.573681028065935,25.6733340276429));
#40980=CARTESIAN_POINT('Ctrl Pts',(13.9001080179661,0.426868072514974,25.5892925948294));
#40981=CARTESIAN_POINT('Ctrl Pts',(13.8895224824655,0.267722733869405,25.544588084381));
#40982=CARTESIAN_POINT('Ctrl Pts',(13.878936946965,0.108577395223831,25.4998835739326));
#40983=CARTESIAN_POINT('Ctrl Pts',(13.8683514114645,-0.0629003265163543,
25.4945159858495));
#40984=CARTESIAN_POINT('Ctrl Pts',(13.8577658759639,-0.223393305045033,
25.5318493698681));
#40985=CARTESIAN_POINT('Ctrl Pts',(13.8365948049629,-0.544379262102385,
25.6065161379052));
#40986=CARTESIAN_POINT('Ctrl Pts',(13.8154237339618,-0.821426246313716,
25.851986794349));
#40987=CARTESIAN_POINT('Ctrl Pts',(13.7942526629607,-0.934203567068004,
26.161645294637));
#40988=CARTESIAN_POINT('Ctrl Pts',(13.7868907011859,-0.973420398584022,
26.2693249695227));
#40989=CARTESIAN_POINT('Ctrl Pts',(13.7795287394111,-0.992773590522822,
26.3847662978295));
#40990=CARTESIAN_POINT('Ctrl Pts',(13.7721667776362,-0.992441988512883,
26.5000464541839));
#40991=CARTESIAN_POINT('Ctrl Pts',(13.6278332223638,-0.992417767911371,
26.4999920932966));
#40992=CARTESIAN_POINT('Ctrl Pts',(13.6325909163231,-0.992438336575435,
26.4258028368843));
#40993=CARTESIAN_POINT('Ctrl Pts',(13.6373486102825,-0.984229759594754,
26.3516180612386));
#40994=CARTESIAN_POINT('Ctrl Pts',(13.6421063042418,-0.967743493691695,
26.2793208860457));
#40995=CARTESIAN_POINT('Ctrl Pts',(13.6527155071401,-0.930980696106187,
26.1181050938677));
#40996=CARTESIAN_POINT('Ctrl Pts',(13.6633247100383,-0.853057307023846,
25.9662753455335));
#40997=CARTESIAN_POINT('Ctrl Pts',(13.6739339129366,-0.74351052477647,25.8424143854487));
#40998=CARTESIAN_POINT('Ctrl Pts',(13.6845431158349,-0.633963742529094,
25.7185534253638));
#40999=CARTESIAN_POINT('Ctrl Pts',(13.6951523187332,-0.492793567116679,
25.6226612535283));
#41000=CARTESIAN_POINT('Ctrl Pts',(13.7057615216314,-0.337278096646842,
25.5664743032779));
#41001=CARTESIAN_POINT('Ctrl Pts',(13.7163707245297,-0.181762626177006,
25.5102873530275));
#41002=CARTESIAN_POINT('Ctrl Pts',(13.726979927428,-0.011901860649759,25.4938056243621));
#41003=CARTESIAN_POINT('Ctrl Pts',(13.7375891303262,0.151514603528741,25.5190463487831));
#41004=CARTESIAN_POINT('Ctrl Pts',(13.7481983332245,0.314931067707251,25.544287073204));
#41005=CARTESIAN_POINT('Ctrl Pts',(13.7588075361228,0.471903230537002,25.6112502507112));
#41006=CARTESIAN_POINT('Ctrl Pts',(13.7694167390211,0.603218957290428,25.7117401250326));
#41007=CARTESIAN_POINT('Ctrl Pts',(13.7800259419193,0.734534684043851,25.8122299993539));
#41008=CARTESIAN_POINT('Ctrl Pts',(13.7906351448176,0.840193974720952,25.9462465704894));
#41009=CARTESIAN_POINT('Ctrl Pts',(13.8012443477159,0.907264978915181,26.0973872841647));
#41010=CARTESIAN_POINT('Ctrl Pts',(13.8118535506141,0.974335983109407,26.2485279978399));
#41011=CARTESIAN_POINT('Ctrl Pts',(13.8224627535124,1.00281870082077,26.416792854055));
#41012=CARTESIAN_POINT('Ctrl Pts',(13.8330719564107,0.989227075666942,26.5815875829136));
#41013=CARTESIAN_POINT('Ctrl Pts',(13.843681159309,0.975635450513119,26.7463823117722));
#41014=CARTESIAN_POINT('Ctrl Pts',(13.8542903622072,0.919969482494115,26.9077069132743));
#41015=CARTESIAN_POINT('Ctrl Pts',(13.8648995651055,0.829042239978501,27.0458165490801));
#41016=CARTESIAN_POINT('Ctrl Pts',(13.8755087680038,0.738114997462886,27.1839261848858));
#41017=CARTESIAN_POINT('Ctrl Pts',(13.8861179709021,0.611926480450659,27.2988208549953));
#41018=CARTESIAN_POINT('Ctrl Pts',(13.8967271738003,0.465921152126924,27.3764383725733));
#41019=CARTESIAN_POINT('Ctrl Pts',(13.9073363766986,0.319915823803185,27.4540558901513));
#41020=CARTESIAN_POINT('Ctrl Pts',(13.9179455795969,0.154093684167947,27.4943962551979));
#41021=CARTESIAN_POINT('Ctrl Pts',(13.9285547824951,-0.0112499658155442,
27.4925221303263));
#41022=CARTESIAN_POINT('Ctrl Pts',(13.9391639853934,-0.176593615799031,
27.4906480054546));
#41023=CARTESIAN_POINT('Ctrl Pts',(13.9497731882917,-0.341458776130763,
27.4465593906646));
#41024=CARTESIAN_POINT('Ctrl Pts',(13.96038239119,-0.485667272444817,27.3656523790727));
#41025=CARTESIAN_POINT('Ctrl Pts',(13.9709915940882,-0.62987576875887,27.2847453674808));
#41026=CARTESIAN_POINT('Ctrl Pts',(13.9816007969865,-0.75342760105525,27.1670199590869));
#41027=CARTESIAN_POINT('Ctrl Pts',(13.9922099998848,-0.84120101522721,27.0268848004061));
#41028=CARTESIAN_POINT('Ctrl Pts',(14.002819202783,-0.92897442939917,26.8867496417253));
#41029=CARTESIAN_POINT('Ctrl Pts',(14.0134284056813,-0.980969425446714,
26.7242047327576));
#41030=CARTESIAN_POINT('Ctrl Pts',(14.0240376085796,-0.990822232550754,
26.5591442676968));
#41031=CARTESIAN_POINT('Ctrl Pts',(14.0253028131743,-0.991997232872517,
26.5394599180989));
#41032=CARTESIAN_POINT('Ctrl Pts',(14.0265680177691,-0.992572893419552,
26.5197397926465));
#41033=CARTESIAN_POINT('Ctrl Pts',(14.0278332223638,-0.992555916844723,
26.5000186768892));
#41034=CARTESIAN_POINT('Origin',(18.,0.,26.5));
#41035=CARTESIAN_POINT('',(14.5721667776362,-0.992492707894564,26.5000909218272));
#41036=CARTESIAN_POINT('',(14.4278332223638,-0.992459136234123,26.4999764698814));
#41037=CARTESIAN_POINT('',(18.,-0.9925,26.5));
#41038=CARTESIAN_POINT('Ctrl Pts',(14.5721667776362,-0.992492707894564,
26.5000909218272));
#41039=CARTESIAN_POINT('Ctrl Pts',(14.5669149247572,-0.99244755231627,26.5819256581969));
#41040=CARTESIAN_POINT('Ctrl Pts',(14.5616630718781,-0.982361046646003,
26.6637403493712));
#41041=CARTESIAN_POINT('Ctrl Pts',(14.5564112189991,-0.962284559437845,
26.7430744931871));
#41042=CARTESIAN_POINT('Ctrl Pts',(14.5458256834985,-0.921818770893843,
26.9029788955205));
#41043=CARTESIAN_POINT('Ctrl Pts',(14.535240147998,-0.840768010570442,27.0528059074049));
#41044=CARTESIAN_POINT('Ctrl Pts',(14.5246546124975,-0.728778863616166,
27.1739578340904));
#41045=CARTESIAN_POINT('Ctrl Pts',(14.5140690769969,-0.616789716661883,
27.2951097607759));
#41046=CARTESIAN_POINT('Ctrl Pts',(14.5034835414964,-0.473862183076721,
27.3875866022624));
#41047=CARTESIAN_POINT('Ctrl Pts',(14.4928980059959,-0.317532787833618,
27.4403738110395));
#41048=CARTESIAN_POINT('Ctrl Pts',(14.4823124704953,-0.161203392590524,
27.4931610198166));
#41049=CARTESIAN_POINT('Ctrl Pts',(14.4717269349948,0.00852786431050967,
27.5062585958844));
#41050=CARTESIAN_POINT('Ctrl Pts',(14.4611413994943,0.171036982825635,27.4777955536263));
#41051=CARTESIAN_POINT('Ctrl Pts',(14.4505558639937,0.333546101340761,27.4493325113683));
#41052=CARTESIAN_POINT('Ctrl Pts',(14.4399703284932,0.488833081469978,27.3793088507844));
#41053=CARTESIAN_POINT('Ctrl Pts',(14.4293847929927,0.617951802230289,27.2766674659666));
#41054=CARTESIAN_POINT('Ctrl Pts',(14.4187992574921,0.7470705229906,27.1740260811488));
#41055=CARTESIAN_POINT('Ctrl Pts',(14.4082137219916,0.850020984382004,27.0387669720972));
#41056=CARTESIAN_POINT('Ctrl Pts',(14.3976281864911,0.914254878263044,26.8866586219403));
#41057=CARTESIAN_POINT('Ctrl Pts',(14.3870426509905,0.978488772144085,26.7345502717833));
#41058=CARTESIAN_POINT('Ctrl Pts',(14.37645711549,1.00400609851476,26.565592680521));
#41059=CARTESIAN_POINT('Ctrl Pts',(14.3658715799895,0.987727198252969,26.4016716323048));
#41060=CARTESIAN_POINT('Ctrl Pts',(14.355286044489,0.971448297991179,26.2377505840885));
#41061=CARTESIAN_POINT('Ctrl Pts',(14.3447005089884,0.913373171096924,26.0788660789183));
#41062=CARTESIAN_POINT('Ctrl Pts',(14.3341149734879,0.820514056354027,25.9421074708667));
#41063=CARTESIAN_POINT('Ctrl Pts',(14.3235294379874,0.72765494161113,25.8053488628151));
#41064=CARTESIAN_POINT('Ctrl Pts',(14.3129439024868,0.600011839019592,25.6907161518822));
#41065=CARTESIAN_POINT('Ctrl Pts',(14.3023583669863,0.453243444191403,25.6158107715758));
#41066=CARTESIAN_POINT('Ctrl Pts',(14.2811872959852,0.159706654535029,25.4660000109631));
#41067=CARTESIAN_POINT('Ctrl Pts',(14.2600162249842,-0.210331304067943,
25.4750985728568));
#41068=CARTESIAN_POINT('Ctrl Pts',(14.2388451539831,-0.496150677754313,
25.6391546501678));
#41069=CARTESIAN_POINT('Ctrl Pts',(14.2282596184826,-0.639060364597492,
25.7211826888233));
#41070=CARTESIAN_POINT('Ctrl Pts',(14.217674082982,-0.760915405211523,25.841950106333));
#41071=CARTESIAN_POINT('Ctrl Pts',(14.2070885474815,-0.84694107800222,25.9831071666876));
#41072=CARTESIAN_POINT('Ctrl Pts',(14.196503011981,-0.932966750792924,26.1242642270422));
#41073=CARTESIAN_POINT('Ctrl Pts',(14.1859174764804,-0.983163055760287,
26.2858109302416));
#41074=CARTESIAN_POINT('Ctrl Pts',(14.1753319409799,-0.991366112532681,
26.4503339453539));
#41075=CARTESIAN_POINT('Ctrl Pts',(14.174276886532,-0.992183706648124,26.4667318629526));
#41076=CARTESIAN_POINT('Ctrl Pts',(14.1732218320841,-0.992584139909162,
26.4831593472286));
#41077=CARTESIAN_POINT('Ctrl Pts',(14.1721667776362,-0.992571522832967,
26.4995949047598));
#41078=CARTESIAN_POINT('Ctrl Pts',(14.0278332223638,-0.992555916844723,
26.5000186768892));
#41079=CARTESIAN_POINT('Ctrl Pts',(14.0371772206673,-0.992430538635496,
26.3543710299033));
#41080=CARTESIAN_POINT('Ctrl Pts',(14.0465212189709,-0.959980584759993,
26.208669368106));
#41081=CARTESIAN_POINT('Ctrl Pts',(14.0558652172744,-0.89790604859668,26.0769261662407));
#41082=CARTESIAN_POINT('Ctrl Pts',(14.0664744201727,-0.827426439378023,
25.9273445509992));
#41083=CARTESIAN_POINT('Ctrl Pts',(14.077083623071,-0.718756602780171,25.7957573416698));
#41084=CARTESIAN_POINT('Ctrl Pts',(14.0876928259692,-0.585196855903322,
25.6982697581112));
#41085=CARTESIAN_POINT('Ctrl Pts',(14.0983020288675,-0.451637109026474,
25.6007821745526));
#41086=CARTESIAN_POINT('Ctrl Pts',(14.1089112317658,-0.29318745187063,25.5373942167648));
#41087=CARTESIAN_POINT('Ctrl Pts',(14.119520434664,-0.129240852627964,25.5158640627788));
#41088=CARTESIAN_POINT('Ctrl Pts',(14.1301296375623,0.0347057466146934,
25.4943339087927));
#41089=CARTESIAN_POINT('Ctrl Pts',(14.1407388404606,0.20414928794417,25.5146615586084));
#41090=CARTESIAN_POINT('Ctrl Pts',(14.1513480433589,0.358351239852387,25.5743590707977));
#41091=CARTESIAN_POINT('Ctrl Pts',(14.1619572462571,0.512553191760612,25.634056582987));
#41092=CARTESIAN_POINT('Ctrl Pts',(14.1725664491554,0.651513554247573,25.73312395755));
#41093=CARTESIAN_POINT('Ctrl Pts',(14.1831756520537,0.7582246925979,25.8594361417836));
#41094=CARTESIAN_POINT('Ctrl Pts',(14.193784854952,0.864935830948223,25.9857483260173));
#41095=CARTESIAN_POINT('Ctrl Pts',(14.2043940578502,0.939397745161913,26.1393053199216));
#41096=CARTESIAN_POINT('Ctrl Pts',(14.2150032607485,0.972496893690223,26.3013129780758));
#41097=CARTESIAN_POINT('Ctrl Pts',(14.2256124636468,1.00559604221853,26.4633206362299));
#41098=CARTESIAN_POINT('Ctrl Pts',(14.236221666545,0.997332425061462,26.6337789586339));
#41099=CARTESIAN_POINT('Ctrl Pts',(14.2468308694433,0.948717442732942,26.7918252127088));
#41100=CARTESIAN_POINT('Ctrl Pts',(14.2574400723416,0.900102460404423,26.9498714667836));
#41101=CARTESIAN_POINT('Ctrl Pts',(14.2680492752399,0.811136112904449,27.0955056525294));
#41102=CARTESIAN_POINT('Ctrl Pts',(14.2786584781381,0.692707168174913,27.2109033127489));
#41103=CARTESIAN_POINT('Ctrl Pts',(14.2892676810364,0.574278223445373,27.3263009729684));
#41104=CARTESIAN_POINT('Ctrl Pts',(14.2998768839347,0.426386681486266,27.4114621076618));
#41105=CARTESIAN_POINT('Ctrl Pts',(14.3104860868329,0.267133281804292,27.455963676439));
#41106=CARTESIAN_POINT('Ctrl Pts',(14.3210952897312,0.107879882122317,27.5004652452162));
#41107=CARTESIAN_POINT('Ctrl Pts',(14.3317044926295,-0.0627353752825216,
27.5043072480772));
#41108=CARTESIAN_POINT('Ctrl Pts',(14.3423136955278,-0.22383055024486,27.4670194546623));
#41109=CARTESIAN_POINT('Ctrl Pts',(14.352922898426,-0.384925725207203,27.4297316612474));
#41110=CARTESIAN_POINT('Ctrl Pts',(14.3635321013243,-0.536500817727043,
27.3513140715566));
#41111=CARTESIAN_POINT('Ctrl Pts',(14.3741413042226,-0.660004251229673,
27.2413643701157));
#41112=CARTESIAN_POINT('Ctrl Pts',(14.3847505071209,-0.783507684732299,
27.1314146686747));
#41113=CARTESIAN_POINT('Ctrl Pts',(14.3953597100191,-0.878939459217715,
26.9899328554835));
#41114=CARTESIAN_POINT('Ctrl Pts',(14.4059689129174,-0.934619490296102,
26.8342351706163));
#41115=CARTESIAN_POINT('Ctrl Pts',(14.4132570160662,-0.972869471347363,
26.727277013795));
#41116=CARTESIAN_POINT('Ctrl Pts',(14.420545119215,-0.992360020119326,26.6136101780797));
#41117=CARTESIAN_POINT('Ctrl Pts',(14.4278332223638,-0.992459136234123,
26.4999764698814));
#41118=CARTESIAN_POINT('Origin',(18.,0.,26.5));
#41119=CARTESIAN_POINT('',(14.9721667776363,-0.992543902023409,26.5000135256884));
#41120=CARTESIAN_POINT('',(14.8278332223638,-0.992487339104761,26.5000259875884));
#41121=CARTESIAN_POINT('',(18.,-0.9925,26.5));
#41122=CARTESIAN_POINT('Ctrl Pts',(14.9721667776362,-0.992609386691394,
26.5000337007337));
#41123=CARTESIAN_POINT('Ctrl Pts',(14.9711935529308,-0.992625808208597,
26.5152038908542));
#41124=CARTESIAN_POINT('Ctrl Pts',(14.9702203282253,-0.992289639355945,
26.530373213192));
#41125=CARTESIAN_POINT('Ctrl Pts',(14.9692471035198,-0.99159729580047,26.5455257855143));
#41126=CARTESIAN_POINT('Ctrl Pts',(14.9586615680193,-0.98406683829784,26.7103367395949));
#41127=CARTESIAN_POINT('Ctrl Pts',(14.9480760325187,-0.934399490014543,
26.873166099916));
#41128=CARTESIAN_POINT('Ctrl Pts',(14.9374904970182,-0.848903141093112,
27.0142892502091));
#41129=CARTESIAN_POINT('Ctrl Pts',(14.9269049615177,-0.763406792171678,
27.1554124005022));
#41130=CARTESIAN_POINT('Ctrl Pts',(14.9163194260172,-0.642081442612108,
27.2748293407674));
#41131=CARTESIAN_POINT('Ctrl Pts',(14.9057338905166,-0.499489145232929,
27.3578160571941));
#41132=CARTESIAN_POINT('Ctrl Pts',(14.8951483550161,-0.356896847853745,
27.4408027736207));
#41133=CARTESIAN_POINT('Ctrl Pts',(14.8845628195156,-0.193037602654965,
27.4873592662088));
#41134=CARTESIAN_POINT('Ctrl Pts',(14.873977284015,-0.0281609175057919,
27.4921107525352));
#41135=CARTESIAN_POINT('Ctrl Pts',(14.8633917485145,0.136715767643367,27.4968622388615));
#41136=CARTESIAN_POINT('Ctrl Pts',(14.852806213014,0.302609892742916,27.4598087189262));
#41137=CARTESIAN_POINT('Ctrl Pts',(14.8422206775134,0.449763830553274,27.384917718816));
#41138=CARTESIAN_POINT('Ctrl Pts',(14.8316351420129,0.596917768363644,27.3100267187059));
#41139=CARTESIAN_POINT('Ctrl Pts',(14.8210496065124,0.725331518884833,27.197298238421));
#41140=CARTESIAN_POINT('Ctrl Pts',(14.8104640710118,0.818543675128617,27.0614799533102));
#41141=CARTESIAN_POINT('Ctrl Pts',(14.7998785355113,0.911755831372396,26.9256616681994));
#41142=CARTESIAN_POINT('Ctrl Pts',(14.7892930000108,0.969766393338773,26.7667535782628));
#41143=CARTESIAN_POINT('Ctrl Pts',(14.7787074645102,0.986921312052431,26.6023411674448));
#41144=CARTESIAN_POINT('Ctrl Pts',(14.7681219290097,1.00407623076609,26.4379287566269));
#41145=CARTESIAN_POINT('Ctrl Pts',(14.7575363935092,0.980375506227025,26.2680120249276));
#41146=CARTESIAN_POINT('Ctrl Pts',(14.7469508580086,0.916445647298258,26.1161411888312));
#41147=CARTESIAN_POINT('Ctrl Pts',(14.7257797870076,0.788585929440723,25.8123995166384));
#41148=CARTESIAN_POINT('Ctrl Pts',(14.7046087160065,0.49980967402437,25.5808414268568));
#41149=CARTESIAN_POINT('Ctrl Pts',(14.6834376450054,0.175541983023264,25.5220402750828));
#41150=CARTESIAN_POINT('Ctrl Pts',(14.6728521095049,0.013408137522709,25.4926396991958));
#41151=CARTESIAN_POINT('Ctrl Pts',(14.6622665740044,-0.157598566874034,
25.5064283578108));
#41152=CARTESIAN_POINT('Ctrl Pts',(14.6516810385039,-0.31435451270915,25.5589003075781));
#41153=CARTESIAN_POINT('Ctrl Pts',(14.6410955030033,-0.47111045854426,25.6113722573453));
#41154=CARTESIAN_POINT('Ctrl Pts',(14.6305099675028,-0.613615645817744,
25.702527498265));
#41155=CARTESIAN_POINT('Ctrl Pts',(14.6199244320022,-0.725933430857789,
25.8230257464088));
#41156=CARTESIAN_POINT('Ctrl Pts',(14.6093388965017,-0.838251215897837,
25.9435239945527));
#41157=CARTESIAN_POINT('Ctrl Pts',(14.5987533610012,-0.920381598704446,
26.0933652499209));
#41158=CARTESIAN_POINT('Ctrl Pts',(14.5881678255007,-0.961506381725449,
26.2532767739961));
#41159=CARTESIAN_POINT('Ctrl Pts',(14.5828341428792,-0.982227727424042,
26.3338506209113));
#41160=CARTESIAN_POINT('Ctrl Pts',(14.5775004602577,-0.992538567047276,
26.4169811087267));
#41161=CARTESIAN_POINT('Ctrl Pts',(14.5721667776362,-0.992492707894564,
26.5000909218272));
#41162=CARTESIAN_POINT('Ctrl Pts',(14.4278332223638,-0.992459136234123,
26.4999764698814));
#41163=CARTESIAN_POINT('Ctrl Pts',(14.4311543221133,-0.992504302239228,
26.4481949744602));
#41164=CARTESIAN_POINT('Ctrl Pts',(14.4344754218628,-0.988522810522003,
26.3964203580136));
#41165=CARTESIAN_POINT('Ctrl Pts',(14.4377965216122,-0.980454858551326,
26.3452905585901));
#41166=CARTESIAN_POINT('Ctrl Pts',(14.4484057245105,-0.954681908056806,
26.1819571879744));
#41167=CARTESIAN_POINT('Ctrl Pts',(14.4590149274088,-0.887207719396409,
26.0252040032861));
#41168=CARTESIAN_POINT('Ctrl Pts',(14.469624130307,-0.786290592512034,25.8942163380832));
#41169=CARTESIAN_POINT('Ctrl Pts',(14.4802333332053,-0.685373465627659,
25.7632286728803));
#41170=CARTESIAN_POINT('Ctrl Pts',(14.4908425361036,-0.551013400519304,
25.6580065271629));
#41171=CARTESIAN_POINT('Ctrl Pts',(14.5014517390018,-0.399654992370801,
25.5914282482977));
#41172=CARTESIAN_POINT('Ctrl Pts',(14.5120609419001,-0.248296584222298,
25.5248499694325));
#41173=CARTESIAN_POINT('Ctrl Pts',(14.5226701447984,-0.0799398330336454,
25.4969155574197));
#41174=CARTESIAN_POINT('Ctrl Pts',(14.5332793476967,0.0848097440905795,
25.5110439604181));
#41175=CARTESIAN_POINT('Ctrl Pts',(14.5438885505949,0.249559321214804,25.5251723634165));
#41176=CARTESIAN_POINT('Ctrl Pts',(14.5544977534932,0.410701724274602,25.5813635814262));
#41177=CARTESIAN_POINT('Ctrl Pts',(14.5651069563915,0.548514414559299,25.6727402596893));
#41178=CARTESIAN_POINT('Ctrl Pts',(14.5757161592898,0.686327104843997,25.7641169379523));
#41179=CARTESIAN_POINT('Ctrl Pts',(14.586325362188,0.800810082353595,25.8906790764687));
#41180=CARTESIAN_POINT('Ctrl Pts',(14.5969345650863,0.877951548127839,26.0369364837755));
#41181=CARTESIAN_POINT('Ctrl Pts',(14.6075437679846,0.955093013902084,26.1831938910823));
#41182=CARTESIAN_POINT('Ctrl Pts',(14.6181529708829,0.994892967940975,26.3491465671794));
#41183=CARTESIAN_POINT('Ctrl Pts',(14.6287621737811,0.992480214834056,26.5144832344869));
#41184=CARTESIAN_POINT('Ctrl Pts',(14.6393713766794,0.990067461727136,26.6798199017944));
#41185=CARTESIAN_POINT('Ctrl Pts',(14.6499805795777,0.945442001474406,26.8445405603122));
#41186=CARTESIAN_POINT('Ctrl Pts',(14.6605897824759,0.864065632774431,26.9884847215383));
#41187=CARTESIAN_POINT('Ctrl Pts',(14.6711989853742,0.782689264074457,27.1324288827645));
#41188=CARTESIAN_POINT('Ctrl Pts',(14.6818081882725,0.664561986927239,27.255596546699));
#41189=CARTESIAN_POINT('Ctrl Pts',(14.6924173911708,0.524141633362612,27.3429129783639));
#41190=CARTESIAN_POINT('Ctrl Pts',(14.703026594069,0.38372127979798,27.4302294100287));
#41191=CARTESIAN_POINT('Ctrl Pts',(14.7136357969673,0.221007849815937,27.4816946094239));
#41192=CARTESIAN_POINT('Ctrl Pts',(14.7242449998656,0.0559161632319498,
27.4910096485946));
#41193=CARTESIAN_POINT('Ctrl Pts',(14.7348542027638,-0.109175523352037,
27.5003246877654));
#41194=CARTESIAN_POINT('Ctrl Pts',(14.7454634056621,-0.276645466537967,
27.4674895667118));
#41195=CARTESIAN_POINT('Ctrl Pts',(14.7560726085604,-0.425996687413761,
27.3965230411042));
#41196=CARTESIAN_POINT('Ctrl Pts',(14.7666818114587,-0.57534790828955,27.3255565154967));
#41197=CARTESIAN_POINT('Ctrl Pts',(14.7772910143569,-0.706580406855203,
27.2164585853352));
#41198=CARTESIAN_POINT('Ctrl Pts',(14.7879002172552,-0.803632377006842,
27.0825819629414));
#41199=CARTESIAN_POINT('Ctrl Pts',(14.7985094201535,-0.900684347158478,
26.9487053405475));
#41200=CARTESIAN_POINT('Ctrl Pts',(14.8091186230517,-0.963555788896102,
26.7900500259213));
#41201=CARTESIAN_POINT('Ctrl Pts',(14.81972782595,-0.984551741613934,26.6260341580811));
#41202=CARTESIAN_POINT('Ctrl Pts',(14.8224296247546,-0.989898688080915,
26.5842649620431));
#41203=CARTESIAN_POINT('Ctrl Pts',(14.8251314235592,-0.992529818241405,
26.5421481096989));
#41204=CARTESIAN_POINT('Ctrl Pts',(14.8278332223638,-0.992487339104761,
26.5000259875884));
#41205=CARTESIAN_POINT('Origin',(18.,0.,26.5));
#41206=CARTESIAN_POINT('',(15.3721667776362,-0.9925,26.4999999999999));
#41207=CARTESIAN_POINT('',(15.2278332223638,-0.992527725525489,26.4999759343258));
#41208=CARTESIAN_POINT('',(18.,-0.9925,26.5));
#41209=CARTESIAN_POINT('Ctrl Pts',(15.3721667776362,-0.9925,26.4999999999999));
#41210=CARTESIAN_POINT('Ctrl Pts',(15.3554259338597,-0.992500000000016,
26.7609923249228));
#41211=CARTESIAN_POINT('Ctrl Pts',(15.3386850900832,-0.884539443097445,
27.0203491301746));
#41212=CARTESIAN_POINT('Ctrl Pts',(15.3219442463066,-0.699346033936964,
27.2042523516586));
#41213=CARTESIAN_POINT('Ctrl Pts',(15.3052034025301,-0.514152624776482,
27.3881555731425));
#41214=CARTESIAN_POINT('Ctrl Pts',(15.2884625587536,-0.254047408344541,
27.4943003359056));
#41215=CARTESIAN_POINT('Ctrl Pts',(15.271721714977,0.00693853867338895,
27.4924757461425));
#41216=CARTESIAN_POINT('Ctrl Pts',(15.2549808712005,0.267924485691319,27.4906511563793));
#41217=CARTESIAN_POINT('Ctrl Pts',(15.238240027424,0.526520203887957,27.3808800818309));
#41218=CARTESIAN_POINT('Ctrl Pts',(15.2214991836474,0.709124249559236,27.1944055361869));
#41219=CARTESIAN_POINT('Ctrl Pts',(15.2047583398709,0.891728295230515,27.0079309905429));
#41220=CARTESIAN_POINT('Ctrl Pts',(15.1880174960944,0.996052076106157,26.747090075384));
#41221=CARTESIAN_POINT('Ctrl Pts',(15.1712766523178,0.99240298575532,26.4861232617692));
#41222=CARTESIAN_POINT('Ctrl Pts',(15.1545358085413,0.988753895404483,26.2251564481544));
#41223=CARTESIAN_POINT('Ctrl Pts',(15.1377949647648,0.877177668191593,25.9673344556904));
#41224=CARTESIAN_POINT('Ctrl Pts',(15.1210541209882,0.68943109987178,25.7860385104716));
#41225=CARTESIAN_POINT('Ctrl Pts',(15.1043132772117,0.501684531551967,25.6047425652528));
#41226=CARTESIAN_POINT('Ctrl Pts',(15.0875724334352,0.240120666075862,25.5022448650135));
#41227=CARTESIAN_POINT('Ctrl Pts',(15.0708315896586,-0.0208142595727541,
25.5077182776054));
#41228=CARTESIAN_POINT('Ctrl Pts',(15.0540907458821,-0.28174918522137,25.5131916901973));
#41229=CARTESIAN_POINT('Ctrl Pts',(15.0373499021056,-0.538784851090443,
25.6265676168677));
#41230=CARTESIAN_POINT('Ctrl Pts',(15.020609058329,-0.718763835149441,25.8155770318865));
#41231=CARTESIAN_POINT('Ctrl Pts',(15.0044616314314,-0.892363059118749,
25.9978865828694));
#41232=CARTESIAN_POINT('Ctrl Pts',(14.9883142045338,-0.992499999999987,
26.2482591353349));
#41233=CARTESIAN_POINT('Ctrl Pts',(14.9721667776362,-0.9925,26.4999999999999));
#41234=CARTESIAN_POINT('Ctrl Pts',(14.8278332223638,-0.992487339104761,
26.5000259875884));
#41235=CARTESIAN_POINT('Ctrl Pts',(14.8357406264575,-0.992363014636773,
26.3767464005799));
#41236=CARTESIAN_POINT('Ctrl Pts',(14.8436480305512,-0.969337407946782,
26.2534216744387));
#41237=CARTESIAN_POINT('Ctrl Pts',(14.8515554346448,-0.92446862061909,26.1386352114429));
#41238=CARTESIAN_POINT('Ctrl Pts',(14.8621646375431,-0.864269083208378,
25.9846285536991));
#41239=CARTESIAN_POINT('Ctrl Pts',(14.8727738404414,-0.764749544688916,
25.8459916592655));
#41240=CARTESIAN_POINT('Ctrl Pts',(14.8833830433397,-0.638090399008227,
25.7396925729603));
#41241=CARTESIAN_POINT('Ctrl Pts',(14.8939922462379,-0.511431253327537,
25.633393486655));
#41242=CARTESIAN_POINT('Ctrl Pts',(14.9046014491362,-0.35763250048562,25.559432208478));
#41243=CARTESIAN_POINT('Ctrl Pts',(14.9152106520345,-0.195517875259795,
25.5268610061393));
#41244=CARTESIAN_POINT('Ctrl Pts',(14.9258198549328,-0.0334032500339701,
25.4942898038006));
#41245=CARTESIAN_POINT('Ctrl Pts',(14.936429057831,0.137027247575762,25.5031086773003));
#41246=CARTESIAN_POINT('Ctrl Pts',(14.9470382607293,0.294914290522258,25.5522382671979));
#41247=CARTESIAN_POINT('Ctrl Pts',(14.9576474636276,0.452801333468754,25.6013678570955));
#41248=CARTESIAN_POINT('Ctrl Pts',(14.9682566665258,0.598144921752012,25.6908081633911));
#41249=CARTESIAN_POINT('Ctrl Pts',(14.9788658694241,0.713156164975501,25.8096124093846));
#41250=CARTESIAN_POINT('Ctrl Pts',(14.9894750723224,0.82816740819899,25.9284166553781));
#41251=CARTESIAN_POINT('Ctrl Pts',(15.0000842752207,0.91284630636271,26.0765848410695));
#41252=CARTESIAN_POINT('Ctrl Pts',(15.0106934781189,0.956828840963156,26.2359823679764));
#41253=CARTESIAN_POINT('Ctrl Pts',(15.0213026810172,1.0008113755636,26.3953798948832));
#41254=CARTESIAN_POINT('Ctrl Pts',(15.0319118839155,1.00409754660077,26.5660067630055));
#41255=CARTESIAN_POINT('Ctrl Pts',(15.0425210868137,0.966285153075671,26.7269796111191));
#41256=CARTESIAN_POINT('Ctrl Pts',(15.053130289712,0.928472759550572,26.8879524592327));
#41257=CARTESIAN_POINT('Ctrl Pts',(15.0637394926103,0.849561801463207,27.0392712873376));
#41258=CARTESIAN_POINT('Ctrl Pts',(15.0743486955086,0.739210347677032,27.1624158835697));
#41259=CARTESIAN_POINT('Ctrl Pts',(15.0849578984068,0.628858893890858,27.2855604798019));
#41260=CARTESIAN_POINT('Ctrl Pts',(15.0955671013051,0.487066944405874,27.3805308441612));
#41261=CARTESIAN_POINT('Ctrl Pts',(15.1061763042034,0.331188697493168,27.4357033651596));
#41262=CARTESIAN_POINT('Ctrl Pts',(15.1167855071017,0.175310450580462,27.490875886158));
#41263=CARTESIAN_POINT('Ctrl Pts',(15.1273947099999,0.00534590624003523,
27.5062505637954));
#41264=CARTESIAN_POINT('Ctrl Pts',(15.1380039128982,-0.1579026374269,27.4799456607445));
#41265=CARTESIAN_POINT('Ctrl Pts',(15.1486131157965,-0.321151181093836,
27.4536407576935));
#41266=CARTESIAN_POINT('Ctrl Pts',(15.1592223186947,-0.47768372408728,27.3856562739541));
#41267=CARTESIAN_POINT('Ctrl Pts',(15.169831521593,-0.608341937624443,27.2843129654963));
#41268=CARTESIAN_POINT('Ctrl Pts',(15.1804407244913,-0.739000151161607,
27.1829696570385));
#41269=CARTESIAN_POINT('Ctrl Pts',(15.1910499273896,-0.84378403524249,27.0482675238623));
#41270=CARTESIAN_POINT('Ctrl Pts',(15.2016591302878,-0.909868882212257,
26.8966930275415));
#41271=CARTESIAN_POINT('Ctrl Pts',(15.2103838276465,-0.964215122484324,
26.7720426065467));
#41272=CARTESIAN_POINT('Ctrl Pts',(15.2191085250052,-0.992389454393167,
26.6359815155442));
#41273=CARTESIAN_POINT('Ctrl Pts',(15.2278332223638,-0.992527725525489,
26.4999759343258));
#41274=CARTESIAN_POINT('Origin',(18.,0.,26.5));
#41275=CARTESIAN_POINT('',(15.7721667776362,-0.99246122082366,26.5000241305601));
#41276=CARTESIAN_POINT('',(15.6278332223638,-0.992430455435604,26.5000159512924));
#41277=CARTESIAN_POINT('',(18.,-0.9925,26.5));
#41278=CARTESIAN_POINT('Ctrl Pts',(15.7721667776362,-0.9925,26.4999999999999));
#41279=CARTESIAN_POINT('Ctrl Pts',(15.7554259338597,-0.992500000000018,
26.7609923249228));
#41280=CARTESIAN_POINT('Ctrl Pts',(15.7386850900832,-0.884539443097449,
27.0203491301746));
#41281=CARTESIAN_POINT('Ctrl Pts',(15.7219442463066,-0.699346033936969,
27.2042523516586));
#41282=CARTESIAN_POINT('Ctrl Pts',(15.7052034025301,-0.514152624776489,
27.3881555731425));
#41283=CARTESIAN_POINT('Ctrl Pts',(15.6884625587536,-0.254047408344548,
27.4943003359056));
#41284=CARTESIAN_POINT('Ctrl Pts',(15.671721714977,0.00693853867338218,
27.4924757461425));
#41285=CARTESIAN_POINT('Ctrl Pts',(15.6549808712005,0.267924485691312,27.4906511563793));
#41286=CARTESIAN_POINT('Ctrl Pts',(15.638240027424,0.526520203887951,27.3808800818309));
#41287=CARTESIAN_POINT('Ctrl Pts',(15.6214991836474,0.709124249559231,27.1944055361869));
#41288=CARTESIAN_POINT('Ctrl Pts',(15.6047583398709,0.891728295230511,27.0079309905429));
#41289=CARTESIAN_POINT('Ctrl Pts',(15.5880174960944,0.996052076106155,26.747090075384));
#41290=CARTESIAN_POINT('Ctrl Pts',(15.5712766523178,0.99240298575532,26.4861232617692));
#41291=CARTESIAN_POINT('Ctrl Pts',(15.5545358085413,0.988753895404485,26.2251564481544));
#41292=CARTESIAN_POINT('Ctrl Pts',(15.5377949647648,0.877177668191597,25.9673344556904));
#41293=CARTESIAN_POINT('Ctrl Pts',(15.5210541209882,0.689431099871785,25.7860385104716));
#41294=CARTESIAN_POINT('Ctrl Pts',(15.5043132772117,0.501684531551973,25.6047425652528));
#41295=CARTESIAN_POINT('Ctrl Pts',(15.4875724334352,0.240120666075869,25.5022448650135));
#41296=CARTESIAN_POINT('Ctrl Pts',(15.4708315896586,-0.0208142595727472,
25.5077182776054));
#41297=CARTESIAN_POINT('Ctrl Pts',(15.4540907458821,-0.281749185221363,
25.5131916901973));
#41298=CARTESIAN_POINT('Ctrl Pts',(15.4373499021056,-0.538784851090437,
25.6265676168677));
#41299=CARTESIAN_POINT('Ctrl Pts',(15.420609058329,-0.718763835149436,25.8155770318865));
#41300=CARTESIAN_POINT('Ctrl Pts',(15.4044616314314,-0.892363059118746,
25.9978865828694));
#41301=CARTESIAN_POINT('Ctrl Pts',(15.3883142045338,-0.992499999999985,
26.2482591353348));
#41302=CARTESIAN_POINT('Ctrl Pts',(15.3721667776362,-0.9925,26.4999999999999));
#41303=CARTESIAN_POINT('Ctrl Pts',(15.2278332223638,-0.992527725525489,
26.4999759343258));
#41304=CARTESIAN_POINT('Ctrl Pts',(15.2297177279034,-0.992557591629048,
26.4705991822521));
#41305=CARTESIAN_POINT('Ctrl Pts',(15.231602233443,-0.991279447663092,26.4412250199629));
#41306=CARTESIAN_POINT('Ctrl Pts',(15.2334867389827,-0.988674508136253,
26.4119689947814));
#41307=CARTESIAN_POINT('Ctrl Pts',(15.2440959418809,-0.974009477231833,
26.2472663178072));
#41308=CARTESIAN_POINT('Ctrl Pts',(15.2547051447792,-0.917293605564346,
26.086307823324));
#41309=CARTESIAN_POINT('Ctrl Pts',(15.2653143476775,-0.825468461294819,
25.9487935411066));
#41310=CARTESIAN_POINT('Ctrl Pts',(15.2759235505757,-0.733643317025287,
25.8112792588891));
#41311=CARTESIAN_POINT('Ctrl Pts',(15.286532753474,-0.606708900153712,25.6972091889375));
#41312=CARTESIAN_POINT('Ctrl Pts',(15.2971419563723,-0.460200966030206,
25.6205445936359));
#41313=CARTESIAN_POINT('Ctrl Pts',(15.3077511592706,-0.313693031906705,
25.5438799983342));
#41314=CARTESIAN_POINT('Ctrl Pts',(15.3183603621688,-0.147611580531275,
25.5046208776827));
#41315=CARTESIAN_POINT('Ctrl Pts',(15.3289695650671,0.0177163494539894,
25.5075722334193));
#41316=CARTESIAN_POINT('Ctrl Pts',(15.3395787679654,0.183044279439254,25.510523589156));
#41317=CARTESIAN_POINT('Ctrl Pts',(15.3501879708637,0.347618688034365,25.5556854212809));
#41318=CARTESIAN_POINT('Ctrl Pts',(15.3607971737619,0.491296986555805,25.6375302834769));
#41319=CARTESIAN_POINT('Ctrl Pts',(15.3714063766602,0.634975285077253,25.7193751456729));
#41320=CARTESIAN_POINT('Ctrl Pts',(15.3820155795585,0.757757473525031,25.83790303794));
#41321=CARTESIAN_POINT('Ctrl Pts',(15.3926247824567,0.844615996031423,25.9786070961682));
#41322=CARTESIAN_POINT('Ctrl Pts',(15.403233985355,0.931474518537809,26.1193111543965));
#41323=CARTESIAN_POINT('Ctrl Pts',(15.4138431882533,0.9824093751028,26.282191378586));
#41324=CARTESIAN_POINT('Ctrl Pts',(15.4244523911516,0.991186547483833,26.4473125346469));
#41325=CARTESIAN_POINT('Ctrl Pts',(15.4350615940498,0.999963719864865,26.6124336907078));
#41326=CARTESIAN_POINT('Ctrl Pts',(15.4456707969481,0.966583208061936,26.7797957786401));
#41327=CARTESIAN_POINT('Ctrl Pts',(15.4562799998464,0.895130519202377,26.9289150201505));
#41328=CARTESIAN_POINT('Ctrl Pts',(15.4668892027446,0.823677830342816,27.0780342616609));
#41329=CARTESIAN_POINT('Ctrl Pts',(15.4774984056429,0.714152964426622,27.2089106567494));
#41330=CARTESIAN_POINT('Ctrl Pts',(15.4881076085412,0.579960887290202,27.3055259835237));
#41331=CARTESIAN_POINT('Ctrl Pts',(15.4987168114395,0.445768810153782,27.402141310298));
#41332=CARTESIAN_POINT('Ctrl Pts',(15.5093260143377,0.286909521797139,27.4644955687583));
#41333=CARTESIAN_POINT('Ctrl Pts',(15.519935217236,0.122826125988562,27.4849570973869));
#41334=CARTESIAN_POINT('Ctrl Pts',(15.5305444201343,-0.0412572698200145,
27.5054186260156));
#41335=CARTESIAN_POINT('Ctrl Pts',(15.5411536230325,-0.210564773080522,
27.4839874248128));
#41336=CARTESIAN_POINT('Ctrl Pts',(15.5517628259308,-0.364374502254287,
27.4232865010522));
#41337=CARTESIAN_POINT('Ctrl Pts',(15.5623720288291,-0.518184231428048,
27.3625855772916));
#41338=CARTESIAN_POINT('Ctrl Pts',(15.5729812317274,-0.656496186515066,
27.2626149309732));
#41339=CARTESIAN_POINT('Ctrl Pts',(15.5835904346256,-0.762382092669272,
27.135610168024));
#41340=CARTESIAN_POINT('Ctrl Pts',(15.5941996375239,-0.868267998823484,
27.0086054050747));
#41341=CARTESIAN_POINT('Ctrl Pts',(15.6048088404222,-0.941727856044881,
26.8545665254945));
#41342=CARTESIAN_POINT('Ctrl Pts',(15.6154180433205,-0.973770766529909,
26.6923466536491));
#41343=CARTESIAN_POINT('Ctrl Pts',(15.6195564363349,-0.986269929585368,
26.6290686118502));
#41344=CARTESIAN_POINT('Ctrl Pts',(15.6236948293494,-0.992467126962446,
26.5645457575642));
#41345=CARTESIAN_POINT('Ctrl Pts',(15.6278332223638,-0.992430455435604,
26.5000159512924));
#41346=CARTESIAN_POINT('Origin',(18.,0.,26.5));
#41347=CARTESIAN_POINT('',(16.1721667776362,-0.992590313145785,26.499881711609));
#41348=CARTESIAN_POINT('',(16.0278332223638,-0.992581467290118,26.4999926332401));
#41349=CARTESIAN_POINT('',(18.,-0.9925,26.5));
#41350=CARTESIAN_POINT('Ctrl Pts',(16.1721667776362,-0.992590313145785,
26.499881711609));
#41351=CARTESIAN_POINT('Ctrl Pts',(16.1628583664504,-0.992388437590192,
26.645171964642));
#41352=CARTESIAN_POINT('Ctrl Pts',(16.1535499552646,-0.960027564764405,
26.7907481822402));
#41353=CARTESIAN_POINT('Ctrl Pts',(16.1442415440789,-0.898492852461372,
26.9218815949269));
#41354=CARTESIAN_POINT('Ctrl Pts',(16.1336560085783,-0.828515509540174,
27.0710066569378));
#41355=CARTESIAN_POINT('Ctrl Pts',(16.1230704730778,-0.720809788480869,
27.2014539029726));
#41356=CARTESIAN_POINT('Ctrl Pts',(16.1124849375773,-0.587682335814658,
27.2994478487736));
#41357=CARTESIAN_POINT('Ctrl Pts',(16.1018994020768,-0.454554883148454,
27.3974417945746));
#41358=CARTESIAN_POINT('Ctrl Pts',(16.0913138665762,-0.296005698875348,
27.4629824401418));
#41359=CARTESIAN_POINT('Ctrl Pts',(16.0807283310757,-0.132664255717563,
27.4846930519805));
#41360=CARTESIAN_POINT('Ctrl Pts',(16.0595572600746,0.194018630598016,27.5281142756581));
#41361=CARTESIAN_POINT('Ctrl Pts',(16.0383861890736,0.539870552452309,27.3962153644219));
#41362=CARTESIAN_POINT('Ctrl Pts',(16.0172151180725,0.754676553619223,27.1462843884709));
#41363=CARTESIAN_POINT('Ctrl Pts',(16.006629582572,0.862079554202677,27.0213189004954));
#41364=CARTESIAN_POINT('Ctrl Pts',(15.9960440470714,0.936721074614288,26.8668453963413));
#41365=CARTESIAN_POINT('Ctrl Pts',(15.9854585115709,0.970786327779025,26.7050885090262));
#41366=CARTESIAN_POINT('Ctrl Pts',(15.9748729760704,1.00485158094376,26.5433316217111));
#41367=CARTESIAN_POINT('Ctrl Pts',(15.9642874405698,0.998340566861622,26.3742913512351));
#41368=CARTESIAN_POINT('Ctrl Pts',(15.9537019050693,0.951245016724583,26.2164397696804));
#41369=CARTESIAN_POINT('Ctrl Pts',(15.9431163695688,0.904149466587543,26.0585881881256));
#41370=CARTESIAN_POINT('Ctrl Pts',(15.9325308340682,0.816469380395605,25.9119252954921));
#41371=CARTESIAN_POINT('Ctrl Pts',(15.9219452985677,0.699353476675405,25.7955345380996));
#41372=CARTESIAN_POINT('Ctrl Pts',(15.9113597630672,0.582237572955209,25.6791437807071));
#41373=CARTESIAN_POINT('Ctrl Pts',(15.9007742275666,0.435685851706754,25.5930251585557));
#41374=CARTESIAN_POINT('Ctrl Pts',(15.8901886920661,0.277288843390337,25.5470111858464));
#41375=CARTESIAN_POINT('Ctrl Pts',(15.8796031565656,0.118891835073919,25.5009972131371));
#41376=CARTESIAN_POINT('Ctrl Pts',(15.869017621065,-0.0513504603104619,
25.4950878898698));
#41377=CARTESIAN_POINT('Ctrl Pts',(15.8584320855645,-0.212515773811046,
25.5303738658292));
#41378=CARTESIAN_POINT('Ctrl Pts',(15.847846550064,-0.373681087311639,25.5656598417886));
#41379=CARTESIAN_POINT('Ctrl Pts',(15.8372610145634,-0.525769418928423,
25.6421411169746));
#41380=CARTESIAN_POINT('Ctrl Pts',(15.8266754790629,-0.650406542850507,
25.7502658438782));
#41381=CARTESIAN_POINT('Ctrl Pts',(15.8160899435624,-0.775043666772584,
25.8583905707819));
#41382=CARTESIAN_POINT('Ctrl Pts',(15.8055044080619,-0.872229582999959,
25.9981587494031));
#41383=CARTESIAN_POINT('Ctrl Pts',(15.7949188725613,-0.929914181101119,
26.1527286220079));
#41384=CARTESIAN_POINT('Ctrl Pts',(15.7873348409196,-0.971242446186617,
26.263470568377));
#41385=CARTESIAN_POINT('Ctrl Pts',(15.7797508092779,-0.992294528632976,
26.38181028274));
#41386=CARTESIAN_POINT('Ctrl Pts',(15.7721667776362,-0.992381283892664,
26.5000738717641));
#41387=CARTESIAN_POINT('Ctrl Pts',(15.6278332223638,-0.992430455435604,
26.5000159512924));
#41388=CARTESIAN_POINT('Ctrl Pts',(15.6343040322476,-0.992373115671711,
26.3991168567002));
#41389=CARTESIAN_POINT('Ctrl Pts',(15.6407748421315,-0.977074845476574,
26.2982007654828));
#41390=CARTESIAN_POINT('Ctrl Pts',(15.6472456520153,-0.946795964687865,
26.2019997614615));
#41391=CARTESIAN_POINT('Ctrl Pts',(15.6578548549136,-0.897152288612132,
26.0442736052299));
#41392=CARTESIAN_POINT('Ctrl Pts',(15.6684640578118,-0.807238972712001,
25.8992221568774));
#41393=CARTESIAN_POINT('Ctrl Pts',(15.6790732607101,-0.688060686272364,
25.7845985512143));
#41394=CARTESIAN_POINT('Ctrl Pts',(15.6896824636084,-0.568882399832727,
25.6699749455512));
#41395=CARTESIAN_POINT('Ctrl Pts',(15.7002916665066,-0.42043914285358,25.5857791825775));
#41396=CARTESIAN_POINT('Ctrl Pts',(15.7109008694049,-0.260899180338543,
25.5423161489213));
#41397=CARTESIAN_POINT('Ctrl Pts',(15.7215100723032,-0.101359217823505,
25.4988531152651));
#41398=CARTESIAN_POINT('Ctrl Pts',(15.7321192752015,0.0692774502274137,
25.4961228109265));
#41399=CARTESIAN_POINT('Ctrl Pts',(15.7427284780997,0.230126263157377,25.5344594032753));
#41400=CARTESIAN_POINT('Ctrl Pts',(15.753337680998,0.390975076087336,25.5727959956241));
#41401=CARTESIAN_POINT('Ctrl Pts',(15.7639468838963,0.542036033896329,25.6521994846604));
#41402=CARTESIAN_POINT('Ctrl Pts',(15.7745560867945,0.664820485977887,25.7629515196797));
#41403=CARTESIAN_POINT('Ctrl Pts',(15.7851652896928,0.787604938059444,25.8737035546991));
#41404=CARTESIAN_POINT('Ctrl Pts',(15.7957744925911,0.882112884413569,26.0158041357016));
#41405=CARTESIAN_POINT('Ctrl Pts',(15.8063836954894,0.936777309809986,26.1718612903917));
#41406=CARTESIAN_POINT('Ctrl Pts',(15.8169928983876,0.991441735206403,26.3279184450818));
#41407=CARTESIAN_POINT('Ctrl Pts',(15.8276021012859,1.00626263964511,26.4979321734596));
#41408=CARTESIAN_POINT('Ctrl Pts',(15.8382113041842,0.979426063200181,26.6610941576918));
#41409=CARTESIAN_POINT('Ctrl Pts',(15.8488205070824,0.952589486755249,26.8242561419241));
#41410=CARTESIAN_POINT('Ctrl Pts',(15.8594297099807,0.884095429426674,26.9805663820109));
#41411=CARTESIAN_POINT('Ctrl Pts',(15.870038912879,0.782327014907929,27.1108937572635));
#41412=CARTESIAN_POINT('Ctrl Pts',(15.8806481157773,0.680558600389184,27.2412211325161));
#41413=CARTESIAN_POINT('Ctrl Pts',(15.8912573186755,0.545515828680267,27.3455656429346));
#41414=CARTESIAN_POINT('Ctrl Pts',(15.9018665215738,0.393726852781588,27.4111563566792));
#41415=CARTESIAN_POINT('Ctrl Pts',(15.9124757244721,0.241937876882906,27.4767470704238));
#41416=CARTESIAN_POINT('Ctrl Pts',(15.9230849273704,0.0734026967944721,
27.5035839874945));
#41417=CARTESIAN_POINT('Ctrl Pts',(15.9336941302686,-0.0912513321117865,
27.4883824843177));
#41418=CARTESIAN_POINT('Ctrl Pts',(15.9443033331669,-0.25590536101804,27.4731809811409));
#41419=CARTESIAN_POINT('Ctrl Pts',(15.9549125360652,-0.416678238742111,
27.4159410577166));
#41420=CARTESIAN_POINT('Ctrl Pts',(15.9655217389634,-0.553892653512971,
27.3236684219409));
#41421=CARTESIAN_POINT('Ctrl Pts',(15.9761309418617,-0.691107068283828,
27.2313957861652));
#41422=CARTESIAN_POINT('Ctrl Pts',(15.98674014476,-0.804763020101481,27.1040904380383));
#41423=CARTESIAN_POINT('Ctrl Pts',(15.9973493476583,-0.880949931322436,
26.9573335319231));
#41424=CARTESIAN_POINT('Ctrl Pts',(16.0075106392268,-0.953920297338052,
26.8167725748909));
#41425=CARTESIAN_POINT('Ctrl Pts',(16.0176719307953,-0.992518656563027,
26.6583678441027));
#41426=CARTESIAN_POINT('Ctrl Pts',(16.0278332223638,-0.992581467290118,
26.4999926332401));
#41427=CARTESIAN_POINT('Origin',(18.,0.,26.5));
#41428=CARTESIAN_POINT('',(16.5721667776362,-0.992268890272332,26.499572269901));
#41429=CARTESIAN_POINT('',(16.4278332223638,-0.992414999655005,26.4999960454856));
#41430=CARTESIAN_POINT('',(18.,-0.9925,26.5));
#41431=CARTESIAN_POINT('Ctrl Pts',(16.5721667776362,-0.992268890272332,
26.499572269901));
#41432=CARTESIAN_POINT('Ctrl Pts',(16.567136994624,-0.992197798349475,26.5777683735014));
#41433=CARTESIAN_POINT('Ctrl Pts',(16.5621072116118,-0.982958907028698,
26.6560429188629));
#41434=CARTESIAN_POINT('Ctrl Pts',(16.5570774285996,-0.964609050907775,
26.7324150805005));
#41435=CARTESIAN_POINT('Ctrl Pts',(16.5464918930991,-0.925990475727351,
26.8931457176487));
#41436=CARTESIAN_POINT('Ctrl Pts',(16.5359063575986,-0.847017441008614,
27.0454502804246));
#41437=CARTESIAN_POINT('Ctrl Pts',(16.525320822098,-0.736129089314115,27.1673336311242));
#41438=CARTESIAN_POINT('Ctrl Pts',(16.504149751097,-0.514352385925116,27.4111003325234));
#41439=CARTESIAN_POINT('Ctrl Pts',(16.4829786800959,-0.164914414633087,
27.5331821856175));
#41440=CARTESIAN_POINT('Ctrl Pts',(16.4618076090948,0.160412328171246,27.4805549940388));
#41441=CARTESIAN_POINT('Ctrl Pts',(16.4512220735943,0.323075699573415,27.4542413982495));
#41442=CARTESIAN_POINT('Ctrl Pts',(16.4406365380938,0.479711263853668,27.384250541292));
#41443=CARTESIAN_POINT('Ctrl Pts',(16.4300510025932,0.610018972578666,27.2825370558838));
#41444=CARTESIAN_POINT('Ctrl Pts',(16.4194654670927,0.74032668130366,27.1808235704756));
#41445=CARTESIAN_POINT('Ctrl Pts',(16.4088799315922,0.844306534473414,27.0473874566168));
#41446=CARTESIAN_POINT('Ctrl Pts',(16.3982943960917,0.910045716302035,26.896346162215));
#41447=CARTESIAN_POINT('Ctrl Pts',(16.3877088605911,0.97578489813066,26.7453048678133));
#41448=CARTESIAN_POINT('Ctrl Pts',(16.3771233250906,1.00328340861815,26.5766583928687));
#41449=CARTESIAN_POINT('Ctrl Pts',(16.3665377895901,0.98876440761581,26.4121830393336));
#41450=CARTESIAN_POINT('Ctrl Pts',(16.3559522540895,0.974245406613472,26.2477076857986));
#41451=CARTESIAN_POINT('Ctrl Pts',(16.345366718589,0.917708894121311,26.087403453673));
#41452=CARTESIAN_POINT('Ctrl Pts',(16.3347811830884,0.826265950081132,25.9501260487101));
#41453=CARTESIAN_POINT('Ctrl Pts',(16.3241956475879,0.734823006040954,25.8128486437472));
#41454=CARTESIAN_POINT('Ctrl Pts',(16.3136101120874,0.608473630452758,25.6985980659469));
#41455=CARTESIAN_POINT('Ctrl Pts',(16.3030245765869,0.462510895873329,25.6216939796495));
#41456=CARTESIAN_POINT('Ctrl Pts',(16.2924390410863,0.316548161293896,25.544789893352));
#41457=CARTESIAN_POINT('Ctrl Pts',(16.2818535055858,0.150972067723229,25.5052322985575));
#41458=CARTESIAN_POINT('Ctrl Pts',(16.2712679700853,-0.0140126065616156,
25.5075617789023));
#41459=CARTESIAN_POINT('Ctrl Pts',(16.2606824345847,-0.178997280846465,
25.509891259247));
#41460=CARTESIAN_POINT('Ctrl Pts',(16.2500968990842,-0.343390535845491,
25.5541078147311));
#41461=CARTESIAN_POINT('Ctrl Pts',(16.2395113635837,-0.487123842434778,
25.6351022278228));
#41462=CARTESIAN_POINT('Ctrl Pts',(16.2289258280831,-0.630857149024054,
25.7160966409144));
#41463=CARTESIAN_POINT('Ctrl Pts',(16.2183402925826,-0.753930507203593,
25.8338689116136));
#41464=CARTESIAN_POINT('Ctrl Pts',(16.2077547570821,-0.841461229554299,
25.9736733127347));
#41465=CARTESIAN_POINT('Ctrl Pts',(16.1971692215815,-0.928991951905009,
26.1134777138559));
#41466=CARTESIAN_POINT('Ctrl Pts',(16.186583686081,-0.980980038426882,26.2753142453991));
#41467=CARTESIAN_POINT('Ctrl Pts',(16.1759981505805,-0.99084959929627,26.4401339501642));
#41468=CARTESIAN_POINT('Ctrl Pts',(16.1747210262657,-0.992040342661269,
26.4600191276779));
#41469=CARTESIAN_POINT('Ctrl Pts',(16.173443901951,-0.992618010695394,26.4799477281244));
#41470=CARTESIAN_POINT('Ctrl Pts',(16.1721667776362,-0.992590313145785,
26.499881711609));
#41471=CARTESIAN_POINT('Ctrl Pts',(16.0278332223638,-0.992581467290118,
26.4999926332401));
#41472=CARTESIAN_POINT('Ctrl Pts',(16.0282811336936,-0.992584235996843,
26.4930114290478));
#41473=CARTESIAN_POINT('Ctrl Pts',(16.0287290450233,-0.992512127810711,
26.4860302822144));
#41474=CARTESIAN_POINT('Ctrl Pts',(16.0291769563531,-0.992364786122702,
26.4790507235948));
#41475=CARTESIAN_POINT('Ctrl Pts',(16.0397861592514,-0.988874859077747,
26.3137332854852));
#41476=CARTESIAN_POINT('Ctrl Pts',(16.0503953621496,-0.943177134363577,
26.1493068733695));
#41477=CARTESIAN_POINT('Ctrl Pts',(16.0610045650479,-0.860864647255521,
26.0058959623481));
#41478=CARTESIAN_POINT('Ctrl Pts',(16.0716137679462,-0.778552160147466,
25.8624850513267));
#41479=CARTESIAN_POINT('Ctrl Pts',(16.0822229708444,-0.659624910645523,
25.7400896413997));
#41480=CARTESIAN_POINT('Ctrl Pts',(16.0928321737427,-0.518638640984628,
25.6536899498435));
#41481=CARTESIAN_POINT('Ctrl Pts',(16.103441376641,-0.377652371323737,25.5672902582873));
#41482=CARTESIAN_POINT('Ctrl Pts',(16.1140505795393,-0.214607081503895,
25.516886285102));
#41483=CARTESIAN_POINT('Ctrl Pts',(16.1246597824375,-0.049458208325129,
25.508647072659));
#41484=CARTESIAN_POINT('Ctrl Pts',(16.1352689853358,0.115690664853637,25.500407860216));
#41485=CARTESIAN_POINT('Ctrl Pts',(16.1458781882341,0.282943121391326,25.5343334085154));
#41486=CARTESIAN_POINT('Ctrl Pts',(16.1564873911323,0.431828800998626,25.6062715023306));
#41487=CARTESIAN_POINT('Ctrl Pts',(16.1670965940306,0.580714480605926,25.6782095961459));
#41488=CARTESIAN_POINT('Ctrl Pts',(16.1777057969289,0.711233383282836,25.788160235477));
#41489=CARTESIAN_POINT('Ctrl Pts',(16.1883149998272,0.807411041343378,25.9226663432338));
#41490=CARTESIAN_POINT('Ctrl Pts',(16.1989242027255,0.90358869940392,26.0571724509906));
#41491=CARTESIAN_POINT('Ctrl Pts',(16.2095334056237,0.965425112848094,26.2162340271731));
#41492=CARTESIAN_POINT('Ctrl Pts',(16.220142608522,0.985352000238336,26.3803832096043));
#41493=CARTESIAN_POINT('Ctrl Pts',(16.2307518114202,1.00527888762858,26.5445323920355));
#41494=CARTESIAN_POINT('Ctrl Pts',(16.2413610143185,0.983296248964886,26.7137691807154));
#41495=CARTESIAN_POINT('Ctrl Pts',(16.2519702172168,0.922094583046927,26.8673803490033));
#41496=CARTESIAN_POINT('Ctrl Pts',(16.2625794201151,0.860892917128968,27.0209915172911));
#41497=CARTESIAN_POINT('Ctrl Pts',(16.2731886230133,0.760472223956742,27.158977065187));
#41498=CARTESIAN_POINT('Ctrl Pts',(16.2837978259116,0.633123191585252,27.264448667469));
#41499=CARTESIAN_POINT('Ctrl Pts',(16.2944070288099,0.505774159213761,27.369920269751));
#41500=CARTESIAN_POINT('Ctrl Pts',(16.3050162317082,0.351496787643007,27.4428779264193));
#41501=CARTESIAN_POINT('Ctrl Pts',(16.3156254346064,0.189173390746985,27.4743922049932));
#41502=CARTESIAN_POINT('Ctrl Pts',(16.3262346375047,0.0268499938509623,
27.5059064835671));
#41503=CARTESIAN_POINT('Ctrl Pts',(16.336843840403,-0.143519428370328,27.4959773840466));
#41504=CARTESIAN_POINT('Ctrl Pts',(16.3474530433012,-0.301083024007819,
27.4458201486396));
#41505=CARTESIAN_POINT('Ctrl Pts',(16.3580622461995,-0.458646619645319,
27.3956629132325));
#41506=CARTESIAN_POINT('Ctrl Pts',(16.3686714490978,-0.603404388699017,
27.3052775419388));
#41507=CARTESIAN_POINT('Ctrl Pts',(16.3792806519961,-0.717639140351219,
27.1857264798403));
#41508=CARTESIAN_POINT('Ctrl Pts',(16.3898898548944,-0.831873892003415,
27.0661754177419));
#41509=CARTESIAN_POINT('Ctrl Pts',(16.4004990577926,-0.915585626254117,
26.9174586648388));
#41510=CARTESIAN_POINT('Ctrl Pts',(16.4111082606909,-0.95852869771175,26.7577779598439));
#41511=CARTESIAN_POINT('Ctrl Pts',(16.4166832479152,-0.981094679062509,
26.6738679904662));
#41512=CARTESIAN_POINT('Ctrl Pts',(16.4222582351395,-0.992402985346778,
26.5869304847006));
#41513=CARTESIAN_POINT('Ctrl Pts',(16.4278332223638,-0.992414999655005,
26.4999960454856));
#41514=CARTESIAN_POINT('Origin',(18.,0.,26.5));
#41515=CARTESIAN_POINT('',(16.9721667776362,-0.993608664717065,26.5006377171609));
#41516=CARTESIAN_POINT('',(16.8278332223638,-0.992566518425997,26.500015300021));
#41517=CARTESIAN_POINT('',(18.,-0.9925,26.5));
#41518=CARTESIAN_POINT('Ctrl Pts',(16.9721667776362,-0.993608664717065,
26.5006377171609));
#41519=CARTESIAN_POINT('Ctrl Pts',(16.9714156227976,-0.99360792305922,26.5123412234469));
#41520=CARTESIAN_POINT('Ctrl Pts',(16.970664467959,-0.993388337675886,26.5240391525227));
#41521=CARTESIAN_POINT('Ctrl Pts',(16.9699133131204,-0.992947148238254,
26.5357235520371));
#41522=CARTESIAN_POINT('Ctrl Pts',(16.9487422421193,-0.98051235792753,26.8650448038074));
#41523=CARTESIAN_POINT('Ctrl Pts',(16.9275711711183,-0.792040380383265,
27.1836184818102));
#41524=CARTESIAN_POINT('Ctrl Pts',(16.9064001001172,-0.509390844161436,
27.3530774755247));
#41525=CARTESIAN_POINT('Ctrl Pts',(16.8958145646167,-0.36806607605052,27.4378069723819));
#41526=CARTESIAN_POINT('Ctrl Pts',(16.8852290291161,-0.203196918270212,
27.4852577981671));
#41527=CARTESIAN_POINT('Ctrl Pts',(16.8746434936156,-0.0380092888994282,
27.4914850905056));
#41528=CARTESIAN_POINT('Ctrl Pts',(16.8640579581151,0.127178340471351,27.4977123828441));
#41529=CARTESIAN_POINT('Ctrl Pts',(16.8534724226145,0.292684441432607,27.462716141736));
#41530=CARTESIAN_POINT('Ctrl Pts',(16.842886887114,0.44030145421419,27.3896112159135));
#41531=CARTESIAN_POINT('Ctrl Pts',(16.8323013516135,0.587918466995774,27.316506290091));
#41532=CARTESIAN_POINT('Ctrl Pts',(16.8217158161129,0.717646391597684,27.205292679554));
#41533=CARTESIAN_POINT('Ctrl Pts',(16.8111302806124,0.812561361623588,27.0701849752009));
#41534=CARTESIAN_POINT('Ctrl Pts',(16.8005447451119,0.907476331649495,26.9350772708479));
#41535=CARTESIAN_POINT('Ctrl Pts',(16.7899592096113,0.967578347099393,26.7760754726787));
#41536=CARTESIAN_POINT('Ctrl Pts',(16.7793736741108,0.986150395205684,26.6121792342922));
#41537=CARTESIAN_POINT('Ctrl Pts',(16.7687881386103,1.00472244331198,26.4482829959057));
#41538=CARTESIAN_POINT('Ctrl Pts',(16.7582026031097,0.981764524074659,26.279492317302));
#41539=CARTESIAN_POINT('Ctrl Pts',(16.7476170676092,0.919738931278878,26.1266126776718));
#41540=CARTESIAN_POINT('Ctrl Pts',(16.7370315321087,0.857713338483099,25.9737330380415));
#41541=CARTESIAN_POINT('Ctrl Pts',(16.7264459966081,0.756620072128858,25.8367644373847));
#41542=CARTESIAN_POINT('Ctrl Pts',(16.7158604611076,0.628979934428365,25.7322017075267));
#41543=CARTESIAN_POINT('Ctrl Pts',(16.7052749256071,0.501339796727873,25.6276389776688));
#41544=CARTESIAN_POINT('Ctrl Pts',(16.6946893901066,0.347152787681117,25.5554821186096));
#41545=CARTESIAN_POINT('Ctrl Pts',(16.684103854606,0.185055486963601,25.5247604084482));
#41546=CARTESIAN_POINT('Ctrl Pts',(16.6735183191055,0.0229581862460808,
25.4940386982867));
#41547=CARTESIAN_POINT('Ctrl Pts',(16.662932783605,-0.14704940614221,25.504752137023));
#41548=CARTESIAN_POINT('Ctrl Pts',(16.6523472481044,-0.304084154022982,
25.5552198087159));
#41549=CARTESIAN_POINT('Ctrl Pts',(16.6417617126039,-0.461118901903754,
25.6056874804089));
#41550=CARTESIAN_POINT('Ctrl Pts',(16.6311761771033,-0.605180805276994,
25.6959093850586));
#41551=CARTESIAN_POINT('Ctrl Pts',(16.6205906416028,-0.718963948417315,
25.8155602924839));
#41552=CARTESIAN_POINT('Ctrl Pts',(16.6100051061023,-0.832747091557636,
25.9352111999092));
#41553=CARTESIAN_POINT('Ctrl Pts',(16.5994195706018,-0.916251474465024,
26.0842911101102));
#41554=CARTESIAN_POINT('Ctrl Pts',(16.5888340351012,-0.958871608097665,
26.243409420971));
#41555=CARTESIAN_POINT('Ctrl Pts',(16.5832782826129,-0.98124052022978,26.3269216770548));
#41556=CARTESIAN_POINT('Ctrl Pts',(16.5777225301246,-0.992347416349173,
26.4131991209793));
#41557=CARTESIAN_POINT('Ctrl Pts',(16.5721667776362,-0.992268890272332,
26.499572269901));
#41558=CARTESIAN_POINT('Ctrl Pts',(16.4278332223638,-0.992414999655005,
26.4999960454856));
#41559=CARTESIAN_POINT('Ctrl Pts',(16.4328674380378,-0.992425848580097,
26.4214942124059));
#41560=CARTESIAN_POINT('Ctrl Pts',(16.4379016537117,-0.983225591272503,
26.3429948798214));
#41561=CARTESIAN_POINT('Ctrl Pts',(16.4429358693857,-0.964785793511,26.2667295270344));
#41562=CARTESIAN_POINT('Ctrl Pts',(16.453545072284,-0.925925409188051,26.1060064563066));
#41563=CARTESIAN_POINT('Ctrl Pts',(16.4641542751823,-0.846030231877589,
25.9552049719378));
#41564=CARTESIAN_POINT('Ctrl Pts',(16.4747634780805,-0.734878790988267,
25.8327819670648));
#41565=CARTESIAN_POINT('Ctrl Pts',(16.4853726809788,-0.62372735009895,25.7103589621919));
#41566=CARTESIAN_POINT('Ctrl Pts',(16.4959818838771,-0.481319645630766,
25.6163144368148));
#41567=CARTESIAN_POINT('Ctrl Pts',(16.5065910867753,-0.325085239329991,
25.5621586871501));
#41568=CARTESIAN_POINT('Ctrl Pts',(16.5172002896736,-0.168850833029208,
25.5080029374855));
#41569=CARTESIAN_POINT('Ctrl Pts',(16.5278094925719,0.00121027510417573,
25.4937359635333));
#41570=CARTESIAN_POINT('Ctrl Pts',(16.5384186954702,0.164283968334559,25.5211039285672));
#41571=CARTESIAN_POINT('Ctrl Pts',(16.5490278983684,0.327357661564934,25.5484718936012));
#41572=CARTESIAN_POINT('Ctrl Pts',(16.5596371012667,0.483443939892306,25.6174747976213));
#41573=CARTESIAN_POINT('Ctrl Pts',(16.570246304165,0.613439093752594,25.719667238177));
#41574=CARTESIAN_POINT('Ctrl Pts',(16.5808555070633,0.743434247612885,25.8218596787328));
#41575=CARTESIAN_POINT('Ctrl Pts',(16.5914647099615,0.847338277006087,25.9572416558241));
#41576=CARTESIAN_POINT('Ctrl Pts',(16.6020739128598,0.912434161439791,26.1092435004303));
#41577=CARTESIAN_POINT('Ctrl Pts',(16.6126831157581,0.977530045873495,26.2612453450365));
#41578=CARTESIAN_POINT('Ctrl Pts',(16.6232923186563,1.0038177853477,26.4298670571576));
#41579=CARTESIAN_POINT('Ctrl Pts',(16.6339015215546,0.988079971225441,26.5944706905942));
#41580=CARTESIAN_POINT('Ctrl Pts',(16.6445107244529,0.972342157103183,26.7590743240309));
#41581=CARTESIAN_POINT('Ctrl Pts',(16.6551199273512,0.914578789384463,26.9196598787832));
#41582=CARTESIAN_POINT('Ctrl Pts',(16.6657291302494,0.821859641352038,27.0565729699105));
#41583=CARTESIAN_POINT('Ctrl Pts',(16.6763383331477,0.729140493319612,27.1934860610379));
#41584=CARTESIAN_POINT('Ctrl Pts',(16.686947536046,0.601465564973483,27.3067266885402));
#41585=CARTESIAN_POINT('Ctrl Pts',(16.6975567389442,0.454461244333888,27.382435107142));
#41586=CARTESIAN_POINT('Ctrl Pts',(16.7081659418425,0.307456923694284,27.4581435257437));
#41587=CARTESIAN_POINT('Ctrl Pts',(16.7187751447408,0.141123210761213,27.4963197354449));
#41588=CARTESIAN_POINT('Ctrl Pts',(16.7293843476391,-0.0241819810306813,
27.4922912741286));
#41589=CARTESIAN_POINT('Ctrl Pts',(16.7399935505373,-0.189487172822562,
27.4882628128124));
#41590=CARTESIAN_POINT('Ctrl Pts',(16.7506027534356,-0.353763843473277,
27.4420296804787));
#41591=CARTESIAN_POINT('Ctrl Pts',(16.7612119563339,-0.496905845036753,
27.3592504420054));
#41592=CARTESIAN_POINT('Ctrl Pts',(16.7718211592322,-0.640047846600237,
27.2764712035321));
#41593=CARTESIAN_POINT('Ctrl Pts',(16.7824303621304,-0.762055179076489,
27.1571458589192));
#41594=CARTESIAN_POINT('Ctrl Pts',(16.7930395650287,-0.847995122760424,
27.0158788740514));
#41595=CARTESIAN_POINT('Ctrl Pts',(16.803648767927,-0.933935066444353,26.8746118891835));
#41596=CARTESIAN_POINT('Ctrl Pts',(16.8142579708253,-0.983807621335963,
26.7114032640608));
#41597=CARTESIAN_POINT('Ctrl Pts',(16.8248671737235,-0.99150878640109,26.546228426418));
#41598=CARTESIAN_POINT('Ctrl Pts',(16.8258558566036,-0.992226466148543,
26.5308356079597));
#41599=CARTESIAN_POINT('Ctrl Pts',(16.8268445394837,-0.992577905342496,
26.5154257137833));
#41600=CARTESIAN_POINT('Ctrl Pts',(16.8278332223638,-0.992566518425997,
26.500015300021));
#41601=CARTESIAN_POINT('Origin',(18.,0.,26.5));
#41602=CARTESIAN_POINT('',(17.3721667776362,-0.991136349068622,26.5001921337659));
#41603=CARTESIAN_POINT('',(17.2278332223638,-0.99244811917863,26.4999785467739));
#41604=CARTESIAN_POINT('',(18.,-0.9925,26.5));
#41605=CARTESIAN_POINT('Ctrl Pts',(17.3721667776362,-0.991136349068622,
26.5001921337659));
#41606=CARTESIAN_POINT('Ctrl Pts',(17.3651087154707,-0.991892155534025,
26.6100961603842));
#41607=CARTESIAN_POINT('Ctrl Pts',(17.3580506533051,-0.974948391853953,
26.7199509551589));
#41608=CARTESIAN_POINT('Ctrl Pts',(17.3509925911395,-0.939319387565507,
26.8238816182409));
#41609=CARTESIAN_POINT('Ctrl Pts',(17.340407055639,-0.885883744623132,26.9797546748733));
#41610=CARTESIAN_POINT('Ctrl Pts',(17.3298215201385,-0.790418681165517,
27.1223023573604));
#41611=CARTESIAN_POINT('Ctrl Pts',(17.319235984638,-0.668138790300684,27.2335379649631));
#41612=CARTESIAN_POINT('Ctrl Pts',(17.3086504491374,-0.545858899435857,
27.3447735725658));
#41613=CARTESIAN_POINT('Ctrl Pts',(17.2980649136369,-0.396764181163814,
27.4246971052841));
#41614=CARTESIAN_POINT('Ctrl Pts',(17.2874793781363,-0.236782908219976,
27.4639540139289));
#41615=CARTESIAN_POINT('Ctrl Pts',(17.2768938426358,-0.0768016352761392,
27.5032109225737));
#41616=CARTESIAN_POINT('Ctrl Pts',(17.2663083071353,0.0940661923394922,
27.5018012071451));
#41617=CARTESIAN_POINT('Ctrl Pts',(17.2557227716348,0.253719211720844,27.4596840281348));
#41618=CARTESIAN_POINT('Ctrl Pts',(17.2451372361342,0.413372231102205,27.4175668491245));
#41619=CARTESIAN_POINT('Ctrl Pts',(17.2345517006337,0.561810442249285,27.3347422065326));
#41620=CARTESIAN_POINT('Ctrl Pts',(17.2239661651331,0.68165181448249,27.2214066719458));
#41621=CARTESIAN_POINT('Ctrl Pts',(17.2133806296326,0.801493186715687,27.1080711373589));
#41622=CARTESIAN_POINT('Ctrl Pts',(17.2027950941321,0.892737720035012,26.9642247107773));
#41623=CARTESIAN_POINT('Ctrl Pts',(17.1922095586316,0.943857422910035,26.807361284942));
#41624=CARTESIAN_POINT('Ctrl Pts',(17.181624023131,0.994977125785058,26.6504978591067));
#41625=CARTESIAN_POINT('Ctrl Pts',(17.1710384876305,1.00597199821578,26.4806174340177));
#41626=CARTESIAN_POINT('Ctrl Pts',(17.16045295213,0.975782759799013,26.3184015929024));
#41627=CARTESIAN_POINT('Ctrl Pts',(17.1498674166294,0.945593521382245,26.156185751787));
#41628=CARTESIAN_POINT('Ctrl Pts',(17.1392818811289,0.874220172117985,26.0016344946453));
#41629=CARTESIAN_POINT('Ctrl Pts',(17.1286963456284,0.770091285950915,25.8736636642194));
#41630=CARTESIAN_POINT('Ctrl Pts',(17.1181108101278,0.66596239978385,25.7456928337934));
#41631=CARTESIAN_POINT('Ctrl Pts',(17.1075252746273,0.529077976713979,25.6443024300833));
#41632=CARTESIAN_POINT('Ctrl Pts',(17.0969397391268,0.376487631167103,25.5816678998663));
#41633=CARTESIAN_POINT('Ctrl Pts',(17.0863542036262,0.223897285620227,25.5190333696494));
#41634=CARTESIAN_POINT('Ctrl Pts',(17.0757686681257,0.0556010175963462,
25.4951547129257));
#41635=CARTESIAN_POINT('Ctrl Pts',(17.0651831326252,-0.108514671340715,
25.5132926277484));
#41636=CARTESIAN_POINT('Ctrl Pts',(17.0545975971246,-0.272630360277776,
25.5314305425711));
#41637=CARTESIAN_POINT('Ctrl Pts',(17.0440120616241,-0.432565470128018,
25.5915850289401));
#41638=CARTESIAN_POINT('Ctrl Pts',(17.0334265261236,-0.567713051738021,
25.6857670008228));
#41639=CARTESIAN_POINT('Ctrl Pts',(17.022840990623,-0.702860633348025,25.7799489727055));
#41640=CARTESIAN_POINT('Ctrl Pts',(17.0122554551225,-0.813220686717791,
25.9081584301017));
#41641=CARTESIAN_POINT('Ctrl Pts',(17.001669919622,-0.887296664229188,26.0559369184634));
#41642=CARTESIAN_POINT('Ctrl Pts',(16.9918355389601,-0.956116173711191,
26.1932289721453));
#41643=CARTESIAN_POINT('Ctrl Pts',(16.9820011582981,-0.993618374759788,
26.347411338285));
#41644=CARTESIAN_POINT('Ctrl Pts',(16.9721667776362,-0.993608664717065,
26.5006377171609));
#41645=CARTESIAN_POINT('Ctrl Pts',(16.8278332223638,-0.992566518425997,
26.500015300021));
#41646=CARTESIAN_POINT('Ctrl Pts',(16.837453742382,-0.992455716408151,26.3500620672179));
#41647=CARTESIAN_POINT('Ctrl Pts',(16.8470742624002,-0.957990575121126,
26.2000596372117));
#41648=CARTESIAN_POINT('Ctrl Pts',(16.8566947824183,-0.892316991382856,
26.065262000966));
#41649=CARTESIAN_POINT('Ctrl Pts',(16.8673039853166,-0.819894256060864,
25.9166114633197));
#41650=CARTESIAN_POINT('Ctrl Pts',(16.8779131882149,-0.709519010178247,
25.7864514381899));
#41651=CARTESIAN_POINT('Ctrl Pts',(16.8885223911132,-0.57470029925367,25.690712469537));
#41652=CARTESIAN_POINT('Ctrl Pts',(16.8991315940114,-0.439881588329094,
25.594973500884));
#41653=CARTESIAN_POINT('Ctrl Pts',(16.9097407969097,-0.280619412362559,
25.5336555887078));
#41654=CARTESIAN_POINT('Ctrl Pts',(16.920349999808,-0.11640618535689,25.5142635540274));
#41655=CARTESIAN_POINT('Ctrl Pts',(16.9309592027062,0.0478070416487797,
25.4948715193471));
#41656=CARTESIAN_POINT('Ctrl Pts',(16.9415684056045,0.216971319693583,25.5174053621625));
#41657=CARTESIAN_POINT('Ctrl Pts',(16.9521776085028,0.370382296894979,25.5791071207387));
#41658=CARTESIAN_POINT('Ctrl Pts',(16.9627868114011,0.523793274096375,25.6408088793148));
#41659=CARTESIAN_POINT('Ctrl Pts',(16.9733960142993,0.661450950454363,25.7416785536516));
#41660=CARTESIAN_POINT('Ctrl Pts',(16.9840052171976,0.766507129524873,25.8693705039312));
#41661=CARTESIAN_POINT('Ctrl Pts',(16.9946144200959,0.871563308595388,25.9970624542109));
#41662=CARTESIAN_POINT('Ctrl Pts',(17.0052236229942,0.944017990378417,26.1515766804334));
#41663=CARTESIAN_POINT('Ctrl Pts',(17.0158328258924,0.975003302622344,26.314001879739));
#41664=CARTESIAN_POINT('Ctrl Pts',(17.0264420287907,1.00598861486627,26.4764270790447));
#41665=CARTESIAN_POINT('Ctrl Pts',(17.037051231689,0.995504557571091,26.6467632514335));
#41666=CARTESIAN_POINT('Ctrl Pts',(17.0476604345872,0.94483429507576,26.8041626142725));
#41667=CARTESIAN_POINT('Ctrl Pts',(17.0582696374855,0.894164032580429,26.9615619771116));
#41668=CARTESIAN_POINT('Ctrl Pts',(17.0688788403838,0.803307564884947,27.106024530401));
#41669=CARTESIAN_POINT('Ctrl Pts',(17.0794880432821,0.683384995972857,27.2198692158136));
#41670=CARTESIAN_POINT('Ctrl Pts',(17.0900972461803,0.563462427060767,27.3337139012263));
#41671=CARTESIAN_POINT('Ctrl Pts',(17.1007064490786,0.414473756932069,27.4169407187623));
#41672=CARTESIAN_POINT('Ctrl Pts',(17.1113156519769,0.254654003887244,27.4593633721055));
#41673=CARTESIAN_POINT('Ctrl Pts',(17.1219248548751,0.0948342508424191,
27.5017860254488));
#41674=CARTESIAN_POINT('Ctrl Pts',(17.1325340577734,-0.0758165851185327,
27.5034045145994));
#41675=CARTESIAN_POINT('Ctrl Pts',(17.1431432606717,-0.236412207597704,
27.4640207510499));
#41676=CARTESIAN_POINT('Ctrl Pts',(17.15375246357,-0.397007830076871,27.4246369875004));
#41677=CARTESIAN_POINT('Ctrl Pts',(17.1643616664682,-0.547548239074259,
27.3442509712509));
#41678=CARTESIAN_POINT('Ctrl Pts',(17.1749708693665,-0.669608498200657,
27.232701303453));
#41679=CARTESIAN_POINT('Ctrl Pts',(17.1855800722648,-0.791668757327062,
27.1211516356551));
#41680=CARTESIAN_POINT('Ctrl Pts',(17.196189275163,-0.885248866582474,26.978438316309));
#41681=CARTESIAN_POINT('Ctrl Pts',(17.2067984780613,-0.938895364492047,
26.8220283176548));
#41682=CARTESIAN_POINT('Ctrl Pts',(17.2138100594955,-0.974350128846863,
26.7186575504825));
#41683=CARTESIAN_POINT('Ctrl Pts',(17.2208216409296,-0.992362541423131,
26.6093042966119));
#41684=CARTESIAN_POINT('Ctrl Pts',(17.2278332223638,-0.99244811917863,26.4999785467739));
#41685=CARTESIAN_POINT('Origin',(18.,0.,26.5));
#41686=CARTESIAN_POINT('',(17.7721667776362,-0.992388106880432,26.5001388685385));
#41687=CARTESIAN_POINT('',(17.6278332223638,-0.992500513774779,26.5000263957801));
#41688=CARTESIAN_POINT('',(18.,-0.9925,26.5));
#41689=CARTESIAN_POINT('Ctrl Pts',(17.7721667776362,-0.992388106880432,
26.5001388685385));
#41690=CARTESIAN_POINT('Ctrl Pts',(17.7693873436442,-0.992277927963132,
26.5436557685285));
#41691=CARTESIAN_POINT('Ctrl Pts',(17.7666079096523,-0.989362052989495,
26.5871401972748));
#41692=CARTESIAN_POINT('Ctrl Pts',(17.7638284756603,-0.983640977958964,
26.6301655848495));
#41693=CARTESIAN_POINT('Ctrl Pts',(17.7532429401598,-0.961852137852761,
26.7940287199015));
#41694=CARTESIAN_POINT('Ctrl Pts',(17.7426574046592,-0.899374320287603,
26.9512335362917));
#41695=CARTESIAN_POINT('Ctrl Pts',(17.7320718691587,-0.802363869957874,
27.0843655363258));
#41696=CARTESIAN_POINT('Ctrl Pts',(17.7214863336582,-0.705353419628139,
27.2174975363598));
#41697=CARTESIAN_POINT('Ctrl Pts',(17.7109007981576,-0.573810336533829,
27.3265567200377));
#41698=CARTESIAN_POINT('Ctrl Pts',(17.7003152626571,-0.424601154204597,
27.3972635217341));
#41699=CARTESIAN_POINT('Ctrl Pts',(17.6897297271566,-0.275391971875373,
27.4679703234305));
#41700=CARTESIAN_POINT('Ctrl Pts',(17.679144191656,-0.108516690311227,27.5003247431453));
#41701=CARTESIAN_POINT('Ctrl Pts',(17.6685586561555,0.0561603902068333,
27.4909200220565));
#41702=CARTESIAN_POINT('Ctrl Pts',(17.657973120655,0.220837470724894,27.4815153009676));
#41703=CARTESIAN_POINT('Ctrl Pts',(17.6473875851544,0.383316350196873,27.4303514390751));
#41704=CARTESIAN_POINT('Ctrl Pts',(17.6368020496539,0.523508687926737,27.3433720559961));
#41705=CARTESIAN_POINT('Ctrl Pts',(17.6262165141534,0.663701025656609,27.2563926729171));
#41706=CARTESIAN_POINT('Ctrl Pts',(17.6156309786528,0.781606821644367,27.1335977686517));
#41707=CARTESIAN_POINT('Ctrl Pts',(17.6050454431523,0.863084818137216,26.9901170051206));
#41708=CARTESIAN_POINT('Ctrl Pts',(17.5944599076518,0.944562814630061,26.8466362415895));
#41709=CARTESIAN_POINT('Ctrl Pts',(17.5838743721513,0.989613011628003,26.6824696187928));
#41710=CARTESIAN_POINT('Ctrl Pts',(17.5732888366507,0.992487299462635,26.5175117774126));
#41711=CARTESIAN_POINT('Ctrl Pts',(17.5627033011502,0.995361587297268,26.3525539360324));
#41712=CARTESIAN_POINT('Ctrl Pts',(17.5521177656496,0.956059965968592,26.1868048760686));
#41713=CARTESIAN_POINT('Ctrl Pts',(17.5415322301491,0.879769581345556,26.0405630378266));
#41714=CARTESIAN_POINT('Ctrl Pts',(17.5309466946486,0.803479196722518,25.8943211995846));
#41715=CARTESIAN_POINT('Ctrl Pts',(17.5203611591481,0.690200048805118,25.7675865830643));
#41716=CARTESIAN_POINT('Ctrl Pts',(17.5097756236475,0.553034680142503,25.6756702789943));
#41717=CARTESIAN_POINT('Ctrl Pts',(17.499190088147,0.415869311479896,25.5837539749243));
#41718=CARTESIAN_POINT('Ctrl Pts',(17.4886045526465,0.254817722072074,25.5266559833047));
#41719=CARTESIAN_POINT('Ctrl Pts',(17.4780190171459,0.0907843533403148,
25.5115508634293));
#41720=CARTESIAN_POINT('Ctrl Pts',(17.4674334816454,-0.0732490153914441,
25.4964457435539));
#41721=CARTESIAN_POINT('Ctrl Pts',(17.4568479461449,-0.240264163447142,
25.5233334954228));
#41722=CARTESIAN_POINT('Ctrl Pts',(17.4462624106443,-0.392151958435379,
25.5885702267216));
#41723=CARTESIAN_POINT('Ctrl Pts',(17.4356768751438,-0.544039753423623,
25.6538069580204));
#41724=CARTESIAN_POINT('Ctrl Pts',(17.4250913396433,-0.680800195344407,
25.7573926687492));
#41725=CARTESIAN_POINT('Ctrl Pts',(17.4145058041427,-0.782181555987627,
25.8872910775428));
#41726=CARTESIAN_POINT('Ctrl Pts',(17.4003927953072,-0.917346757449673,
26.0604762121946));
#41727=CARTESIAN_POINT('Ctrl Pts',(17.3862797864717,-0.989625069757963,
26.2804325932095));
#41728=CARTESIAN_POINT('Ctrl Pts',(17.3721667776362,-0.991136349068622,
26.5001921337659));
#41729=CARTESIAN_POINT('Ctrl Pts',(17.2278332223638,-0.99244811917863,26.4999785467739));
#41730=CARTESIAN_POINT('Ctrl Pts',(17.2314308438279,-0.992492028869037,
26.443883831496));
#41731=CARTESIAN_POINT('Ctrl Pts',(17.235028465292,-0.987816366912872,26.3877963571647));
#41732=CARTESIAN_POINT('Ctrl Pts',(17.2386260867561,-0.978355688226005,
26.3325279671566));
#41733=CARTESIAN_POINT('Ctrl Pts',(17.2492352896544,-0.95045662748666,26.1695442932747));
#41734=CARTESIAN_POINT('Ctrl Pts',(17.2598444925527,-0.880945619444235,
26.0136836234732));
#41735=CARTESIAN_POINT('Ctrl Pts',(17.270453695451,-0.778330232769517,25.8840220748992));
#41736=CARTESIAN_POINT('Ctrl Pts',(17.2810628983492,-0.675714846094799,
25.7543605263252));
#41737=CARTESIAN_POINT('Ctrl Pts',(17.2916721012475,-0.539995080787785,
25.6508980989787));
#41738=CARTESIAN_POINT('Ctrl Pts',(17.3022813041458,-0.387781989300544,
25.5862977265485));
#41739=CARTESIAN_POINT('Ctrl Pts',(17.312890507044,-0.235568897813299,25.5216973541183));
#41740=CARTESIAN_POINT('Ctrl Pts',(17.3234997099423,-0.0668624801458348,
25.4959590366045));
#41741=CARTESIAN_POINT('Ctrl Pts',(17.3341089128406,0.0976890273760728,
25.5122330100268));
#41742=CARTESIAN_POINT('Ctrl Pts',(17.3447181157389,0.262240534897985,25.5285069834492));
#41743=CARTESIAN_POINT('Ctrl Pts',(17.3553273186371,0.42263713227433,25.5867932478078));
#41744=CARTESIAN_POINT('Ctrl Pts',(17.3659365215354,0.559247415751573,25.6799578950811));
#41745=CARTESIAN_POINT('Ctrl Pts',(17.3765457244337,0.695857699228807,25.7731225423545));
#41746=CARTESIAN_POINT('Ctrl Pts',(17.387154927332,0.808681668806945,25.9011655725426));
#41747=CARTESIAN_POINT('Ctrl Pts',(17.3977641302302,0.883910849877243,26.0484158024241));
#41748=CARTESIAN_POINT('Ctrl Pts',(17.4083733331285,0.959140030947542,26.1956660323055));
#41749=CARTESIAN_POINT('Ctrl Pts',(17.4189825360268,0.996774423510004,26.3621234618803));
#41750=CARTESIAN_POINT('Ctrl Pts',(17.429591738925,0.992207360123716,26.5274145495491));
#41751=CARTESIAN_POINT('Ctrl Pts',(17.4402009418233,0.987640296737429,26.6927056372179));
#41752=CARTESIAN_POINT('Ctrl Pts',(17.4508101447216,0.940871777402391,26.8568303829806));
#41753=CARTESIAN_POINT('Ctrl Pts',(17.4614193476199,0.857626874806772,26.9997021513987));
#41754=CARTESIAN_POINT('Ctrl Pts',(17.4720285505181,0.774381972211152,27.1425739198167));
#41755=CARTESIAN_POINT('Ctrl Pts',(17.4826377534164,0.654660686354949,27.2641927108899));
#41756=CARTESIAN_POINT('Ctrl Pts',(17.4932469563147,0.513114091336382,27.3496716256727));
#41757=CARTESIAN_POINT('Ctrl Pts',(17.503856159213,0.371567496317814,27.4351505404554));
#41758=CARTESIAN_POINT('Ctrl Pts',(17.5144653621112,0.20819559213688,27.4844895789476));
#41759=CARTESIAN_POINT('Ctrl Pts',(17.5250745650095,0.0429972871920246,
27.4916533116257));
#41760=CARTESIAN_POINT('Ctrl Pts',(17.5356837679078,-0.122201017752836,
27.4988170443038));
#41761=CARTESIAN_POINT('Ctrl Pts',(17.546292970806,-0.289225723461607,27.4638054711678));
#41762=CARTESIAN_POINT('Ctrl Pts',(17.5569021737043,-0.437640946846334,
27.3908975473816));
#41763=CARTESIAN_POINT('Ctrl Pts',(17.5675113766026,-0.586056170231056,
27.3179896235954));
#41764=CARTESIAN_POINT('Ctrl Pts',(17.5781205795009,-0.715861911291723,
27.2071853491589));
#41765=CARTESIAN_POINT('Ctrl Pts',(17.5887297823991,-0.811158521085179,
27.0720579498581));
#41766=CARTESIAN_POINT('Ctrl Pts',(17.5993389852974,-0.906455130878635,
26.9369305505572));
#41767=CARTESIAN_POINT('Ctrl Pts',(17.6099481881957,-0.967242609404881,
26.7774800263921));
#41768=CARTESIAN_POINT('Ctrl Pts',(17.6205573910939,-0.986104595712793,
26.6131998072346));
#41769=CARTESIAN_POINT('Ctrl Pts',(17.6229826681839,-0.990416469441883,
26.5756451430741));
#41770=CARTESIAN_POINT('Ctrl Pts',(17.6254079452739,-0.992537378432218,
26.5378380861361));
#41771=CARTESIAN_POINT('Ctrl Pts',(17.6278332223638,-0.992500513774779,
26.5000263957801));
#41772=CARTESIAN_POINT('Origin',(18.,0.,26.5));
#41773=CARTESIAN_POINT('',(18.1721667776362,-0.993299106214555,26.5003419800918));
#41774=CARTESIAN_POINT('',(18.0278332223638,-0.992167930500117,26.4998747777436));
#41775=CARTESIAN_POINT('',(18.,-0.9925,26.5));
#41776=CARTESIAN_POINT('Ctrl Pts',(18.1721667776362,-0.993299106214555,
26.5003419800918));
#41777=CARTESIAN_POINT('Ctrl Pts',(18.1524949008168,-0.991326401614957,
26.8062082540558));
#41778=CARTESIAN_POINT('Ctrl Pts',(18.1328230239973,-0.841330030363234,
27.1099769695095));
#41779=CARTESIAN_POINT('Ctrl Pts',(18.1131511471779,-0.596827584575755,
27.2943640520012));
#41780=CARTESIAN_POINT('Ctrl Pts',(18.1025656116773,-0.465259593193731,
27.3935836651306));
#41781=CARTESIAN_POINT('Ctrl Pts',(18.0919800761768,-0.306326706074318,
27.4582354903689));
#41782=CARTESIAN_POINT('Ctrl Pts',(18.0813945406763,-0.142734068023168,
27.4819016698871));
#41783=CARTESIAN_POINT('Ctrl Pts',(18.0708090051757,0.020858570027974,27.5055678494052));
#41784=CARTESIAN_POINT('Ctrl Pts',(18.0602234696752,0.189110959010848,27.4882483832032));
#41785=CARTESIAN_POINT('Ctrl Pts',(18.0496379341747,0.343650673209678,27.4311978245028));
#41786=CARTESIAN_POINT('Ctrl Pts',(18.0390523986741,0.498190387408508,27.3741472658025));
#41787=CARTESIAN_POINT('Ctrl Pts',(18.0284668631736,0.639017426823289,27.2773656146038));
#41788=CARTESIAN_POINT('Ctrl Pts',(18.0178813276731,0.747674083450534,27.153028467699));
#41789=CARTESIAN_POINT('Ctrl Pts',(18.0072957921725,0.856330740077779,27.0286913207943));
#41790=CARTESIAN_POINT('Ctrl Pts',(17.996710256672,0.932817013917483,26.8767986781835));
#41791=CARTESIAN_POINT('Ctrl Pts',(17.9861247211715,0.968680791357801,26.7158540046014));
#41792=CARTESIAN_POINT('Ctrl Pts',(17.9755391856709,1.00454456879812,26.5549093310193));
#41793=CARTESIAN_POINT('Ctrl Pts',(17.9649536501704,0.999785849839044,26.3849126264658));
#41794=CARTESIAN_POINT('Ctrl Pts',(17.9543681146699,0.954200819239477,26.2262053483874));
#41795=CARTESIAN_POINT('Ctrl Pts',(17.9437825791693,0.908615788639911,26.067498070309));
#41796=CARTESIAN_POINT('Ctrl Pts',(17.9331970436688,0.822204446399863,25.9200802187056));
#41797=CARTESIAN_POINT('Ctrl Pts',(17.9226115081683,0.706508638419301,25.8028122796583));
#41798=CARTESIAN_POINT('Ctrl Pts',(17.9120259726677,0.590812830438738,25.685544340611));
#41799=CARTESIAN_POINT('Ctrl Pts',(17.9014404371672,0.445832556717666,25.5984263141198));
#41800=CARTESIAN_POINT('Ctrl Pts',(17.8908549016667,0.287669343599446,25.5503946860645));
#41801=CARTESIAN_POINT('Ctrl Pts',(17.8802693661661,0.129506130481227,25.5023630580093));
#41802=CARTESIAN_POINT('Ctrl Pts',(17.8696838306656,-0.0418400220341332,
25.49341782839));
#41803=CARTESIAN_POINT('Ctrl Pts',(17.8590982951651,-0.203087213622878,
25.5273885686025));
#41804=CARTESIAN_POINT('Ctrl Pts',(17.837927224164,-0.525581596800377,25.5953300490274));
#41805=CARTESIAN_POINT('Ctrl Pts',(17.816756153163,-0.807680136271397,25.8349354087794));
#41806=CARTESIAN_POINT('Ctrl Pts',(17.7955850821619,-0.926913165898742,
26.1421658003154));
#41807=CARTESIAN_POINT('Ctrl Pts',(17.7877789806533,-0.970876229099324,
26.2554464001832));
#41808=CARTESIAN_POINT('Ctrl Pts',(17.7799728791448,-0.992697546793389,
26.3779206976304));
#41809=CARTESIAN_POINT('Ctrl Pts',(17.7721667776362,-0.992388106880432,
26.5001388685385));
#41810=CARTESIAN_POINT('Ctrl Pts',(17.6278332223638,-0.992500513774779,
26.5000263957801));
#41811=CARTESIAN_POINT('Ctrl Pts',(17.6360171481721,-0.992376116598608,
26.372433524086));
#41812=CARTESIAN_POINT('Ctrl Pts',(17.6442010739804,-0.96768164208166,26.2447878927147));
#41813=CARTESIAN_POINT('Ctrl Pts',(17.6523849997888,-0.91969241995934,26.1266093718736));
#41814=CARTESIAN_POINT('Ctrl Pts',(17.662994202687,-0.857481763808406,25.9734090698196));
#41815=CARTESIAN_POINT('Ctrl Pts',(17.6736034055853,-0.756123957416963,
25.8361183798614));
#41816=CARTESIAN_POINT('Ctrl Pts',(17.6842126084836,-0.628108302777589,
25.7314620191992));
#41817=CARTESIAN_POINT('Ctrl Pts',(17.6948218113819,-0.500092648138214,
25.6268056585371));
#41818=CARTESIAN_POINT('Ctrl Pts',(17.7054310142801,-0.345419145250907,
25.5547836271711));
#41819=CARTESIAN_POINT('Ctrl Pts',(17.7160402171784,-0.182860175475946,
25.5243591626045));
#41820=CARTESIAN_POINT('Ctrl Pts',(17.7266494200767,-0.0203012057009853,
25.493934698038));
#41821=CARTESIAN_POINT('Ctrl Pts',(17.7372586229749,0.150143230961628,25.5051078002709));
#41822=CARTESIAN_POINT('Ctrl Pts',(17.7478678258732,0.307313306622748,25.5562311193872));
#41823=CARTESIAN_POINT('Ctrl Pts',(17.7584770287715,0.464483382283867,25.6073544385036));
#41824=CARTESIAN_POINT('Ctrl Pts',(17.7690862316698,0.608379096943491,25.6984279745035));
#41825=CARTESIAN_POINT('Ctrl Pts',(17.779695434568,0.721950285213137,25.8188318149112));
#41826=CARTESIAN_POINT('Ctrl Pts',(17.7903046374663,0.835521473482784,25.9392356553189));
#41827=CARTESIAN_POINT('Ctrl Pts',(17.8009138403646,0.918768135362452,26.0889698001345));
#41828=CARTESIAN_POINT('Ctrl Pts',(17.8115230432629,0.960463045171784,26.2487268741978));
#41829=CARTESIAN_POINT('Ctrl Pts',(17.8221322461611,1.00215795498112,26.4084839482611));
#41830=CARTESIAN_POINT('Ctrl Pts',(17.8327414490594,1.00230111272011,26.5782639515722));
#41831=CARTESIAN_POINT('Ctrl Pts',(17.8433506519577,0.962664065091785,26.7390341250452));
#41832=CARTESIAN_POINT('Ctrl Pts',(17.8539598548559,0.923027017463459,26.8998042985182));
#41833=CARTESIAN_POINT('Ctrl Pts',(17.8645690577542,0.843609764467811,27.0515646421531));
#41834=CARTESIAN_POINT('Ctrl Pts',(17.8751782606525,0.73155870107366,27.1728217499988));
#41835=CARTESIAN_POINT('Ctrl Pts',(17.896396666449,0.507456574285351,27.4153359656903));
#41836=CARTESIAN_POINT('Ctrl Pts',(17.9176150722456,0.152819205903019,27.5358372382248));
#41837=CARTESIAN_POINT('Ctrl Pts',(17.9388334780421,-0.170925105187162,
27.4793334710585));
#41838=CARTESIAN_POINT('Ctrl Pts',(17.9600518838387,-0.494669416277325,
27.4228297038923));
#41839=CARTESIAN_POINT('Ctrl Pts',(17.9812702896352,-0.787520670075341,
27.1893208970252));
#41840=CARTESIAN_POINT('Ctrl Pts',(18.0024886954318,-0.916222847840073,
26.8852310131387));
#41841=CARTESIAN_POINT('Ctrl Pts',(18.0109368710758,-0.967466028593146,
26.7641566602738));
#41842=CARTESIAN_POINT('Ctrl Pts',(18.0193850467198,-0.992687320953884,
26.6318933750482));
#41843=CARTESIAN_POINT('Ctrl Pts',(18.0278332223638,-0.992167930500117,
26.4998747777436));
#41844=CARTESIAN_POINT('Origin',(18.,0.,26.5));
#41845=CARTESIAN_POINT('',(18.5721667776362,-0.992013826433795,26.5001094462548));
#41846=CARTESIAN_POINT('',(18.4278332223638,-0.992438477235227,26.500018847878));
#41847=CARTESIAN_POINT('',(18.,-0.9925,26.5));
#41848=CARTESIAN_POINT('Ctrl Pts',(18.5721667776362,-0.992013826433795,
26.5001094462548));
#41849=CARTESIAN_POINT('Ctrl Pts',(18.5673590644909,-0.992691797507188,
26.5748924995848));
#41850=CARTESIAN_POINT('Ctrl Pts',(18.5625513513455,-0.984964120408148,
26.6496733034542));
#41851=CARTESIAN_POINT('Ctrl Pts',(18.5577436382002,-0.968324488518865,
26.7226384852639));
#41852=CARTESIAN_POINT('Ctrl Pts',(18.5471581026997,-0.931687649182769,
26.8832918976037));
#41853=CARTESIAN_POINT('Ctrl Pts',(18.5365725671991,-0.851847049743327,
27.0351434587505));
#41854=CARTESIAN_POINT('Ctrl Pts',(18.5259870316986,-0.742027972960165,
27.1586971060113));
#41855=CARTESIAN_POINT('Ctrl Pts',(18.5154014961981,-0.632208896177009,
27.2822507532721));
#41856=CARTESIAN_POINT('Ctrl Pts',(18.5048159606975,-0.492411342050135,
27.3775064866468));
#41857=CARTESIAN_POINT('Ctrl Pts',(18.494230425197,-0.337483980317443,27.4334763293345));
#41858=CARTESIAN_POINT('Ctrl Pts',(18.4836448896965,-0.182556618584751,
27.4894461720223));
#41859=CARTESIAN_POINT('Ctrl Pts',(18.473059354196,-0.0124994492462404,
27.5061301240229));
#41860=CARTESIAN_POINT('Ctrl Pts',(18.4624738186954,0.150714681188409,27.4811482717958));
#41861=CARTESIAN_POINT('Ctrl Pts',(18.4518882831949,0.313928811623069,27.4561664195688));
#41862=CARTESIAN_POINT('Ctrl Pts',(18.4413027476943,0.470299903153866,27.3895187631141));
#41863=CARTESIAN_POINT('Ctrl Pts',(18.4307172121938,0.601464224911203,27.2895046704257));
#41864=CARTESIAN_POINT('Ctrl Pts',(18.4201316766933,0.732628546668532,27.1894905777374));
#41865=CARTESIAN_POINT('Ctrl Pts',(18.4095461411927,0.838586098652403,27.0561100488154));
#41866=CARTESIAN_POINT('Ctrl Pts',(18.3989606056922,0.906022115696002,26.9055386884288));
#41867=CARTESIAN_POINT('Ctrl Pts',(18.3883750701917,0.973458132739602,26.7549673280422));
#41868=CARTESIAN_POINT('Ctrl Pts',(18.3777895346912,1.00237261484293,26.5872051361909));
#41869=CARTESIAN_POINT('Ctrl Pts',(18.3672039991906,0.989522901577106,26.4227050502185));
#41870=CARTESIAN_POINT('Ctrl Pts',(18.3566184636901,0.976673188311281,26.2582049642461));
#41871=CARTESIAN_POINT('Ctrl Pts',(18.3460329281896,0.922059279676299,26.0969669841524));
#41872=CARTESIAN_POINT('Ctrl Pts',(18.335447392689,0.832060708684393,25.9586934803334));
#41873=CARTESIAN_POINT('Ctrl Pts',(18.3248618571885,0.742062137692492,25.8204199765144));
#41874=CARTESIAN_POINT('Ctrl Pts',(18.314276321688,0.616678904343671,25.7051109489701));
#41875=CARTESIAN_POINT('Ctrl Pts',(18.3036907861874,0.47157520535541,25.6266768609303));
#41876=CARTESIAN_POINT('Ctrl Pts',(18.2931052506869,0.326471506367148,25.5482427728905));
#41877=CARTESIAN_POINT('Ctrl Pts',(18.2825197151864,0.161647341739446,25.5066836243552));
#41878=CARTESIAN_POINT('Ctrl Pts',(18.2719341796858,-0.00346591980345378,
25.5073490266028));
#41879=CARTESIAN_POINT('Ctrl Pts',(18.2613486441853,-0.168579181346363,
25.5080144288503));
#41880=CARTESIAN_POINT('Ctrl Pts',(18.2507631086848,-0.333981539804471,
25.5509043818806));
#41881=CARTESIAN_POINT('Ctrl Pts',(18.2401775731842,-0.478339357414782,
25.6302515771747));
#41882=CARTESIAN_POINT('Ctrl Pts',(18.2295920376837,-0.622697175025086,
25.7095987724687));
#41883=CARTESIAN_POINT('Ctrl Pts',(18.2190065021832,-0.746010451787596,
25.8254032100265));
#41884=CARTESIAN_POINT('Ctrl Pts',(18.2084209666827,-0.835311394982777,
25.9645118802334));
#41885=CARTESIAN_POINT('Ctrl Pts',(18.1978354311821,-0.924612338177959,
26.1036205504403));
#41886=CARTESIAN_POINT('Ctrl Pts',(18.1872498956816,-0.97990094780581,26.2660334532962));
#41887=CARTESIAN_POINT('Ctrl Pts',(18.176664360181,-0.991147287588631,26.4304271181706));
#41888=CARTESIAN_POINT('Ctrl Pts',(18.1751651659994,-0.992740069282665,
26.4537096460938));
#41889=CARTESIAN_POINT('Ctrl Pts',(18.1736659718178,-0.993449446077136,
26.4770319043688));
#41890=CARTESIAN_POINT('Ctrl Pts',(18.1721667776362,-0.993299106214555,
26.5003419800918));
#41891=CARTESIAN_POINT('Ctrl Pts',(18.0278332223638,-0.992167930500117,
26.4998747777436));
#41892=CARTESIAN_POINT('Ctrl Pts',(18.0299942496181,-0.992035071410358,
26.4661046717627));
#41893=CARTESIAN_POINT('Ctrl Pts',(18.0321552768723,-0.990217930806179,
26.432350576365));
#41894=CARTESIAN_POINT('Ctrl Pts',(18.0343163041266,-0.986721215380445,
26.3988038623597));
#41895=CARTESIAN_POINT('Ctrl Pts',(18.0449255070248,-0.969554674164404,
26.2341118647219));
#41896=CARTESIAN_POINT('Ctrl Pts',(18.0555347099231,-0.911907771858281,
26.0744180806445));
#41897=CARTESIAN_POINT('Ctrl Pts',(18.0661439128214,-0.81856096012734,25.9382301187795));
#41898=CARTESIAN_POINT('Ctrl Pts',(18.0767531157197,-0.725214148396399,
25.8020421569145));
#41899=CARTESIAN_POINT('Ctrl Pts',(18.0873623186179,-0.59616742724064,25.6893600172619));
#41900=CARTESIAN_POINT('Ctrl Pts',(18.0979715215162,-0.448524532865736,
25.6145464133485));
#41901=CARTESIAN_POINT('Ctrl Pts',(18.1085807244145,-0.300881638490831,
25.5397328094351));
#41902=CARTESIAN_POINT('Ctrl Pts',(18.1191899273128,-0.134642570896782,
25.502787741261));
#41903=CARTESIAN_POINT('Ctrl Pts',(18.129799130211,0.0305530962615577,25.5079275849267));
#41904=CARTESIAN_POINT('Ctrl Pts',(18.1404083331093,0.195748763419897,25.5130674285925));
#41905=CARTESIAN_POINT('Ctrl Pts',(18.1510175360076,0.359901030142527,25.5602921840981));
#41906=CARTESIAN_POINT('Ctrl Pts',(18.1616267389058,0.502543046533664,25.6439840108097));
#41907=CARTESIAN_POINT('Ctrl Pts',(18.1722359418041,0.645185062924801,25.7276758375213));
#41908=CARTESIAN_POINT('Ctrl Pts',(18.1828451447024,0.766316828984445,25.847834735439));
#41909=CARTESIAN_POINT('Ctrl Pts',(18.1934543476007,0.851312079351126,25.9896683318641));
#41910=CARTESIAN_POINT('Ctrl Pts',(18.2040635504989,0.936307329717812,26.1315019282893));
#41911=CARTESIAN_POINT('Ctrl Pts',(18.2146727533972,0.985166064391531,26.295010223222));
#41912=CARTESIAN_POINT('Ctrl Pts',(18.2252819562955,0.991802795610055,26.4602266028182));
#41913=CARTESIAN_POINT('Ctrl Pts',(18.2358911591938,0.998439526828578,26.6254429824145));
#41914=CARTESIAN_POINT('Ctrl Pts',(18.246500362092,0.962854254591912,26.7923674466743));
#41915=CARTESIAN_POINT('Ctrl Pts',(18.2571095649903,0.889458244410594,26.9405456860461));
#41916=CARTESIAN_POINT('Ctrl Pts',(18.2677187678886,0.816062234229276,27.088723925418));
#41917=CARTESIAN_POINT('Ctrl Pts',(18.2783279707868,0.704855486103307,27.218155939902));
#41918=CARTESIAN_POINT('Ctrl Pts',(18.2889371736851,0.569419202462848,27.3130130479835));
#41919=CARTESIAN_POINT('Ctrl Pts',(18.2995463765834,0.433982918822389,27.4078701560651));
#41920=CARTESIAN_POINT('Ctrl Pts',(18.3101555794817,0.27431709966744,27.4681523577442));
#41921=CARTESIAN_POINT('Ctrl Pts',(18.3207647823799,0.109979244513689,27.4864748370148));
#41922=CARTESIAN_POINT('Ctrl Pts',(18.3313739852782,-0.0543586106400621,
27.5047973162853));
#41923=CARTESIAN_POINT('Ctrl Pts',(18.3419831881765,-0.223368501792614,
27.4811600731473));
#41924=CARTESIAN_POINT('Ctrl Pts',(18.3525923910747,-0.376373278442671,
27.4184596955982));
#41925=CARTESIAN_POINT('Ctrl Pts',(18.363201593973,-0.529378055092728,27.3557593180491));
#41926=CARTESIAN_POINT('Ctrl Pts',(18.3738107968713,-0.666377717240289,
27.2539958060888));
#41927=CARTESIAN_POINT('Ctrl Pts',(18.3844199997696,-0.770600205445519,
27.1256223026464));
#41928=CARTESIAN_POINT('Ctrl Pts',(18.3950292026678,-0.874822693650748,
26.9972487992039));
#41929=CARTESIAN_POINT('Ctrl Pts',(18.4056384055661,-0.946268007913646,
26.8422653042792));
#41930=CARTESIAN_POINT('Ctrl Pts',(18.4162476084644,-0.976194143930204,
26.6796415593889));
#41931=CARTESIAN_POINT('Ctrl Pts',(18.4201094797642,-0.98708760000836,26.6204446546749));
#41932=CARTESIAN_POINT('Ctrl Pts',(18.423971351064,-0.992479585039877,26.5602353837305));
#41933=CARTESIAN_POINT('Ctrl Pts',(18.4278332223638,-0.992438477235227,
26.500018847878));
#41934=CARTESIAN_POINT('Origin',(18.,0.,26.5));
#41935=CARTESIAN_POINT('',(18.9721667776362,-0.992230389713068,26.5005256112294));
#41936=CARTESIAN_POINT('',(18.8278332223638,-0.992574927394752,26.4999883895028));
#41937=CARTESIAN_POINT('',(18.,-0.9925,26.5));
#41938=CARTESIAN_POINT('Ctrl Pts',(18.9721667776362,-0.992230389713068,
26.5005256112294));
#41939=CARTESIAN_POINT('Ctrl Pts',(18.9716376926645,-0.9922196485029,26.5087936640491));
#41940=CARTESIAN_POINT('Ctrl Pts',(18.9711086076927,-0.992106388713782,
26.5170588667457));
#41941=CARTESIAN_POINT('Ctrl Pts',(18.970579522721,-0.991890303783251,26.5253182937189));
#41942=CARTESIAN_POINT('Ctrl Pts',(18.9599939872204,-0.987567038475448,
26.6905667171419));
#41943=CARTESIAN_POINT('Ctrl Pts',(18.9494084517199,-0.942083890356008,
26.8535031758697));
#41944=CARTESIAN_POINT('Ctrl Pts',(18.9388229162194,-0.859710884972681,
26.9961559032424));
#41945=CARTESIAN_POINT('Ctrl Pts',(18.9282373807188,-0.777337879589353,
27.138808630615));
#41946=CARTESIAN_POINT('Ctrl Pts',(18.9176518452183,-0.658075016942137,
27.2611776266325));
#41947=CARTESIAN_POINT('Ctrl Pts',(18.9070663097178,-0.517187564913484,
27.3472802930853));
#41948=CARTESIAN_POINT('Ctrl Pts',(18.8964807742172,-0.376300112884831,
27.433382959538));
#41949=CARTESIAN_POINT('Ctrl Pts',(18.8858952387167,-0.213788071474739,
27.4832192964261));
#41950=CARTESIAN_POINT('Ctrl Pts',(18.8753097032162,-0.0490408952192969,
27.4912980243871));
#41951=CARTESIAN_POINT('Ctrl Pts',(18.8647241677156,0.115706281036145,27.4993767523481));
#41952=CARTESIAN_POINT('Ctrl Pts',(18.8541386322151,0.282688592136938,27.4656978713822));
#41953=CARTESIAN_POINT('Ctrl Pts',(18.8435530967146,0.43130001490854,27.3940459112129));
#41954=CARTESIAN_POINT('Ctrl Pts',(18.832967561214,0.57991143768015,27.3223939510436));
#41955=CARTESIAN_POINT('Ctrl Pts',(18.8223820257135,0.710151972122568,27.212768911671));
#41956=CARTESIAN_POINT('Ctrl Pts',(18.811796490213,0.806359128334629,27.0787183528563));
#41957=CARTESIAN_POINT('Ctrl Pts',(18.8012109547124,0.902566284546691,26.9446677940417));
#41958=CARTESIAN_POINT('Ctrl Pts',(18.7906254192119,0.964740062528397,26.7861917157849));
#41959=CARTESIAN_POINT('Ctrl Pts',(18.7800398837114,0.985058465493209,26.6224647452279));
#41960=CARTESIAN_POINT('Ctrl Pts',(18.7694543482108,1.00537686845802,26.4587377746709));
#41961=CARTESIAN_POINT('Ctrl Pts',(18.7588688127103,0.98383989640594,26.2897599118136));
#41962=CARTESIAN_POINT('Ctrl Pts',(18.7482832772098,0.923457247109937,26.1362645256848));
#41963=CARTESIAN_POINT('Ctrl Pts',(18.7376977417093,0.863074597813934,25.9827691395561));
#41964=CARTESIAN_POINT('Ctrl Pts',(18.7271122062087,0.763846271274007,25.8447562301559));
#41965=CARTESIAN_POINT('Ctrl Pts',(18.7165266707082,0.637180468464792,25.7388377815076));
#41966=CARTESIAN_POINT('Ctrl Pts',(18.7059411352077,0.510514665655577,25.6329193328593));
#41967=CARTESIAN_POINT('Ctrl Pts',(18.6953555997071,0.356411386577074,25.5590953449629));
#41968=CARTESIAN_POINT('Ctrl Pts',(18.6847700642066,0.194898297897354,25.5267127145229));
#41969=CARTESIAN_POINT('Ctrl Pts',(18.6741845287061,0.0333852092176347,
25.4943300840828));
#41970=CARTESIAN_POINT('Ctrl Pts',(18.6635989932055,-0.135537689063301,
25.5033888110992));
#41971=CARTESIAN_POINT('Ctrl Pts',(18.653013457705,-0.293477330358148,25.5521822718937));
#41972=CARTESIAN_POINT('Ctrl Pts',(18.6424279222045,-0.451416971653003,
25.6009757326883));
#41973=CARTESIAN_POINT('Ctrl Pts',(18.6318423867039,-0.598373355961768,
25.689503927261));
#41974=CARTESIAN_POINT('Ctrl Pts',(18.6212568512034,-0.712934505791141,
25.8079417618848));
#41975=CARTESIAN_POINT('Ctrl Pts',(18.6048934933477,-0.890025696966787,
25.9910256192399));
#41976=CARTESIAN_POINT('Ctrl Pts',(18.5885301354919,-0.989706308710838,
26.2455805618997));
#41977=CARTESIAN_POINT('Ctrl Pts',(18.5721667776362,-0.992013826433795,
26.5001094462548));
#41978=CARTESIAN_POINT('Ctrl Pts',(18.4278332223638,-0.992438477235227,
26.500018847878));
#41979=CARTESIAN_POINT('Ctrl Pts',(18.4345805539623,-0.992366655062056,
26.394810542483));
#41980=CARTESIAN_POINT('Ctrl Pts',(18.4413278855608,-0.975709826569298,
26.2895800603005));
#41981=CARTESIAN_POINT('Ctrl Pts',(18.4480752171592,-0.942832678942907,
26.1896879916471));
#41982=CARTESIAN_POINT('Ctrl Pts',(18.4586844200575,-0.891138120168834,
26.0326221636518));
#41983=CARTESIAN_POINT('Ctrl Pts',(18.4692936229557,-0.799342044850471,
25.8887545025172));
#41984=CARTESIAN_POINT('Ctrl Pts',(18.479902825854,-0.678680210339956,25.7756935385323));
#41985=CARTESIAN_POINT('Ctrl Pts',(18.4905120287523,-0.558018375829447,
25.6626325745473));
#41986=CARTESIAN_POINT('Ctrl Pts',(18.5011212316506,-0.408490782126793,
25.580378307712));
#41987=CARTESIAN_POINT('Ctrl Pts',(18.5117304345488,-0.248398062315547,
25.5389978519782));
#41988=CARTESIAN_POINT('Ctrl Pts',(18.5223396374471,-0.0883053425042835,
25.4976173962445));
#41989=CARTESIAN_POINT('Ctrl Pts',(18.5329488403454,0.0823525034155692,
25.4971107516123));
#41990=CARTESIAN_POINT('Ctrl Pts',(18.5435580432436,0.242688139518946,25.5375400062926));
#41991=CARTESIAN_POINT('Ctrl Pts',(18.5541672461419,0.403023775622313,25.577969260973));
#41992=CARTESIAN_POINT('Ctrl Pts',(18.5647764490402,0.553037201909199,25.659334414966));
#41993=CARTESIAN_POINT('Ctrl Pts',(18.5753856519385,0.674368074295156,25.7716769836757));
#41994=CARTESIAN_POINT('Ctrl Pts',(18.5859948548367,0.795698946681113,25.8840195523854));
#41995=CARTESIAN_POINT('Ctrl Pts',(18.596604057735,0.888347265166135,26.0273395358117));
#41996=CARTESIAN_POINT('Ctrl Pts',(18.6072132606333,0.940973566665014,26.1840957387243));
#41997=CARTESIAN_POINT('Ctrl Pts',(18.6178224635316,0.993599868163893,26.3408519416368));
#41998=CARTESIAN_POINT('Ctrl Pts',(18.6284316664298,1.00620415267662,26.5110443640355));
#41999=CARTESIAN_POINT('Ctrl Pts',(18.6390408693281,0.977243784014913,26.6738428056409));
#42000=CARTESIAN_POINT('Ctrl Pts',(18.6496500722264,0.948283415353202,26.8366412472463));
#42001=CARTESIAN_POINT('Ctrl Pts',(18.6602592751246,0.877758393517053,26.9920457080584));
#42002=CARTESIAN_POINT('Ctrl Pts',(18.6708684780229,0.774300401561698,27.121035933725));
#42003=CARTESIAN_POINT('Ctrl Pts',(18.6814776809212,0.670842409606337,27.2500261593916));
#42004=CARTESIAN_POINT('Ctrl Pts',(18.6920868838195,0.53445144753177,27.3526021499128));
#42005=CARTESIAN_POINT('Ctrl Pts',(18.7026960867178,0.381820683670061,27.416209422821));
#42006=CARTESIAN_POINT('Ctrl Pts',(18.713305289616,0.229189919808361,27.4798166957291));
#42007=CARTESIAN_POINT('Ctrl Pts',(18.7239144925143,0.0603193541595261,
27.5044552510242));
#42008=CARTESIAN_POINT('Ctrl Pts',(18.7345236954126,-0.104122613443559,
27.4871095287382));
#42009=CARTESIAN_POINT('Ctrl Pts',(18.7451328983108,-0.268564581046635,
27.4697638064523));
#42010=CARTESIAN_POINT('Ctrl Pts',(18.7557421012091,-0.428577950603957,
27.4104338065854));
#42011=CARTESIAN_POINT('Ctrl Pts',(18.7663513041074,-0.564578365915668,
27.3163810447172));
#42012=CARTESIAN_POINT('Ctrl Pts',(18.7769605070056,-0.700578781227387,
27.222328282849));
#42013=CARTESIAN_POINT('Ctrl Pts',(18.7875697099039,-0.812566242293489,
27.0935527589795));
#42014=CARTESIAN_POINT('Ctrl Pts',(18.7981789128022,-0.886834382501103,
26.9458155656893));
#42015=CARTESIAN_POINT('Ctrl Pts',(18.8080636826561,-0.956031237388956,
26.8081663786076));
#42016=CARTESIAN_POINT('Ctrl Pts',(18.8179484525099,-0.992484111373763,
26.6540566475057));
#42017=CARTESIAN_POINT('Ctrl Pts',(18.8278332223638,-0.992574927394752,
26.4999883895028));
#42018=CARTESIAN_POINT('Origin',(18.,0.,26.5));
#42019=CARTESIAN_POINT('',(19.3721667776362,-0.992405353361108,26.4996434684176));
#42020=CARTESIAN_POINT('',(19.2278332223638,-0.992414099467528,26.5000000900757));
#42021=CARTESIAN_POINT('',(18.,-0.9925,26.5));
#42022=CARTESIAN_POINT('Ctrl Pts',(19.3721667776362,-0.992405353361108,
26.4996434684176));
#42023=CARTESIAN_POINT('Ctrl Pts',(19.3653307853375,-0.992340977052407,
26.6063601754747));
#42024=CARTESIAN_POINT('Ctrl Pts',(19.3584947930388,-0.975264170858423,
26.7132672752177));
#42025=CARTESIAN_POINT('Ctrl Pts',(19.3516588007401,-0.941543675704311,
26.8144238844136));
#42026=CARTESIAN_POINT('Ctrl Pts',(19.3410732652396,-0.889327481924047,
26.9710649148549));
#42027=CARTESIAN_POINT('Ctrl Pts',(19.3304877297391,-0.797202170370003,
27.1139171148842));
#42028=CARTESIAN_POINT('Ctrl Pts',(19.3199021942385,-0.676452402081721,
27.2262843315731));
#42029=CARTESIAN_POINT('Ctrl Pts',(19.309316658738,-0.555702633793439,27.338651548262));
#42030=CARTESIAN_POINT('Ctrl Pts',(19.2987311232374,-0.406328408770916,
27.4205337816104));
#42031=CARTESIAN_POINT('Ctrl Pts',(19.2881455877369,-0.246523395998278,
27.4615425156544));
#42032=CARTESIAN_POINT('Ctrl Pts',(19.2775600522364,-0.0867183832256306,
27.5025512496983));
#42033=CARTESIAN_POINT('Ctrl Pts',(19.2669745167358,0.0835174172971379,
27.5026864844377));
#42034=CARTESIAN_POINT('Ctrl Pts',(19.2563889812353,0.243476972870307,27.462210444508));
#42035=CARTESIAN_POINT('Ctrl Pts',(19.2458034457348,0.403436528443476,27.4217344045784));
#42036=CARTESIAN_POINT('Ctrl Pts',(19.2352179102343,0.553119839067051,27.3406470899797));
#42037=CARTESIAN_POINT('Ctrl Pts',(19.2246323747337,0.674187278220771,27.2285666119654));
#42038=CARTESIAN_POINT('Ctrl Pts',(19.2140468392332,0.795254717374478,27.1164861339511));
#42039=CARTESIAN_POINT('Ctrl Pts',(19.2034613037327,0.887706285058342,26.9734124925212));
#42040=CARTESIAN_POINT('Ctrl Pts',(19.1928757682321,0.94047898641325,26.817137286811));
#42041=CARTESIAN_POINT('Ctrl Pts',(19.1822902327316,0.993251687768168,26.6608620811007));
#42042=CARTESIAN_POINT('Ctrl Pts',(19.1717046972311,1.00634552279412,26.49138531111));
#42043=CARTESIAN_POINT('Ctrl Pts',(19.1611191617305,0.977775061776517,26.3287609830781));
#42044=CARTESIAN_POINT('Ctrl Pts',(19.15053362623,0.949204600758917,26.1661366550462));
#42045=CARTESIAN_POINT('Ctrl Pts',(19.1399480907295,0.878969843697767,26.0103647689731));
#42046=CARTESIAN_POINT('Ctrl Pts',(19.1293625552289,0.776358190350592,25.8815006496868));
#42047=CARTESIAN_POINT('Ctrl Pts',(19.1187770197284,0.673746537003416,25.7526365304005));
#42048=CARTESIAN_POINT('Ctrl Pts',(19.1081914842279,0.538757987370212,25.6506801779009));
#42049=CARTESIAN_POINT('Ctrl Pts',(19.0976059487273,0.386554949372809,25.586182369478));
#42050=CARTESIAN_POINT('Ctrl Pts',(19.0870204132268,0.234351911375407,25.521684561055));
#42051=CARTESIAN_POINT('Ctrl Pts',(19.0764348777263,0.0649343850138017,
25.4946452967086));
#42052=CARTESIAN_POINT('Ctrl Pts',(19.0658493422258,-0.0989942199664423,
25.5113542819714));
#42053=CARTESIAN_POINT('Ctrl Pts',(19.0446782712247,-0.42685142992694,25.5447722524971));
#42054=CARTESIAN_POINT('Ctrl Pts',(19.0235072002236,-0.732752954362004,
25.7531832214598));
#42055=CARTESIAN_POINT('Ctrl Pts',(19.0023361292225,-0.883835619178809,
26.0460673952717));
#42056=CARTESIAN_POINT('Ctrl Pts',(18.9922796786938,-0.955601253728412,
26.1851900312712));
#42057=CARTESIAN_POINT('Ctrl Pts',(18.982223228165,-0.992434550584083,26.3433726611575));
#42058=CARTESIAN_POINT('Ctrl Pts',(18.9721667776362,-0.992230389713068,
26.5005256112294));
#42059=CARTESIAN_POINT('Ctrl Pts',(18.8278332223638,-0.992574927394752,
26.4999883895028));
#42060=CARTESIAN_POINT('Ctrl Pts',(18.8285576554082,-0.992581583101212,
26.4886970656946));
#42061=CARTESIAN_POINT('Ctrl Pts',(18.8292820884526,-0.992392934494438,
26.4774059646426));
#42062=CARTESIAN_POINT('Ctrl Pts',(18.830006521497,-0.992007557368196,26.4661215821387));
#42063=CARTESIAN_POINT('Ctrl Pts',(18.8406157243953,-0.986363772678551,
26.3008636545894));
#42064=CARTESIAN_POINT('Ctrl Pts',(18.8512249272935,-0.938527383950129,
26.1370466622021));
#42065=CARTESIAN_POINT('Ctrl Pts',(18.8618341301918,-0.854353182112096,
25.9947204921234));
#42066=CARTESIAN_POINT('Ctrl Pts',(18.8724433330901,-0.770178980274068,
25.8523943220447));
#42067=CARTESIAN_POINT('Ctrl Pts',(18.8830525359884,-0.649666965326431,
25.7315589742747));
#42068=CARTESIAN_POINT('Ctrl Pts',(18.8936617388866,-0.507566841925601,
25.6470037269119));
#42069=CARTESIAN_POINT('Ctrl Pts',(18.9042709417849,-0.365466718524772,
25.5624484795491));
#42070=CARTESIAN_POINT('Ctrl Pts',(18.9148801446832,-0.201778486670748,
25.5141733325935));
#42071=CARTESIAN_POINT('Ctrl Pts',(18.9254893475815,-0.0365362742051188,
25.5080867771853));
#42072=CARTESIAN_POINT('Ctrl Pts',(18.9360985504797,0.128705938260501,25.5020002217771));
#42073=CARTESIAN_POINT('Ctrl Pts',(18.946707753378,0.295502131337727,25.5381022579163));
#42074=CARTESIAN_POINT('Ctrl Pts',(18.9573169562763,0.443437787775487,25.6119742856872));
#42075=CARTESIAN_POINT('Ctrl Pts',(18.9679261591746,0.591373444213265,25.6858463134581));
#42076=CARTESIAN_POINT('Ctrl Pts',(18.9785353620728,0.720448564011572,25.7974883328607));
#42077=CARTESIAN_POINT('Ctrl Pts',(18.9891445649711,0.814865386913012,25.93323625545));
#42078=CARTESIAN_POINT('Ctrl Pts',(18.9997537678693,0.909282209814446,26.0689841780393));
#42079=CARTESIAN_POINT('Ctrl Pts',(19.0103629707676,0.969040735819015,26.2288380038151));
#42080=CARTESIAN_POINT('Ctrl Pts',(19.0209721736659,0.986827000272459,26.3932329055939));
#42081=CARTESIAN_POINT('Ctrl Pts',(19.0315813765642,1.0046132647259,26.5576278073727));
#42082=CARTESIAN_POINT('Ctrl Pts',(19.0421905794624,0.980427267628221,26.7265637851543));
#42083=CARTESIAN_POINT('Ctrl Pts',(19.0527997823607,0.917229181186273,26.8793644291443));
#42084=CARTESIAN_POINT('Ctrl Pts',(19.063408985259,0.854031094744325,27.0321650731344));
#42085=CARTESIAN_POINT('Ctrl Pts',(19.0740181881573,0.751820918958111,27.1688303833328));
#42086=CARTESIAN_POINT('Ctrl Pts',(19.0846273910556,0.623108360217072,27.2726336210298));
#42087=CARTESIAN_POINT('Ctrl Pts',(19.0952365939538,0.494395801476034,27.3764368587268));
#42088=CARTESIAN_POINT('Ctrl Pts',(19.1058457968521,0.339180859780171,27.4473780239223));
#42089=CARTESIAN_POINT('Ctrl Pts',(19.1164549997504,0.176460600070971,27.4767744865324));
#42090=CARTESIAN_POINT('Ctrl Pts',(19.1270642026486,0.0137403403617714,
27.5061709491426));
#42091=CARTESIAN_POINT('Ctrl Pts',(19.1376734055469,-0.156485237360765,
27.4940227091673));
#42092=CARTESIAN_POINT('Ctrl Pts',(19.1482826084452,-0.313381886600382,
27.441816613821));
#42093=CARTESIAN_POINT('Ctrl Pts',(19.1588918113435,-0.470278535839999,
27.3896105184747));
#42094=CARTESIAN_POINT('Ctrl Pts',(19.1695010142417,-0.613846256596695,
27.2973465677573));
#42095=CARTESIAN_POINT('Ctrl Pts',(19.18011021714,-0.726513510427623,27.1763171298173));
#42096=CARTESIAN_POINT('Ctrl Pts',(19.1907194200383,-0.839180764258558,
27.0552876918772));
#42097=CARTESIAN_POINT('Ctrl Pts',(19.2013286229365,-0.92094755116372,26.9054927667144));
#42098=CARTESIAN_POINT('Ctrl Pts',(19.2119378258348,-0.961806271719183,
26.7452660526856));
#42099=CARTESIAN_POINT('Ctrl Pts',(19.2172362913445,-0.982212000943896,
26.6652453644069));
#42100=CARTESIAN_POINT('Ctrl Pts',(19.2225347568541,-0.992414359490076,
26.5826227587524));
#42101=CARTESIAN_POINT('Ctrl Pts',(19.2278332223638,-0.992414099682224,
26.5000000900755));
#42102=CARTESIAN_POINT('Origin',(18.,0.,26.5));
#42103=CARTESIAN_POINT('',(19.7721667776362,-0.992492903155771,26.500016853248));
#42104=CARTESIAN_POINT('',(19.6278332223638,-0.992575270015615,26.5000114296632));
#42105=CARTESIAN_POINT('',(18.,-0.9925,26.5));
#42106=CARTESIAN_POINT('Ctrl Pts',(19.7721667776362,-0.992492903155771,
26.500016853248));
#42107=CARTESIAN_POINT('Ctrl Pts',(19.7696094135111,-0.992505792531705,
26.5398596057124));
#42108=CARTESIAN_POINT('Ctrl Pts',(19.767052049386,-0.990124581390803,26.5797014438245));
#42109=CARTESIAN_POINT('Ctrl Pts',(19.7644946852609,-0.985319177046528,
26.6192598084646));
#42110=CARTESIAN_POINT('Ctrl Pts',(19.7539091497603,-0.965428470916284,
26.783001244081));
#42111=CARTESIAN_POINT('Ctrl Pts',(19.7433236142598,-0.904003382287043,
26.9418858491443));
#42112=CARTESIAN_POINT('Ctrl Pts',(19.7327380787593,-0.80825773862658,27.0762440647293));
#42113=CARTESIAN_POINT('Ctrl Pts',(19.7221525432587,-0.712512094966116,
27.2106022803143));
#42114=CARTESIAN_POINT('Ctrl Pts',(19.7115670077582,-0.582445896274432,
27.3204341064211));
#42115=CARTESIAN_POINT('Ctrl Pts',(19.7009814722577,-0.434059675387492,
27.3925929498046));
#42116=CARTESIAN_POINT('Ctrl Pts',(19.6903959367571,-0.285673454500552,
27.4647517931881));
#42117=CARTESIAN_POINT('Ctrl Pts',(19.6798104012566,-0.118967211418359,
27.4992376538483));
#42118=CARTESIAN_POINT('Ctrl Pts',(19.6692248657561,0.0458380169416741,
27.4915829115048));
#42119=CARTESIAN_POINT('Ctrl Pts',(19.6586393302555,0.210643245301707,27.4839281691613));
#42120=CARTESIAN_POINT('Ctrl Pts',(19.648053794755,0.373547458939575,27.4341328238141));
#42121=CARTESIAN_POINT('Ctrl Pts',(19.6374682592545,0.51462458881678,27.3486685543578));
#42122=CARTESIAN_POINT('Ctrl Pts',(19.6268827237539,0.655701718694,27.2632042849015));
#42123=CARTESIAN_POINT('Ctrl Pts',(19.6162971882534,0.774951764810546,27.1420710913361));
#42124=CARTESIAN_POINT('Ctrl Pts',(19.6057116527529,0.857930614775059,26.9993214721802));
#42125=CARTESIAN_POINT('Ctrl Pts',(19.5951261172524,0.940909464739562,26.8565718530243));
#42126=CARTESIAN_POINT('Ctrl Pts',(19.5845405817518,0.987617118552037,26.6922058082778));
#42127=CARTESIAN_POINT('Ctrl Pts',(19.5739550462513,0.992227228213515,26.5275429419996));
#42128=CARTESIAN_POINT('Ctrl Pts',(19.5633695107507,0.996837337874994,26.3628800757214));
#42129=CARTESIAN_POINT('Ctrl Pts',(19.5527839752502,0.959349903385473,26.1979203879114));
#42130=CARTESIAN_POINT('Ctrl Pts',(19.5421984397497,0.884556620605071,26.0505036421938));
#42131=CARTESIAN_POINT('Ctrl Pts',(19.5316129042492,0.809763337824661,25.9030868964762));
#42132=CARTESIAN_POINT('Ctrl Pts',(19.5210273687486,0.697664206753381,25.773213092851));
#42133=CARTESIAN_POINT('Ctrl Pts',(19.5104418332481,0.561562925403105,25.680324886204));
#42134=CARTESIAN_POINT('Ctrl Pts',(19.489270762247,0.289360362702577,25.4945484729099));
#42135=CARTESIAN_POINT('Ctrl Pts',(19.468099691246,-0.0788508011138748,
25.456714447529));
#42136=CARTESIAN_POINT('Ctrl Pts',(19.4469286202449,-0.383144249725361,
25.5832553816541));
#42137=CARTESIAN_POINT('Ctrl Pts',(19.4363430847444,-0.535290974031126,
25.6465258487166));
#42138=CARTESIAN_POINT('Ctrl Pts',(19.4257575492438,-0.671458269535649,
25.7508900556557));
#42139=CARTESIAN_POINT('Ctrl Pts',(19.4151720137433,-0.774666660030811,
25.8800169707371));
#42140=CARTESIAN_POINT('Ctrl Pts',(19.4045864782428,-0.877875050525961,
26.0091438858185));
#42141=CARTESIAN_POINT('Ctrl Pts',(19.3940009427422,-0.948124536011754,
26.1630335090423));
#42142=CARTESIAN_POINT('Ctrl Pts',(19.3834154072417,-0.977095740751408,
26.3251932510807));
#42143=CARTESIAN_POINT('Ctrl Pts',(19.3796658640399,-0.987357742496616,
26.3826324763651));
#42144=CARTESIAN_POINT('Ctrl Pts',(19.375916320838,-0.99244066377986,26.4411093323356));
#42145=CARTESIAN_POINT('Ctrl Pts',(19.3721667776362,-0.992405353361108,
26.4996434684176));
#42146=CARTESIAN_POINT('Ctrl Pts',(19.2278332223638,-0.992414099682224,
26.5000000900755));
#42147=CARTESIAN_POINT('Ctrl Pts',(19.2331439597524,-0.992413839272626,
26.4171860574298));
#42148=CARTESIAN_POINT('Ctrl Pts',(19.238454697141,-0.98216364481267,26.3343719614693));
#42149=CARTESIAN_POINT('Ctrl Pts',(19.2437654345296,-0.961664273866392,
26.254177777068));
#42150=CARTESIAN_POINT('Ctrl Pts',(19.2543746374279,-0.920712901252369,
26.0939747183739));
#42151=CARTESIAN_POINT('Ctrl Pts',(19.2649838403262,-0.838859501818548,
25.9442271038806));
#42152=CARTESIAN_POINT('Ctrl Pts',(19.2755930432245,-0.726122275667864,
25.8232628414981));
#42153=CARTESIAN_POINT('Ctrl Pts',(19.2862022461227,-0.613385049517181,
25.7022985791156));
#42154=CARTESIAN_POINT('Ctrl Pts',(19.296811449021,-0.469763996649633,25.6101176688438));
#42155=CARTESIAN_POINT('Ctrl Pts',(19.3074206519193,-0.312837182931623,
25.5580023153459));
#42156=CARTESIAN_POINT('Ctrl Pts',(19.3180298548175,-0.15591036921363,25.505886961848));
#42157=CARTESIAN_POINT('Ctrl Pts',(19.3286390577158,0.0143222053548266,
25.4938371651239));
#42158=CARTESIAN_POINT('Ctrl Pts',(19.3392482606141,0.177025437920684,25.5233277237234));
#42159=CARTESIAN_POINT('Ctrl Pts',(19.3498574635124,0.33972867048655,25.552818282323));
#42160=CARTESIAN_POINT('Ctrl Pts',(19.3604666664106,0.494902561049821,25.6238491962462));
#42161=CARTESIAN_POINT('Ctrl Pts',(19.3710758693089,0.623555068996665,25.7277268508832));
#42162=CARTESIAN_POINT('Ctrl Pts',(19.3816850722072,0.752207576943509,25.8316045055202));
#42163=CARTESIAN_POINT('Ctrl Pts',(19.3922942751055,0.854338702273929,25.968328900871));
#42164=CARTESIAN_POINT('Ctrl Pts',(19.4029034780037,0.917448413744468,26.1211660666783));
#42165=CARTESIAN_POINT('Ctrl Pts',(19.413512680902,0.98055812521501,26.2740032324856));
#42166=CARTESIAN_POINT('Ctrl Pts',(19.4241218838003,1.00464642282567,26.4429531687493));
#42167=CARTESIAN_POINT('Ctrl Pts',(19.4347310866985,0.986765091996794,26.6073377572656));
#42168=CARTESIAN_POINT('Ctrl Pts',(19.4453402895968,0.968883761167923,26.7717223457819));
#42169=CARTESIAN_POINT('Ctrl Pts',(19.4559494924951,0.909032801899521,26.9315415865509));
#42170=CARTESIAN_POINT('Ctrl Pts',(19.4665586953933,0.814537491949821,27.0672348853221));
#42171=CARTESIAN_POINT('Ctrl Pts',(19.4771678982916,0.720042182000127,27.2029281840933));
#42172=CARTESIAN_POINT('Ctrl Pts',(19.4877771011899,0.590902521369115,27.3144955408667));
#42173=CARTESIAN_POINT('Ctrl Pts',(19.4983863040882,0.442924169569878,27.388282005294));
#42174=CARTESIAN_POINT('Ctrl Pts',(19.5089955069864,0.294945817770624,27.4620684697212));
#42175=CARTESIAN_POINT('Ctrl Pts',(19.5196047098847,0.128128774803148,27.4980740418023));
#42176=CARTESIAN_POINT('Ctrl Pts',(19.530213912783,-0.0371098901747996,
27.4918919280695));
#42177=CARTESIAN_POINT('Ctrl Pts',(19.5408231156813,-0.202348555152747,
27.4857098143367));
#42178=CARTESIAN_POINT('Ctrl Pts',(19.5514323185795,-0.366008842141143,
27.4373400147901));
#42179=CARTESIAN_POINT('Ctrl Pts',(19.5620415214778,-0.508060043615217,
27.3527026052499));
#42180=CARTESIAN_POINT('Ctrl Pts',(19.5726507243761,-0.650111245089282,
27.2680651957097));
#42181=CARTESIAN_POINT('Ctrl Pts',(19.5832599272743,-0.770553361049032,
27.147160176176));
#42182=CARTESIAN_POINT('Ctrl Pts',(19.5938691301726,-0.854645241745505,
27.0047853520854));
#42183=CARTESIAN_POINT('Ctrl Pts',(19.6044783330709,-0.938737122441978,
26.8624105279949));
#42184=CARTESIAN_POINT('Ctrl Pts',(19.6150875359692,-0.986478767875177,
26.6985658993474));
#42185=CARTESIAN_POINT('Ctrl Pts',(19.6256967388675,-0.992026983254105,
26.5333047356095));
#42186=CARTESIAN_POINT('Ctrl Pts',(19.6264089000329,-0.992399416844861,
26.5222112930482));
#42187=CARTESIAN_POINT('Ctrl Pts',(19.6271210611984,-0.992581726893453,
26.5111114675817));
#42188=CARTESIAN_POINT('Ctrl Pts',(19.6278332223638,-0.992575270015615,
26.5000114296632));
#42189=CARTESIAN_POINT('Origin',(18.,0.,26.5));
#42190=CARTESIAN_POINT('',(20.1721667776362,-0.9925,26.5000000000001));
#42191=CARTESIAN_POINT('',(20.0278332223638,-0.992438391306935,26.4999811413391));
#42192=CARTESIAN_POINT('',(18.,-0.9925,26.5));
#42193=CARTESIAN_POINT('Ctrl Pts',(20.1721667776362,-0.992597511301432,
26.4999846070725));
#42194=CARTESIAN_POINT('Ctrl Pts',(20.1633025061841,-0.992451437885555,
26.6381508584163));
#42195=CARTESIAN_POINT('Ctrl Pts',(20.1544382347321,-0.963248274446475,
26.7763584278731));
#42196=CARTESIAN_POINT('Ctrl Pts',(20.14557396328,-0.907195507711203,26.9026490862115));
#42197=CARTESIAN_POINT('Ctrl Pts',(20.1349884277795,-0.840258415882739,
27.0534628619918));
#42198=CARTESIAN_POINT('Ctrl Pts',(20.124402892279,-0.735032022423416,27.1872823381065));
#42199=CARTESIAN_POINT('Ctrl Pts',(20.1138173567784,-0.60409658984389,27.2876579868982));
#42200=CARTESIAN_POINT('Ctrl Pts',(20.1032318212779,-0.473161157264348,
27.3880336356899));
#42201=CARTESIAN_POINT('Ctrl Pts',(20.0926462857774,-0.316516685564598,
27.4549654571587));
#42202=CARTESIAN_POINT('Ctrl Pts',(20.0820607502768,-0.153569034970045,
27.4805576648362));
#42203=CARTESIAN_POINT('Ctrl Pts',(20.0714752147763,0.00937861562448072,
27.5061498725137));
#42204=CARTESIAN_POINT('Ctrl Pts',(20.0608896792758,0.178629445113807,27.4904024663998));
#42205=CARTESIAN_POINT('Ctrl Pts',(20.0503041437752,0.334082461328613,27.4347490472748));
#42206=CARTESIAN_POINT('Ctrl Pts',(20.0397186082747,0.489535477543428,27.3790956281497));
#42207=CARTESIAN_POINT('Ctrl Pts',(20.0291330727742,0.63119068048372,27.2835361960135));
#42208=CARTESIAN_POINT('Ctrl Pts',(20.0185475372736,0.740851630053171,27.1606151287322));
#42209=CARTESIAN_POINT('Ctrl Pts',(20.0079620017731,0.850512579622629,27.0376940614509));
#42210=CARTESIAN_POINT('Ctrl Pts',(19.9973764662726,0.928179275821242,26.8874113590246));
#42211=CARTESIAN_POINT('Ctrl Pts',(19.986790930772,0.966016269521608,26.726494939804));
#42212=CARTESIAN_POINT('Ctrl Pts',(19.9762053952715,1.00385326322197,26.5655785205835));
#42213=CARTESIAN_POINT('Ctrl Pts',(19.965619859771,1.00186055442409,26.3940283845687));
#42214=CARTESIAN_POINT('Ctrl Pts',(19.9550343242704,0.957677353194437,26.2352844950851));
#42215=CARTESIAN_POINT('Ctrl Pts',(19.9338632532694,0.869310950735119,25.9177967161179));
#42216=CARTESIAN_POINT('Ctrl Pts',(19.9126921822683,0.612182578548673,25.6515339232753));
#42217=CARTESIAN_POINT('Ctrl Pts',(19.8915211112673,0.297971613651096,25.5521428753119));
#42218=CARTESIAN_POINT('Ctrl Pts',(19.8809355757667,0.14086613120232,25.5024473513302));
#42219=CARTESIAN_POINT('Ctrl Pts',(19.8703500402662,-0.0305099994242361,
25.4944697635683));
#42220=CARTESIAN_POINT('Ctrl Pts',(19.8597645047656,-0.192648711794436,
25.5266686768725));
#42221=CARTESIAN_POINT('Ctrl Pts',(19.8491789692651,-0.354787424164644,
25.5588675901767));
#42222=CARTESIAN_POINT('Ctrl Pts',(19.8385934337646,-0.507688718278495,
25.631243004547));
#42223=CARTESIAN_POINT('Ctrl Pts',(19.8280078982641,-0.63436145167657,25.7365479486641));
#42224=CARTESIAN_POINT('Ctrl Pts',(19.8174223627635,-0.761034185074659,
25.8418528927812));
#42225=CARTESIAN_POINT('Ctrl Pts',(19.806836827263,-0.861478357756966,25.9800873666451));
#42226=CARTESIAN_POINT('Ctrl Pts',(19.7962512917625,-0.922522282282495,
26.1335037366619));
#42227=CARTESIAN_POINT('Ctrl Pts',(19.788223120387,-0.968818578534504,26.249856179127));
#42228=CARTESIAN_POINT('Ctrl Pts',(19.7801949490116,-0.992452440353502,
26.37494102157));
#42229=CARTESIAN_POINT('Ctrl Pts',(19.7721667776362,-0.992492903155771,
26.500016853248));
#42230=CARTESIAN_POINT('Ctrl Pts',(19.6278332223638,-0.992575270015615,
26.5000114296632));
#42231=CARTESIAN_POINT('Ctrl Pts',(19.6377302640966,-0.992485537532951,
26.3457520515285));
#42232=CARTESIAN_POINT('Ctrl Pts',(19.6476273058294,-0.955938871864007,
26.1914516421247));
#42233=CARTESIAN_POINT('Ctrl Pts',(19.6575243475622,-0.886576419823079,
26.0536716536764));
#42234=CARTESIAN_POINT('Ctrl Pts',(19.6681335504605,-0.812222855688468,
25.9059774343096));
#42235=CARTESIAN_POINT('Ctrl Pts',(19.6787427533588,-0.700160942094587,
25.7772666944042));
#42236=CARTESIAN_POINT('Ctrl Pts',(19.6893519562571,-0.564106159181243,
25.683292597014));
#42237=CARTESIAN_POINT('Ctrl Pts',(19.6999611591554,-0.428051376267899,
25.5893184996239));
#42238=CARTESIAN_POINT('Ctrl Pts',(19.7105703620536,-0.268003724035092,
25.5300810447489));
#42239=CARTESIAN_POINT('Ctrl Pts',(19.7211795649519,-0.103551752465798,
25.5128304221262));
#42240=CARTESIAN_POINT('Ctrl Pts',(19.7317887678502,0.060900219103496,25.4955797995036));
#42241=CARTESIAN_POINT('Ctrl Pts',(19.7423979707484,0.229756510009277,25.5203160091333));
#42242=CARTESIAN_POINT('Ctrl Pts',(19.7530071736467,0.382350463488992,25.5840115371971));
#42243=CARTESIAN_POINT('Ctrl Pts',(19.763616376545,0.534944416968706,25.6477070652609));
#42244=CARTESIAN_POINT('Ctrl Pts',(19.7742255794432,0.671276033022354,25.7503619117588));
#42245=CARTESIAN_POINT('Ctrl Pts',(19.7848347823415,0.774659414430762,25.8794119461736));
#42246=CARTESIAN_POINT('Ctrl Pts',(19.7954439852398,0.87804279583917,26.0084619805884));
#42247=CARTESIAN_POINT('Ctrl Pts',(19.8060531881381,0.948477942602338,26.1639072029201));
#42248=CARTESIAN_POINT('Ctrl Pts',(19.8166623910364,0.977344157236233,26.3267223637209));
#42249=CARTESIAN_POINT('Ctrl Pts',(19.8272715939346,1.00621037187013,26.4895375245218));
#42250=CARTESIAN_POINT('Ctrl Pts',(19.8378807968329,0.993507654374749,26.6597226237918));
#42251=CARTESIAN_POINT('Ctrl Pts',(19.8484899997312,0.940790715569691,26.8164483692739));
#42252=CARTESIAN_POINT('Ctrl Pts',(19.8590992026294,0.888073776764639,26.973174114756));
#42253=CARTESIAN_POINT('Ctrl Pts',(19.8697084055277,0.795342616649919,27.1164405064502));
#42254=CARTESIAN_POINT('Ctrl Pts',(19.880317608426,0.67394678605958,27.2287128861755));
#42255=CARTESIAN_POINT('Ctrl Pts',(19.8909268113243,0.552550955469226,27.3409852659008));
#42256=CARTESIAN_POINT('Ctrl Pts',(19.9015360142225,0.402490454403247,27.4222636336571));
#42257=CARTESIAN_POINT('Ctrl Pts',(19.9121452171208,0.242131485580603,27.4626001686104));
#42258=CARTESIAN_POINT('Ctrl Pts',(19.9227544200191,0.08177251675796,27.5029367035637));
#42259=CARTESIAN_POINT('Ctrl Pts',(19.9333636229173,-0.0888849198213473,
27.5023314057139));
#42260=CARTESIAN_POINT('Ctrl Pts',(19.9439728258156,-0.248953721599025,
27.460858358667));
#42261=CARTESIAN_POINT('Ctrl Pts',(19.9545820287139,-0.409022523376694,
27.4193853116201));
#42262=CARTESIAN_POINT('Ctrl Pts',(19.9651912316122,-0.558502690352734,
27.3370445153759));
#42263=CARTESIAN_POINT('Ctrl Pts',(19.9758004345104,-0.679099048049894,
27.2239138235011));
#42264=CARTESIAN_POINT('Ctrl Pts',(19.9864096374087,-0.799695405747047,
27.1107831316263));
#42265=CARTESIAN_POINT('Ctrl Pts',(19.997018840307,-0.891407954165323,26.9668625441208));
#42266=CARTESIAN_POINT('Ctrl Pts',(20.0076280432052,-0.943011812378983,
26.8097667874901));
#42267=CARTESIAN_POINT('Ctrl Pts',(20.0143631029248,-0.975771584263756,
26.7100374003971));
#42268=CARTESIAN_POINT('Ctrl Pts',(20.0210981626443,-0.992367094517968,
26.6049982692141));
#42269=CARTESIAN_POINT('Ctrl Pts',(20.0278332223638,-0.992438391306935,
26.4999811413391));
#42270=CARTESIAN_POINT('Origin',(18.,0.,26.5));
#42271=CARTESIAN_POINT('',(20.5721667776362,-0.9925,26.5));
#42272=CARTESIAN_POINT('',(20.4278332223638,-0.992514693241506,26.5000253500233));
#42273=CARTESIAN_POINT('',(18.,-0.9925,26.5));
#42274=CARTESIAN_POINT('Ctrl Pts',(20.5721667776362,-0.9925,26.5000000000001));
#42275=CARTESIAN_POINT('Ctrl Pts',(20.5554259338597,-0.99249999999998,26.760992324923));
#42276=CARTESIAN_POINT('Ctrl Pts',(20.5386850900831,-0.884539443097369,
27.0203491301748));
#42277=CARTESIAN_POINT('Ctrl Pts',(20.5219442463066,-0.699346033936857,
27.2042523516587));
#42278=CARTESIAN_POINT('Ctrl Pts',(20.5052034025301,-0.514152624776344,
27.3881555731426));
#42279=CARTESIAN_POINT('Ctrl Pts',(20.4884625587535,-0.25404740834438,27.4943003359057));
#42280=CARTESIAN_POINT('Ctrl Pts',(20.471721714977,0.00693853867355432,
27.4924757461425));
#42281=CARTESIAN_POINT('Ctrl Pts',(20.4549808712005,0.267924485691489,27.4906511563793));
#42282=CARTESIAN_POINT('Ctrl Pts',(20.4382400274239,0.526520203888113,27.3808800818308));
#42283=CARTESIAN_POINT('Ctrl Pts',(20.4214991836474,0.709124249559362,27.1944055361868));
#42284=CARTESIAN_POINT('Ctrl Pts',(20.4047583398709,0.89172829523061,27.0079309905428));
#42285=CARTESIAN_POINT('Ctrl Pts',(20.3880174960943,0.996052076106205,26.7470900753838));
#42286=CARTESIAN_POINT('Ctrl Pts',(20.3712766523178,0.992402985755317,26.486123261769));
#42287=CARTESIAN_POINT('Ctrl Pts',(20.3545358085413,0.98875389540443,26.2251564481542));
#42288=CARTESIAN_POINT('Ctrl Pts',(20.3377949647647,0.877177668191485,25.9673344556902));
#42289=CARTESIAN_POINT('Ctrl Pts',(20.3210541209882,0.689431099871631,25.7860385104715));
#42290=CARTESIAN_POINT('Ctrl Pts',(20.3043132772117,0.501684531551776,25.6047425652527));
#42291=CARTESIAN_POINT('Ctrl Pts',(20.2875724334351,0.240120666075644,25.5022448650134));
#42292=CARTESIAN_POINT('Ctrl Pts',(20.2708315896586,-0.0208142595729757,
25.5077182776054));
#42293=CARTESIAN_POINT('Ctrl Pts',(20.2540907458821,-0.281749185221595,
25.5131916901973));
#42294=CARTESIAN_POINT('Ctrl Pts',(20.2373499021055,-0.538784851090647,
25.6265676168679));
#42295=CARTESIAN_POINT('Ctrl Pts',(20.220609058329,-0.718763835149603,25.8155770318867));
#42296=CARTESIAN_POINT('Ctrl Pts',(20.2044616314314,-0.892363059118839,
25.9978865828696));
#42297=CARTESIAN_POINT('Ctrl Pts',(20.1883142045338,-0.992500000000014,
26.248259135335));
#42298=CARTESIAN_POINT('Ctrl Pts',(20.1721667776362,-0.9925,26.5000000000001));
#42299=CARTESIAN_POINT('Ctrl Pts',(20.0278332223638,-0.992438391306935,
26.4999811413391));
#42300=CARTESIAN_POINT('Ctrl Pts',(20.0317073655426,-0.992479402668399,
26.4395731558791));
#42301=CARTESIAN_POINT('Ctrl Pts',(20.0355815087213,-0.987052908523862,
26.3791724508387));
#42302=CARTESIAN_POINT('Ctrl Pts',(20.0394556519001,-0.97609039996612,26.3197938069537));
#42303=CARTESIAN_POINT('Ctrl Pts',(20.0500648547983,-0.946069961330555,
26.1571875088038));
#42304=CARTESIAN_POINT('Ctrl Pts',(20.0606740576966,-0.874533916050388,
26.0022458382598));
#42305=CARTESIAN_POINT('Ctrl Pts',(20.0712832605949,-0.77023770276533,25.8739324140662));
#42306=CARTESIAN_POINT('Ctrl Pts',(20.0818924634931,-0.66594148948026,25.7456189898725));
#42307=CARTESIAN_POINT('Ctrl Pts',(20.0925016663914,-0.528885108190297,
25.6439338120293));
#42308=CARTESIAN_POINT('Ctrl Pts',(20.1031108692897,-0.375843161571139,
25.5813223313814));
#42309=CARTESIAN_POINT('Ctrl Pts',(20.113720072188,-0.222801214951989,25.5187108507335));
#42310=CARTESIAN_POINT('Ctrl Pts',(20.1243292750862,-0.0537737030036256,
25.495173067281));
#42311=CARTESIAN_POINT('Ctrl Pts',(20.1349384779845,0.110551761427937,25.5135898170825));
#42312=CARTESIAN_POINT('Ctrl Pts',(20.1455476808828,0.27487722585949,25.5320065668839));
#42313=CARTESIAN_POINT('Ctrl Pts',(20.1561568837811,0.434500642774264,25.5923778499392));
#42314=CARTESIAN_POINT('Ctrl Pts',(20.1667660866793,0.569885385192319,25.6873147050288));
#42315=CARTESIAN_POINT('Ctrl Pts',(20.1773752895776,0.705270127610389,25.7822515601183));
#42316=CARTESIAN_POINT('Ctrl Pts',(20.1879844924759,0.816416195531731,25.911753987242));
#42317=CARTESIAN_POINT('Ctrl Pts',(20.1985936953741,0.889720200987109,26.0599719271754));
#42318=CARTESIAN_POINT('Ctrl Pts',(20.2092028982724,0.963024206442483,26.2081898671088));
#42319=CARTESIAN_POINT('Ctrl Pts',(20.2198121011707,0.998486149431895,26.3751233198519));
#42320=CARTESIAN_POINT('Ctrl Pts',(20.230421304069,0.991765772331754,26.5403409686232));
#42321=CARTESIAN_POINT('Ctrl Pts',(20.2410305069672,0.985045395231612,26.7055586173945));
#42322=CARTESIAN_POINT('Ctrl Pts',(20.2516397098655,0.936142698041916,26.8690604621941));
#42323=CARTESIAN_POINT('Ctrl Pts',(20.2622489127638,0.851042978983781,27.0108351875514));
#42324=CARTESIAN_POINT('Ctrl Pts',(20.272858115662,0.765943259925651,27.1526099129086));
#42325=CARTESIAN_POINT('Ctrl Pts',(20.2834673185603,0.644646518999089,27.2726575188235));
#42326=CARTESIAN_POINT('Ctrl Pts',(20.2940765214586,0.501998505199868,27.3562851404149));
#42327=CARTESIAN_POINT('Ctrl Pts',(20.3046857243569,0.359350491400631,27.4399127620063));
#42328=CARTESIAN_POINT('Ctrl Pts',(20.3152949272551,0.195351204728735,27.4871203992742));
#42329=CARTESIAN_POINT('Ctrl Pts',(20.3259041301534,0.0300728435533973,
27.4921302157474));
#42330=CARTESIAN_POINT('Ctrl Pts',(20.3365133330517,-0.135205517621921,
27.4971400322205));
#42331=CARTESIAN_POINT('Ctrl Pts',(20.34712253595,-0.301762953300702,27.459952027899));
#42332=CARTESIAN_POINT('Ctrl Pts',(20.3577317388482,-0.449214168176698,
27.3851177164804));
#42333=CARTESIAN_POINT('Ctrl Pts',(20.3683409417465,-0.596665383052711,
27.3102834050619));
#42334=CARTESIAN_POINT('Ctrl Pts',(20.3789501446448,-0.725010377125957,
27.1978027865463));
#42335=CARTESIAN_POINT('Ctrl Pts',(20.3895593475431,-0.818540751701458,
27.0614425872004));
#42336=CARTESIAN_POINT('Ctrl Pts',(20.4001685504413,-0.912071126276949,
26.9250823878545));
#42337=CARTESIAN_POINT('Ctrl Pts',(20.4107777533396,-0.9707868813547,26.7648426076782));
#42338=CARTESIAN_POINT('Ctrl Pts',(20.4213869562379,-0.987501679071689,
26.600335311575));
#42339=CARTESIAN_POINT('Ctrl Pts',(20.4235357116132,-0.99088704287197,26.5670165090062));
#42340=CARTESIAN_POINT('Ctrl Pts',(20.4256844669885,-0.99254947667873,26.5335226477804));
#42341=CARTESIAN_POINT('Ctrl Pts',(20.4278332223638,-0.992514693241506,
26.5000253500233));
#42342=CARTESIAN_POINT('Origin',(18.,0.,26.5));
#42343=CARTESIAN_POINT('',(20.9721667776362,-0.9925,26.5000000000001));
#42344=CARTESIAN_POINT('',(20.8278332223638,-0.992500311415872,26.4999739716271));
#42345=CARTESIAN_POINT('',(18.,-0.9925,26.5));
#42346=CARTESIAN_POINT('Ctrl Pts',(20.9721667776362,-0.9925,26.5000000000001));
#42347=CARTESIAN_POINT('Ctrl Pts',(20.9554259338597,-0.992499999999982,
26.760992324923));
#42348=CARTESIAN_POINT('Ctrl Pts',(20.9386850900831,-0.884539443097373,
27.0203491301748));
#42349=CARTESIAN_POINT('Ctrl Pts',(20.9219442463066,-0.699346033936861,
27.2042523516587));
#42350=CARTESIAN_POINT('Ctrl Pts',(20.9052034025301,-0.51415262477635,27.3881555731426));
#42351=CARTESIAN_POINT('Ctrl Pts',(20.8884625587535,-0.254047408344387,
27.4943003359057));
#42352=CARTESIAN_POINT('Ctrl Pts',(20.871721714977,0.00693853867354749,
27.4924757461425));
#42353=CARTESIAN_POINT('Ctrl Pts',(20.8549808712005,0.267924485691482,27.4906511563793));
#42354=CARTESIAN_POINT('Ctrl Pts',(20.8382400274239,0.526520203888107,27.3808800818308));
#42355=CARTESIAN_POINT('Ctrl Pts',(20.8214991836474,0.709124249559357,27.1944055361868));
#42356=CARTESIAN_POINT('Ctrl Pts',(20.8047583398709,0.891728295230606,27.0079309905428));
#42357=CARTESIAN_POINT('Ctrl Pts',(20.7880174960943,0.996052076106204,26.7470900753838));
#42358=CARTESIAN_POINT('Ctrl Pts',(20.7712766523178,0.992402985755318,26.486123261769));
#42359=CARTESIAN_POINT('Ctrl Pts',(20.7545358085413,0.988753895404431,26.2251564481542));
#42360=CARTESIAN_POINT('Ctrl Pts',(20.7377949647647,0.877177668191489,25.9673344556903));
#42361=CARTESIAN_POINT('Ctrl Pts',(20.7210541209882,0.689431099871636,25.7860385104715));
#42362=CARTESIAN_POINT('Ctrl Pts',(20.7043132772117,0.501684531551782,25.6047425652527));
#42363=CARTESIAN_POINT('Ctrl Pts',(20.6875724334351,0.240120666075651,25.5022448650134));
#42364=CARTESIAN_POINT('Ctrl Pts',(20.6708315896586,-0.020814259572969,
25.5077182776054));
#42365=CARTESIAN_POINT('Ctrl Pts',(20.6540907458821,-0.281749185221589,
25.5131916901973));
#42366=CARTESIAN_POINT('Ctrl Pts',(20.6373499021055,-0.538784851090641,
25.6265676168679));
#42367=CARTESIAN_POINT('Ctrl Pts',(20.620609058329,-0.718763835149599,25.8155770318867));
#42368=CARTESIAN_POINT('Ctrl Pts',(20.6044616314314,-0.892363059118843,
25.9978865828696));
#42369=CARTESIAN_POINT('Ctrl Pts',(20.5883142045338,-0.99250000000002,26.248259135335));
#42370=CARTESIAN_POINT('Ctrl Pts',(20.5721667776362,-0.9925,26.5000000000001));
#42371=CARTESIAN_POINT('Ctrl Pts',(20.4278332223638,-0.992514693241506,
26.5000253500233));
#42372=CARTESIAN_POINT('Ctrl Pts',(20.4362936698868,-0.992377737937666,
26.368134054676));
#42373=CARTESIAN_POINT('Ctrl Pts',(20.4447541174097,-0.965929007104012,
26.2361894831557));
#42374=CARTESIAN_POINT('Ctrl Pts',(20.4532145649327,-0.914738023432971,
26.114667559886));
#42375=CARTESIAN_POINT('Ctrl Pts',(20.463823767831,-0.850545729721046,25.9622819163303));
#42376=CARTESIAN_POINT('Ctrl Pts',(20.4744329707292,-0.747447301940976,
25.8262854412488));
#42377=CARTESIAN_POINT('Ctrl Pts',(20.4850421736275,-0.618061161403927,
25.7233230132917));
#42378=CARTESIAN_POINT('Ctrl Pts',(20.4956513765258,-0.488675020866886,
25.6203605853346));
#42379=CARTESIAN_POINT('Ctrl Pts',(20.5062605794241,-0.333001167572864,
25.5504322045018));
#42380=CARTESIAN_POINT('Ctrl Pts',(20.5168697823223,-0.170092833567137,
25.5220965441889));
#42381=CARTESIAN_POINT('Ctrl Pts',(20.5274789852206,-0.00718449956139197,
25.4937608838759));
#42382=CARTESIAN_POINT('Ctrl Pts',(20.5380881881189,0.16295831515607,25.5070179440828));
#42383=CARTESIAN_POINT('Ctrl Pts',(20.5486973910171,0.319511493618563,25.5602451668845));
#42384=CARTESIAN_POINT('Ctrl Pts',(20.5593065939154,0.476064672081055,25.6134723896863));
#42385=CARTESIAN_POINT('Ctrl Pts',(20.5699157968137,0.619028214288567,25.706669775083));
#42386=CARTESIAN_POINT('Ctrl Pts',(20.580524999712,0.730904528410161,25.8284307100025));
#42387=CARTESIAN_POINT('Ctrl Pts',(20.5911342026102,0.842780842531747,25.9501916449219));
#42388=CARTESIAN_POINT('Ctrl Pts',(20.6017434055085,0.9235699285674,26.1005161293642));
#42389=CARTESIAN_POINT('Ctrl Pts',(20.6123526084068,0.96338384984444,26.2610056511606));
#42390=CARTESIAN_POINT('Ctrl Pts',(20.622961811305,1.00319777112148,26.421495172957));
#42391=CARTESIAN_POINT('Ctrl Pts',(20.6335710142033,1.00203652763991,26.5921497321076));
#42392=CARTESIAN_POINT('Ctrl Pts',(20.6441802171016,0.960042246295454,26.7520825782283));
#42393=CARTESIAN_POINT('Ctrl Pts',(20.6547894199999,0.918047964951002,26.912015424349));
#42394=CARTESIAN_POINT('Ctrl Pts',(20.6653986228981,0.835220645743676,27.0612265574397));
#42395=CARTESIAN_POINT('Ctrl Pts',(20.6760078257964,0.721697688751602,27.1814537306148));
#42396=CARTESIAN_POINT('Ctrl Pts',(20.6866170286947,0.608174731759521,27.3016809037899));
#42397=CARTESIAN_POINT('Ctrl Pts',(20.697226231593,0.463956136982686,27.3929241170493));
#42398=CARTESIAN_POINT('Ctrl Pts',(20.7078354344912,0.306693104628343,27.4440159323294));
#42399=CARTESIAN_POINT('Ctrl Pts',(20.7184446373895,0.149430072273992,27.4951077476095));
#42400=CARTESIAN_POINT('Ctrl Pts',(20.7290538402878,-0.0208773976578456,
27.5060481649102));
#42401=CARTESIAN_POINT('Ctrl Pts',(20.739663043186,-0.183385035721877,27.4754981648325));
#42402=CARTESIAN_POINT('Ctrl Pts',(20.7502722460843,-0.3458926737859,27.4449481647547));
#42403=CARTESIAN_POINT('Ctrl Pts',(20.7608814489826,-0.500600479982099,
27.3729077472986));
#42404=CARTESIAN_POINT('Ctrl Pts',(20.7714906518809,-0.628573458687896,
27.2681940822158));
#42405=CARTESIAN_POINT('Ctrl Pts',(20.7820998547791,-0.756546437393693,
27.1634804171331));
#42406=CARTESIAN_POINT('Ctrl Pts',(20.7927090576774,-0.857784588609095,
27.0260935044238));
#42407=CARTESIAN_POINT('Ctrl Pts',(20.8033182605757,-0.919897173965862,
26.8728484011604));
#42408=CARTESIAN_POINT('Ctrl Pts',(20.811489914505,-0.967738897520507,26.7548125824239));
#42409=CARTESIAN_POINT('Ctrl Pts',(20.8196615684344,-0.992368487932995,
26.6273685309256));
#42410=CARTESIAN_POINT('Ctrl Pts',(20.8278332223638,-0.992500311415872,
26.4999739716271));
#42411=CARTESIAN_POINT('Origin',(18.,0.,26.5));
#42412=CARTESIAN_POINT('',(21.3721667776362,-0.992404881561636,26.5000957579287));
#42413=CARTESIAN_POINT('',(21.2278332223638,-0.992448585256559,26.5000215597106));
#42414=CARTESIAN_POINT('',(18.,-0.9925,26.5));
#42415=CARTESIAN_POINT('Ctrl Pts',(21.3721667776362,-0.992404881561636,
26.5000957579287));
#42416=CARTESIAN_POINT('Ctrl Pts',(21.3655528552044,-0.99229338944025,26.6034157298074));
#42417=CARTESIAN_POINT('Ctrl Pts',(21.3589389327725,-0.976255401996959,
26.706744520868));
#42418=CARTESIAN_POINT('Ctrl Pts',(21.3523250103407,-0.944684059200136,
26.8047056191727));
#42419=CARTESIAN_POINT('Ctrl Pts',(21.3417394748401,-0.894154351085294,
26.9614916556679));
#42420=CARTESIAN_POINT('Ctrl Pts',(21.3311539393396,-0.803834751993709,
27.1045279320697));
#42421=CARTESIAN_POINT('Ctrl Pts',(21.3205684038391,-0.684188391208178,
27.2185914249928));
#42422=CARTESIAN_POINT('Ctrl Pts',(21.3099828683386,-0.564542030422647,
27.3326549179159));
#42423=CARTESIAN_POINT('Ctrl Pts',(21.299397332838,-0.415568907943175,27.4177456273603));
#42424=CARTESIAN_POINT('Ctrl Pts',(21.2888117973375,-0.256291739646409,
27.4599660179157));
#42425=CARTESIAN_POINT('Ctrl Pts',(21.2676407263364,0.0622625969471221,
27.5444067990263));
#42426=CARTESIAN_POINT('Ctrl Pts',(21.2464696553354,0.422033116809841,27.4573663045809));
#42427=CARTESIAN_POINT('Ctrl Pts',(21.2252985843343,0.666759555135708,27.2366491071053));
#42428=CARTESIAN_POINT('Ctrl Pts',(21.2147130488338,0.789122774298649,27.1262905083675));
#42429=CARTESIAN_POINT('Ctrl Pts',(21.2041275133332,0.882724973077366,26.9825127338723));
#42430=CARTESIAN_POINT('Ctrl Pts',(21.1935419778327,0.936999885799728,26.826371881063));
#42431=CARTESIAN_POINT('Ctrl Pts',(21.1829564423322,0.991274798522085,26.6702310282536));
#42432=CARTESIAN_POINT('Ctrl Pts',(21.1723709068316,1.00622242518808,26.5017270971303));
#42433=CARTESIAN_POINT('Ctrl Pts',(21.1617853713311,0.979495373543125,26.3391824037305));
#42434=CARTESIAN_POINT('Ctrl Pts',(21.1511998358306,0.952768321898173,26.1766377103308));
#42435=CARTESIAN_POINT('Ctrl Pts',(21.14061430033,0.884366591942281,26.0200522546547));
#42436=CARTESIAN_POINT('Ctrl Pts',(21.1300287648295,0.782932539033663,25.8897676576329));
#42437=CARTESIAN_POINT('Ctrl Pts',(21.119443229329,0.681498486125039,25.7594830606111));
#42438=CARTESIAN_POINT('Ctrl Pts',(21.1088576938284,0.54703211026369,25.6554993222437));
#42439=CARTESIAN_POINT('Ctrl Pts',(21.0982721583279,0.395737200458154,25.5897973573186));
#42440=CARTESIAN_POINT('Ctrl Pts',(21.0876866228274,0.244442290652617,25.5240953923935));
#42441=CARTESIAN_POINT('Ctrl Pts',(21.0771010873268,0.0763188469028976,
25.4966752009106));
#42442=CARTESIAN_POINT('Ctrl Pts',(21.0665155518263,-0.0880174092237496,
25.5112681203385));
#42443=CARTESIAN_POINT('Ctrl Pts',(21.0559300163258,-0.252353665350397,
25.5258610397663));
#42444=CARTESIAN_POINT('Ctrl Pts',(21.0453444808252,-0.412902733853967,
25.5824670701049));
#42445=CARTESIAN_POINT('Ctrl Pts',(21.0347589453247,-0.550228722711753,
25.673938060106));
#42446=CARTESIAN_POINT('Ctrl Pts',(21.0241734098242,-0.687554711569525,
25.7654090501072));
#42447=CARTESIAN_POINT('Ctrl Pts',(21.0135878743236,-0.801657620781514,
25.8917449997708));
#42448=CARTESIAN_POINT('Ctrl Pts',(21.0030023388231,-0.878451612019513,
26.0377656876369));
#42449=CARTESIAN_POINT('Ctrl Pts',(20.9927238184275,-0.953018326680525,
26.1795512986096));
#42450=CARTESIAN_POINT('Ctrl Pts',(20.9824452980318,-0.992408900464791,
26.3398963629713));
#42451=CARTESIAN_POINT('Ctrl Pts',(20.9721667776362,-0.992502482922401,
26.5000686713788));
#42452=CARTESIAN_POINT('Ctrl Pts',(20.8278332223638,-0.992500311415872,
26.4999739716271));
#42453=CARTESIAN_POINT('Ctrl Pts',(20.8302707713327,-0.992539633467141,
26.4619730382366));
#42454=CARTESIAN_POINT('Ctrl Pts',(20.8327083203016,-0.990399172499557,
26.4239765086048));
#42455=CARTESIAN_POINT('Ctrl Pts',(20.8351458692705,-0.986044805495746,
26.3862354076476));
#42456=CARTESIAN_POINT('Ctrl Pts',(20.8457550721688,-0.96709283217073,26.2219708112155));
#42457=CARTESIAN_POINT('Ctrl Pts',(20.856364275067,-0.906201866022573,26.0625449121689));
#42458=CARTESIAN_POINT('Ctrl Pts',(20.8669734779653,-0.810824473316787,
25.9274701628834));
#42459=CARTESIAN_POINT('Ctrl Pts',(20.8775826808636,-0.71544708061099,25.7923954135978));
#42460=CARTESIAN_POINT('Ctrl Pts',(20.8881918837618,-0.585583261347557,
25.6816718140735));
#42461=CARTESIAN_POINT('Ctrl Pts',(20.8988010866601,-0.437127306252613,
25.6088510455336));
#42462=CARTESIAN_POINT('Ctrl Pts',(20.9094102895584,-0.288671351157678,
25.5360302769936));
#42463=CARTESIAN_POINT('Ctrl Pts',(20.9200194924567,-0.121623260231236,
25.5011123394381));
#42464=CARTESIAN_POINT('Ctrl Pts',(20.930628695355,0.0435716189503967,25.5083709085851));
#42465=CARTESIAN_POINT('Ctrl Pts',(20.9412378982532,0.208766498132029,25.5156294777322));
#42466=CARTESIAN_POINT('Ctrl Pts',(20.9518471011515,0.372108165568853,25.5650645535818));
#42467=CARTESIAN_POINT('Ctrl Pts',(20.9624563040498,0.513604910215741,25.6506256790316));
#42468=CARTESIAN_POINT('Ctrl Pts',(20.973065506948,0.655101654862629,25.7361868044813));
#42469=CARTESIAN_POINT('Ctrl Pts',(20.9836747098463,0.774753476719582,25.8578739795312));
#42470=CARTESIAN_POINT('Ctrl Pts',(20.9942839127446,0.857915951702268,26.0007936691777));
#42471=CARTESIAN_POINT('Ctrl Pts',(21.0048931156429,0.941078426684954,26.1437133588242));
#42472=CARTESIAN_POINT('Ctrl Pts',(21.0155023185411,0.987751554793373,26.3078655630673));
#42473=CARTESIAN_POINT('Ctrl Pts',(21.0261115214394,0.992222919193793,26.4731593676527));
#42474=CARTESIAN_POINT('Ctrl Pts',(21.0367207243377,0.996694283594215,26.638453172238));
#42475=CARTESIAN_POINT('Ctrl Pts',(21.047329927236,0.958963884286633,26.8048885771656));
#42476=CARTESIAN_POINT('Ctrl Pts',(21.0579391301342,0.883649619768174,26.9520952227151));
#42477=CARTESIAN_POINT('Ctrl Pts',(21.0685483330325,0.808335355249724,27.0993018682646));
#42478=CARTESIAN_POINT('Ctrl Pts',(21.0791575359308,0.695437225520406,27.2272797544361));
#42479=CARTESIAN_POINT('Ctrl Pts',(21.089766738829,0.558773056873417,27.3203654135997));
#42480=CARTESIAN_POINT('Ctrl Pts',(21.1003759417273,0.422108888226428,27.4134510727633));
#42481=CARTESIAN_POINT('Ctrl Pts',(21.1109851446256,0.261678680661741,27.471644504919));
#42482=CARTESIAN_POINT('Ctrl Pts',(21.1215943475238,0.0971178058691354,
27.4878233003434));
#42483=CARTESIAN_POINT('Ctrl Pts',(21.1322035504221,-0.0674430689234892,
27.5040020957679));
#42484=CARTESIAN_POINT('Ctrl Pts',(21.1428127533204,-0.236134610944028,
27.4781662544611));
#42485=CARTESIAN_POINT('Ctrl Pts',(21.1534219562187,-0.38831032737321,27.413477876346));
#42486=CARTESIAN_POINT('Ctrl Pts',(21.1640311591169,-0.5404860438024,27.3487894982309));
#42487=CARTESIAN_POINT('Ctrl Pts',(21.1746403620152,-0.676145934640202,
27.2452485833074));
#42488=CARTESIAN_POINT('Ctrl Pts',(21.1852495649135,-0.778686316450531,
27.1155277097669));
#42489=CARTESIAN_POINT('Ctrl Pts',(21.1958587678118,-0.881226698260843,
26.9858068362265));
#42490=CARTESIAN_POINT('Ctrl Pts',(21.20646797071,-0.950647571043694,26.8299060040692));
#42491=CARTESIAN_POINT('Ctrl Pts',(21.2170771736083,-0.978452376321672,
26.6669062257339));
#42492=CARTESIAN_POINT('Ctrl Pts',(21.2206625231935,-0.987848930240464,
26.6118209197745));
#42493=CARTESIAN_POINT('Ctrl Pts',(21.2242478727786,-0.992492585617876,
26.5559248555442));
#42494=CARTESIAN_POINT('Ctrl Pts',(21.2278332223638,-0.992448585256559,
26.5000215597106));
#42495=CARTESIAN_POINT('Origin',(18.,0.,26.5));
#42496=CARTESIAN_POINT('',(21.7721667776362,-0.992176529618623,26.499357490987));
#42497=CARTESIAN_POINT('',(21.6278332223638,-0.992566083749324,26.4999845389628));
#42498=CARTESIAN_POINT('',(18.,-0.9925,26.5));
#42499=CARTESIAN_POINT('Ctrl Pts',(21.7721667776362,-0.992176529618623,
26.499357490987));
#42500=CARTESIAN_POINT('Ctrl Pts',(21.7698314833779,-0.992196569891483,
26.5357287700307));
#42501=CARTESIAN_POINT('Ctrl Pts',(21.7674961891197,-0.990235918585997,
26.5721393492544));
#42502=CARTESIAN_POINT('Ctrl Pts',(21.7651608948614,-0.986275112555324,
26.6083918497455));
#42503=CARTESIAN_POINT('Ctrl Pts',(21.7545753593609,-0.968321378159688,
26.772718948814));
#42504=CARTESIAN_POINT('Ctrl Pts',(21.7439898238604,-0.909271030322288,
26.9337980488715));
#42505=CARTESIAN_POINT('Ctrl Pts',(21.7334042883598,-0.814709943053242,
27.0687424021946));
#42506=CARTESIAN_POINT('Ctrl Pts',(21.7122332173588,-0.62558776851514,27.3386311088407));
#42507=CARTESIAN_POINT('Ctrl Pts',(21.6910621463577,-0.294422636250437,
27.5039808285492));
#42508=CARTESIAN_POINT('Ctrl Pts',(21.6698910753566,0.0349494571674246,
27.4929746959553));
#42509=CARTESIAN_POINT('Ctrl Pts',(21.6593055398561,0.199635503876346,27.4874716296583));
#42510=CARTESIAN_POINT('Ctrl Pts',(21.6487200043556,0.363873290873557,27.4378796002858));
#42511=CARTESIAN_POINT('Ctrl Pts',(21.6381344688551,0.506012333303722,27.353486326359));
#42512=CARTESIAN_POINT('Ctrl Pts',(21.6275489333545,0.648151375733887,27.2690930524323));
#42513=CARTESIAN_POINT('Ctrl Pts',(21.616963397854,0.768191673597007,27.1498985339513));
#42514=CARTESIAN_POINT('Ctrl Pts',(21.6063778623534,0.85252856782575,27.0083980006877));
#42515=CARTESIAN_POINT('Ctrl Pts',(21.5957923268529,0.936865462054492,26.866897467424));
#42516=CARTESIAN_POINT('Ctrl Pts',(21.5852067913524,0.985498952648858,26.7030909193777));
#42517=CARTESIAN_POINT('Ctrl Pts',(21.5746212558519,0.9919249873757,26.5381010730589));
#42518=CARTESIAN_POINT('Ctrl Pts',(21.5640357203513,0.998351022102542,26.3731112267402));
#42519=CARTESIAN_POINT('Ctrl Pts',(21.5534501848508,0.962569600961857,26.2069380821491));
#42520=CARTESIAN_POINT('Ctrl Pts',(21.5428646493503,0.889246785300691,26.0591860512608));
#42521=CARTESIAN_POINT('Ctrl Pts',(21.5322791138497,0.815923969639525,25.9114340203725));
#42522=CARTESIAN_POINT('Ctrl Pts',(21.5216935783492,0.705059759457878,25.7821031031871));
#42523=CARTESIAN_POINT('Ctrl Pts',(21.5111080428487,0.570010756288525,25.6873343049563));
#42524=CARTESIAN_POINT('Ctrl Pts',(21.5005225073481,0.434961753119187,25.5925655067255));
#42525=CARTESIAN_POINT('Ctrl Pts',(21.4899369718476,0.275727956962149,25.5323588274492));
#42526=CARTESIAN_POINT('Ctrl Pts',(21.4793514363471,0.111776496367536,25.5137769062234));
#42527=CARTESIAN_POINT('Ctrl Pts',(21.4687659008465,-0.0521749642271047,
25.4951949849977));
#42528=CARTESIAN_POINT('Ctrl Pts',(21.458180365346,-0.220844089259322,25.5182378218223));
#42529=CARTESIAN_POINT('Ctrl Pts',(21.4475948298455,-0.373676910774448,
25.580378686339));
#42530=CARTESIAN_POINT('Ctrl Pts',(21.4370092943449,-0.526509732289548,
25.6425195508557));
#42531=CARTESIAN_POINT('Ctrl Pts',(21.4264237588444,-0.663506250287563,
25.7437584430643));
#42532=CARTESIAN_POINT('Ctrl Pts',(21.4158382233439,-0.768036281504167,
25.8713529982065));
#42533=CARTESIAN_POINT('Ctrl Pts',(21.4052526878434,-0.872566312720771,
25.9989475533487));
#42534=CARTESIAN_POINT('Ctrl Pts',(21.3946671523428,-0.944629857155963,
26.1528977714245));
#42535=CARTESIAN_POINT('Ctrl Pts',(21.3840816168423,-0.975291720804518,
26.3151407787567));
#42536=CARTESIAN_POINT('Ctrl Pts',(21.3801100037736,-0.98679582075023,26.376013131241));
#42537=CARTESIAN_POINT('Ctrl Pts',(21.3761383907049,-0.992471831782313,
26.4380528545232));
#42538=CARTESIAN_POINT('Ctrl Pts',(21.3721667776362,-0.992404881561636,
26.5000957579287));
#42539=CARTESIAN_POINT('Ctrl Pts',(21.2278332223638,-0.992448585256559,
26.5000215597106));
#42540=CARTESIAN_POINT('Ctrl Pts',(21.2348570756769,-0.992362386665246,
26.3905046101561));
#42541=CARTESIAN_POINT('Ctrl Pts',(21.24188092899,-0.974285674510598,26.2809599068025));
#42542=CARTESIAN_POINT('Ctrl Pts',(21.2489047823031,-0.938708977451642,
26.1774287728734));
#42543=CARTESIAN_POINT('Ctrl Pts',(21.2595139852014,-0.884972035530529,
26.0210498228614));
#42544=CARTESIAN_POINT('Ctrl Pts',(21.2701231880997,-0.791309413915201,
25.8783906473505));
#42545=CARTESIAN_POINT('Ctrl Pts',(21.2807323909979,-0.669184666862485,
25.7669115861273));
#42546=CARTESIAN_POINT('Ctrl Pts',(21.2913415938962,-0.547059919809769,
25.6554325249041));
#42547=CARTESIAN_POINT('Ctrl Pts',(21.3019507967945,-0.396473047319665,
25.5751335779686));
#42548=CARTESIAN_POINT('Ctrl Pts',(21.3125599996928,-0.235854675755011,
25.5358426928956));
#42549=CARTESIAN_POINT('Ctrl Pts',(21.323169202591,-0.075236304190348,25.4965518078227));
#42550=CARTESIAN_POINT('Ctrl Pts',(21.3337784054893,0.0954135664488655,
25.4982689846123));
#42551=CARTESIAN_POINT('Ctrl Pts',(21.3443876083876,0.255208759614769,25.5407840545872));
#42552=CARTESIAN_POINT('Ctrl Pts',(21.3549968112858,0.415003952780655,25.5832991245621));
#42553=CARTESIAN_POINT('Ctrl Pts',(21.3656060141841,0.563944468473233,25.6666120877223));
#42554=CARTESIAN_POINT('Ctrl Pts',(21.3762152170824,0.683801181207488,25.7805261050618));
#42555=CARTESIAN_POINT('Ctrl Pts',(21.3868244199807,0.803657893941749,25.8944401224014));
#42556=CARTESIAN_POINT('Ctrl Pts',(21.3974336228789,0.894430803717683,26.0389551939203));
#42557=CARTESIAN_POINT('Ctrl Pts',(21.4080428257772,0.945010033848943,26.1963838330341));
#42558=CARTESIAN_POINT('Ctrl Pts',(21.4186520286755,0.995589263980203,26.3538124721479));
#42559=CARTESIAN_POINT('Ctrl Pts',(21.4292612315738,1.00597481446679,26.5241546788566));
#42560=CARTESIAN_POINT('Ctrl Pts',(21.439870434472,0.974895577160786,26.6865619322118));
#42561=CARTESIAN_POINT('Ctrl Pts',(21.4504796373703,0.943816339854783,26.848969185567));
#42562=CARTESIAN_POINT('Ctrl Pts',(21.4610888402686,0.871272314756188,27.0034414855686));
#42563=CARTESIAN_POINT('Ctrl Pts',(21.4716980431668,0.766142309156365,27.131072660665));
#42564=CARTESIAN_POINT('Ctrl Pts',(21.4823072460651,0.661012303556554,27.2587038357614));
#42565=CARTESIAN_POINT('Ctrl Pts',(21.4929164489634,0.523296317455523,27.3594938859524));
#42566=CARTESIAN_POINT('Ctrl Pts',(21.5035256518616,0.369849683871657,27.4211069168442));
#42567=CARTESIAN_POINT('Ctrl Pts',(21.5141348547599,0.216403050287774,27.482719947736));
#42568=CARTESIAN_POINT('Ctrl Pts',(21.5247440576582,0.047225769221051,27.5051559593285));
#42569=CARTESIAN_POINT('Ctrl Pts',(21.5353532605565,-0.116976215942728,
27.485668963609));
#42570=CARTESIAN_POINT('Ctrl Pts',(21.5459624634548,-0.281178201106498,
27.4661819678894));
#42571=CARTESIAN_POINT('Ctrl Pts',(21.556571666353,-0.440404890367325,27.4047719648578));
#42572=CARTESIAN_POINT('Ctrl Pts',(21.5671808692513,-0.575168213030661,
27.3089550467346));
#42573=CARTESIAN_POINT('Ctrl Pts',(21.5777900721496,-0.709931535694004,
27.2131381286113));
#42574=CARTESIAN_POINT('Ctrl Pts',(21.5883992750478,-0.820231491759853,
27.0829142953965));
#42575=CARTESIAN_POINT('Ctrl Pts',(21.5990084779461,-0.89256825056919,26.9342219006385));
#42576=CARTESIAN_POINT('Ctrl Pts',(21.6086167260854,-0.958080196649587,
26.7995583034814));
#42577=CARTESIAN_POINT('Ctrl Pts',(21.6182249742246,-0.992454502819291,
26.649746682434));
#42578=CARTESIAN_POINT('Ctrl Pts',(21.6278332223638,-0.992566083749324,
26.4999845389628));
#42579=CARTESIAN_POINT('Origin',(18.,0.,26.5));
#42580=CARTESIAN_POINT('',(22.1721667776362,-0.993165579585467,26.5002657239842));
#42581=CARTESIAN_POINT('',(22.0278332223638,-0.99241508312295,26.500004132563));
#42582=CARTESIAN_POINT('',(18.,-0.9925,26.5));
#42583=CARTESIAN_POINT('Ctrl Pts',(22.1721667776362,-0.993165579585467,
26.5002657239842));
#42584=CARTESIAN_POINT('Ctrl Pts',(22.1529390405505,-0.990983883449612,
26.7991898919088));
#42585=CARTESIAN_POINT('Ctrl Pts',(22.1337113034647,-0.848467038466999,
27.0965311454012));
#42586=CARTESIAN_POINT('Ctrl Pts',(22.114483566379,-0.613318510459232,27.2817036625806));
#42587=CARTESIAN_POINT('Ctrl Pts',(22.1038980308785,-0.483861097970969,
27.3836475494553));
#42588=CARTESIAN_POINT('Ctrl Pts',(22.0933124953779,-0.326328096839694,
27.4515943934557));
#42589=CARTESIAN_POINT('Ctrl Pts',(22.0827269598774,-0.163258892301617,
27.4786899022784));
#42590=CARTESIAN_POINT('Ctrl Pts',(22.0721414243769,-0.000189687763549218,
27.5057854111011));
#42591=CARTESIAN_POINT('Ctrl Pts',(22.0615558888763,0.168415720181321,27.4920295847462));
#42592=CARTESIAN_POINT('Ctrl Pts',(22.0509703533758,0.32410190589134,27.4382065021411));
#42593=CARTESIAN_POINT('Ctrl Pts',(22.0403848178753,0.47978809160136,27.3843834195361));
#42594=CARTESIAN_POINT('Ctrl Pts',(22.0297992823747,0.622555055076529,27.2904930806809));
#42595=CARTESIAN_POINT('Ctrl Pts',(22.0192137468742,0.7338151263775,27.1684925075482));
#42596=CARTESIAN_POINT('Ctrl Pts',(22.0086282113737,0.845075197678483,27.0464919344155));
#42597=CARTESIAN_POINT('Ctrl Pts',(21.9980426758731,0.924828376805261,26.8963811270054));
#42598=CARTESIAN_POINT('Ctrl Pts',(21.9874571403726,0.964005726421413,26.736156181366));
#42599=CARTESIAN_POINT('Ctrl Pts',(21.9768716048721,1.00318307603756,26.5759312357267));
#42600=CARTESIAN_POINT('Ctrl Pts',(21.9662860693715,1.00178459614309,26.4055921518581));
#42601=CARTESIAN_POINT('Ctrl Pts',(21.955700533871,0.959618079499461,26.2460887247811));
#42602=CARTESIAN_POINT('Ctrl Pts',(21.9451149983705,0.917451562855824,26.0865852977042));
#42603=CARTESIAN_POINT('Ctrl Pts',(21.93452946287,0.83451700946301,25.9379175274189));
#42604=CARTESIAN_POINT('Ctrl Pts',(21.9239439273694,0.721145618717982,25.818033012205));
#42605=CARTESIAN_POINT('Ctrl Pts',(21.9133583918689,0.607774227972941,25.698148496991));
#42606=CARTESIAN_POINT('Ctrl Pts',(21.9027728563683,0.463965999875679,25.6070472368483));
#42607=CARTESIAN_POINT('Ctrl Pts',(21.8921873208678,0.307064068355902,25.5560458421564));
#42608=CARTESIAN_POINT('Ctrl Pts',(21.8816017853673,0.150162136836144,25.5050444474645));
#42609=CARTESIAN_POINT('Ctrl Pts',(21.8710162498668,-0.0198334981061266,
25.4941429182234));
#42610=CARTESIAN_POINT('Ctrl Pts',(21.8604307143662,-0.181994958540001,
25.5243183830589));
#42611=CARTESIAN_POINT('Ctrl Pts',(21.8498451788657,-0.344156418973875,
25.5544938478944));
#42612=CARTESIAN_POINT('Ctrl Pts',(21.8392596433651,-0.498483704899352,
25.6257463068065));
#42613=CARTESIAN_POINT('Ctrl Pts',(21.8286741078646,-0.626502697534403,
25.7300251677291));
#42614=CARTESIAN_POINT('Ctrl Pts',(21.8180885723641,-0.754521690169455,
25.8343040286516));
#42615=CARTESIAN_POINT('Ctrl Pts',(21.8075030368636,-0.856232389514079,
25.9716092915846));
#42616=CARTESIAN_POINT('Ctrl Pts',(21.7969175013631,-0.918659178709456,
26.1240494720909));
#42617=CARTESIAN_POINT('Ctrl Pts',(21.7886672601208,-0.967313880289416,
26.2428595468509));
#42618=CARTESIAN_POINT('Ctrl Pts',(21.7804170188785,-0.992105730367064,
26.3708632657564));
#42619=CARTESIAN_POINT('Ctrl Pts',(21.7721667776362,-0.992176529618623,
26.499357490987));
#42620=CARTESIAN_POINT('Ctrl Pts',(21.6278332223638,-0.992566083749324,
26.4999845389628));
#42621=CARTESIAN_POINT('Ctrl Pts',(21.6288341771228,-0.992577707872818,
26.4843828259284));
#42622=CARTESIAN_POINT('Ctrl Pts',(21.6298351318819,-0.992217486624713,
26.4687816498625));
#42623=CARTESIAN_POINT('Ctrl Pts',(21.6308360866409,-0.991481886769432,
26.453198193129));
#42624=CARTESIAN_POINT('Ctrl Pts',(21.6414452895392,-0.983685202607518,
26.2880278366786));
#42625=CARTESIAN_POINT('Ctrl Pts',(21.6520544924375,-0.93371827273086,26.1248480800787));
#42626=CARTESIAN_POINT('Ctrl Pts',(21.6626636953357,-0.847696648912507,
25.9836308177856));
#42627=CARTESIAN_POINT('Ctrl Pts',(21.673272898234,-0.761675025094154,25.8424135554925));
#42628=CARTESIAN_POINT('Ctrl Pts',(21.6838821011323,-0.639598707334108,
25.7231587875063));
#42629=CARTESIAN_POINT('Ctrl Pts',(21.6944913040306,-0.496408858584897,
25.6404623416995));
#42630=CARTESIAN_POINT('Ctrl Pts',(21.7051005069288,-0.353219009835685,
25.5577658958927));
#42631=CARTESIAN_POINT('Ctrl Pts',(21.7157097098271,-0.188915630097313,
25.5116277722654));
#42632=CARTESIAN_POINT('Ctrl Pts',(21.7263189127254,-0.0236081362932755,
25.5076949073904));
#42633=CARTESIAN_POINT('Ctrl Pts',(21.7369281156237,0.141699357510753,25.5037620425154));
#42634=CARTESIAN_POINT('Ctrl Pts',(21.7475373185219,0.30801096538044,25.5420344363926));
#42635=CARTESIAN_POINT('Ctrl Pts',(21.7581465214202,0.454971479363318,25.6178278547334));
#42636=CARTESIAN_POINT('Ctrl Pts',(21.7687557243185,0.601931993346212,25.6936212730742));
#42637=CARTESIAN_POINT('Ctrl Pts',(21.7793649272167,0.729541413442286,25.8069357158786));
#42638=CARTESIAN_POINT('Ctrl Pts',(21.789974130115,0.822181369316348,25.9439024034692));
#42639=CARTESIAN_POINT('Ctrl Pts',(21.8005833330133,0.91482132519041,26.0808690910598));
#42640=CARTESIAN_POINT('Ctrl Pts',(21.8111925359116,0.972491816842456,26.2414880234368));
#42641=CARTESIAN_POINT('Ctrl Pts',(21.8218017388098,0.988134438275843,26.4061007305058));
#42642=CARTESIAN_POINT('Ctrl Pts',(21.8324109417081,1.00377705970923,26.5707134375748));
#42643=CARTESIAN_POINT('Ctrl Pts',(21.8430201446064,0.977391810923953,26.7393199193359));
#42644=CARTESIAN_POINT('Ctrl Pts',(21.8536293475047,0.912208034915269,26.8912840936638));
#42645=CARTESIAN_POINT('Ctrl Pts',(21.8642385504029,0.847024258906589,27.0432482679916));
#42646=CARTESIAN_POINT('Ctrl Pts',(21.8748477533012,0.743041955674507,27.1785701348863));
#42647=CARTESIAN_POINT('Ctrl Pts',(21.8854569561995,0.612987725801971,27.2806873823333));
#42648=CARTESIAN_POINT('Ctrl Pts',(21.8960661590977,0.48293349592942,27.3828046297803));
#42649=CARTESIAN_POINT('Ctrl Pts',(21.906675361996,0.326807339416416,27.4517172577797));
#42650=CARTESIAN_POINT('Ctrl Pts',(21.9172845648943,0.163717846597389,27.4789909129424));
#42651=CARTESIAN_POINT('Ctrl Pts',(21.9278937677926,0.000628353778372309,
27.5062645681051));
#42652=CARTESIAN_POINT('Ctrl Pts',(21.9385029706908,-0.169424475346632,
27.491899250431));
#42653=CARTESIAN_POINT('Ctrl Pts',(21.9491121735891,-0.325627537326366,
27.4376531596774));
#42654=CARTESIAN_POINT('Ctrl Pts',(21.9597213764874,-0.481830599306091,
27.3834070689238));
#42655=CARTESIAN_POINT('Ctrl Pts',(21.9703305793856,-0.624183894140539,
27.2892802050905));
#42656=CARTESIAN_POINT('Ctrl Pts',(21.9809397822839,-0.735264519386526,
27.1667929419614));
#42657=CARTESIAN_POINT('Ctrl Pts',(21.9915489851822,-0.84634514463252,27.0443056788323));
#42658=CARTESIAN_POINT('Ctrl Pts',(22.0021581880805,-0.926153100290073,
26.8934580164074));
#42659=CARTESIAN_POINT('Ctrl Pts',(22.0127673909787,-0.964920532181839,
26.7327124996475));
#42660=CARTESIAN_POINT('Ctrl Pts',(22.0177893347738,-0.983271379639895,
26.6566224334841));
#42661=CARTESIAN_POINT('Ctrl Pts',(22.0228112785688,-0.992426394010815,
26.5783145833347));
#42662=CARTESIAN_POINT('Ctrl Pts',(22.0278332223638,-0.99241508312295,26.500004132563));
#42663=CARTESIAN_POINT('Origin',(18.,0.,26.5));
#42664=CARTESIAN_POINT('',(22.5721667776362,-0.992204861021737,26.5000685690985));
#42665=CARTESIAN_POINT('',(22.4278332223638,-0.992581696356067,26.5000071712556));
#42666=CARTESIAN_POINT('',(18.,-0.9925,26.5));
#42667=CARTESIAN_POINT('Ctrl Pts',(22.5721667776362,-0.992204861021737,
26.5000685690985));
#42668=CARTESIAN_POINT('Ctrl Pts',(22.5678032042246,-0.992827066651901,
26.5679305324631));
#42669=CARTESIAN_POINT('Ctrl Pts',(22.563439630813,-0.986484995098284,26.6357983943371));
#42670=CARTESIAN_POINT('Ctrl Pts',(22.5590760574013,-0.972771803344622,
26.7023245659368));
#42671=CARTESIAN_POINT('Ctrl Pts',(22.5484905219008,-0.93950515135077,26.8637095329703));
#42672=CARTESIAN_POINT('Ctrl Pts',(22.5379049864003,-0.862859993839026,
27.0171987504581));
#42673=CARTESIAN_POINT('Ctrl Pts',(22.5273194508997,-0.755650710103984,
27.1430236349129));
#42674=CARTESIAN_POINT('Ctrl Pts',(22.5167339153992,-0.648441426368947,
27.2688485193677));
#42675=CARTESIAN_POINT('Ctrl Pts',(22.5061483798987,-0.510668016410612,
27.3670090707894));
#42676=CARTESIAN_POINT('Ctrl Pts',(22.4955628443982,-0.356945922593113,
27.4262089906746));
#42677=CARTESIAN_POINT('Ctrl Pts',(22.4849773088976,-0.203223828775614,
27.4854089105597));
#42678=CARTESIAN_POINT('Ctrl Pts',(22.4743917733971,-0.033553051098976,
27.5056481989083));
#42679=CARTESIAN_POINT('Ctrl Pts',(22.4638062378966,0.130148147127243,27.4840875632523));
#42680=CARTESIAN_POINT('Ctrl Pts',(22.453220702396,0.293849345353462,27.4625269275963));
#42681=CARTESIAN_POINT('Ctrl Pts',(22.4426351668955,0.451580964129261,27.3991663679356));
#42682=CARTESIAN_POINT('Ctrl Pts',(22.4320496313949,0.584809674211439,27.301919215083));
#42683=CARTESIAN_POINT('Ctrl Pts',(22.4214640958944,0.718038384293619,27.2046720622305));
#42684=CARTESIAN_POINT('Ctrl Pts',(22.4108785603939,0.826764185682209,27.0735383161861));
#42685=CARTESIAN_POINT('Ctrl Pts',(22.4002930248934,0.89733657369241,26.9244112011946));
#42686=CARTESIAN_POINT('Ctrl Pts',(22.3897074893929,0.967908961702614,26.7752840862031));
#42687=CARTESIAN_POINT('Ctrl Pts',(22.3791219538923,1.00032793633442,26.6081636022645));
#42688=CARTESIAN_POINT('Ctrl Pts',(22.3685364183917,0.990923755700695,26.4434306953693));
#42689=CARTESIAN_POINT('Ctrl Pts',(22.3579508828912,0.981519575066965,26.278697788474));
#42690=CARTESIAN_POINT('Ctrl Pts',(22.3473653473907,0.930292239167682,26.1163524586221));
#42691=CARTESIAN_POINT('Ctrl Pts',(22.3367798118902,0.843207081642137,25.9762256099674));
#42692=CARTESIAN_POINT('Ctrl Pts',(22.3261942763896,0.756121924116602,25.8360987613127));
#42693=CARTESIAN_POINT('Ctrl Pts',(22.3156087408891,0.633178944964809,25.7181903938551));
#42694=CARTESIAN_POINT('Ctrl Pts',(22.3050232053886,0.489748677103296,25.6367369949742));
#42695=CARTESIAN_POINT('Ctrl Pts',(22.294437669888,0.346318409241783,25.5552835960932));
#42696=CARTESIAN_POINT('Ctrl Pts',(22.2838521343875,0.182400852670543,25.5102851657888));
#42697=CARTESIAN_POINT('Ctrl Pts',(22.273266598887,0.0173094984056945,25.5074944566334));
#42698=CARTESIAN_POINT('Ctrl Pts',(22.2626810633864,-0.147781855859145,
25.5047037474779));
#42699=CARTESIAN_POINT('Ctrl Pts',(22.2520955278859,-0.314047007817625,
25.5441207594714));
#42700=CARTESIAN_POINT('Ctrl Pts',(22.2415099923854,-0.460033215139826,
25.6204302602804));
#42701=CARTESIAN_POINT('Ctrl Pts',(22.2309244568849,-0.606019422462045,
25.6967397610894));
#42702=CARTESIAN_POINT('Ctrl Pts',(22.2203389213843,-0.73172668514799,25.809941750714));
#42703=CARTESIAN_POINT('Ctrl Pts',(22.2097533858838,-0.823920078142038,
25.9471500243541));
#42704=CARTESIAN_POINT('Ctrl Pts',(22.1991678503832,-0.916113471136081,
26.0843582979942));
#42705=CARTESIAN_POINT('Ctrl Pts',(22.1885823148827,-0.97479299443821,26.2455728556497));
#42706=CARTESIAN_POINT('Ctrl Pts',(22.1779967793822,-0.98947726490555,26.4096952182945));
#42707=CARTESIAN_POINT('Ctrl Pts',(22.1760534454669,-0.992173060580657,
26.4398254420867));
#42708=CARTESIAN_POINT('Ctrl Pts',(22.1741101115516,-0.993386082085311,
26.4700536677735));
#42709=CARTESIAN_POINT('Ctrl Pts',(22.1721667776362,-0.993165579585467,
26.5002657239842));
#42710=CARTESIAN_POINT('Ctrl Pts',(22.0278332223638,-0.99241508312295,26.500004132563));
#42711=CARTESIAN_POINT('Ctrl Pts',(22.0334204814671,-0.992402498979485,
26.4128783508313));
#42712=CARTESIAN_POINT('Ctrl Pts',(22.0390077405703,-0.981043747310354,
26.3257493500237));
#42713=CARTESIAN_POINT('Ctrl Pts',(22.0445949996735,-0.958379464788188,
26.2416677674185));
#42714=CARTESIAN_POINT('Ctrl Pts',(22.0552042025718,-0.915344057376794,
26.0820119230443));
#42715=CARTESIAN_POINT('Ctrl Pts',(22.0658134054701,-0.831546334428029,
25.9333436053908));
#42716=CARTESIAN_POINT('Ctrl Pts',(22.0764226083684,-0.717242465660984,
25.8138586250846));
#42717=CARTESIAN_POINT('Ctrl Pts',(22.0870318112667,-0.602938596893939,
25.6943736447783));
#42718=CARTESIAN_POINT('Ctrl Pts',(22.0976410141649,-0.458128582308614,
25.6040720018193));
#42719=CARTESIAN_POINT('Ctrl Pts',(22.1082502170632,-0.300536007157066,
25.5540058936123));
#42720=CARTESIAN_POINT('Ctrl Pts',(22.1188594199615,-0.14294343200551,25.5039397854052));
#42721=CARTESIAN_POINT('Ctrl Pts',(22.1294686228597,0.0274317037122691,
25.4941092119501));
#42722=CARTESIAN_POINT('Ctrl Pts',(22.140077825758,0.189736848801019,25.525717356654));
#42723=CARTESIAN_POINT('Ctrl Pts',(22.1506870286563,0.35204199388976,25.5573255013578));
#42724=CARTESIAN_POINT('Ctrl Pts',(22.1612962315546,0.506277148349473,25.6303723642206));
#42725=CARTESIAN_POINT('Ctrl Pts',(22.1719054344528,0.633565165342219,25.7359175946384));
#42726=CARTESIAN_POINT('Ctrl Pts',(22.1825146373511,0.760853182334965,25.8414628250562));
#42727=CARTESIAN_POINT('Ctrl Pts',(22.1931238402494,0.861194061860744,25.9795064230291));
#42728=CARTESIAN_POINT('Ctrl Pts',(22.2037330431476,0.922306884415235,26.1331529584711));
#42729=CARTESIAN_POINT('Ctrl Pts',(22.2143422460459,0.983419706969726,26.2867994939131));
#42730=CARTESIAN_POINT('Ctrl Pts',(22.2249514489442,1.00530447255293,26.4560489668241));
#42731=CARTESIAN_POINT('Ctrl Pts',(22.2355606518425,0.985282661245862,26.6201865981153));
#42732=CARTESIAN_POINT('Ctrl Pts',(22.2461698547407,0.965260849938794,26.7843242294065));
#42733=CARTESIAN_POINT('Ctrl Pts',(22.256779057639,0.903332461741456,26.9433500190778));
#42734=CARTESIAN_POINT('Ctrl Pts',(22.2673882605373,0.807077035064093,27.0778004849344));
#42735=CARTESIAN_POINT('Ctrl Pts',(22.2779974634355,0.710821608386725,27.212250950791));
#42736=CARTESIAN_POINT('Ctrl Pts',(22.2886066663338,0.58023914322933,27.3221260928329));
#42737=CARTESIAN_POINT('Ctrl Pts',(22.2992158692321,0.431311886816099,27.393978074233));
#42738=CARTESIAN_POINT('Ctrl Pts',(22.3098250721304,0.282384630402886,27.4658300556332));
#42739=CARTESIAN_POINT('Ctrl Pts',(22.3204342750286,0.115112582733842,27.4996588763916));
#42740=CARTESIAN_POINT('Ctrl Pts',(22.3310434779269,-0.0500314981042523,
27.4913241599576));
#42741=CARTESIAN_POINT('Ctrl Pts',(22.3416526808252,-0.215175578942356,
27.4829894435237));
#42742=CARTESIAN_POINT('Ctrl Pts',(22.3522618837235,-0.37819169294951,27.4324911898973));
#42743=CARTESIAN_POINT('Ctrl Pts',(22.3628710866217,-0.519127974211338,
27.3460099806205));
#42744=CARTESIAN_POINT('Ctrl Pts',(22.37348028952,-0.660064255473166,27.2595287713437));
#42745=CARTESIAN_POINT('Ctrl Pts',(22.3840894924183,-0.778920703989667,
27.1370646064163));
#42746=CARTESIAN_POINT('Ctrl Pts',(22.3946986953166,-0.861150242999118,
26.993606118176));
#42747=CARTESIAN_POINT('Ctrl Pts',(22.4053078982148,-0.943379782008568,
26.8501476299357));
#42748=CARTESIAN_POINT('Ctrl Pts',(22.4159171011131,-0.988982411510966,
26.6856948183825));
#42749=CARTESIAN_POINT('Ctrl Pts',(22.4265263040114,-0.992376735122795,
26.5203753896963));
#42750=CARTESIAN_POINT('Ctrl Pts',(22.4269619434622,-0.992516114234338,
26.5135869753534));
#42751=CARTESIAN_POINT('Ctrl Pts',(22.427397582913,-0.992584325009407,26.5067970997886));
#42752=CARTESIAN_POINT('Ctrl Pts',(22.4278332223638,-0.992581696356067,
26.5000071712556));
#42753=CARTESIAN_POINT('Origin',(18.,0.,26.5));
#42754=CARTESIAN_POINT('',(22.9721667776362,-0.992215768961308,26.5005746468071));
#42755=CARTESIAN_POINT('',(22.8278332223638,-0.99243012155925,26.4999841927042));
#42756=CARTESIAN_POINT('',(18.,-0.9925,26.5));
#42757=CARTESIAN_POINT('Ctrl Pts',(22.9721667776362,-0.992215768961308,
26.5005746468071));
#42758=CARTESIAN_POINT('Ctrl Pts',(22.9720818323982,-0.992214140284424,
26.5019013181872));
#42759=CARTESIAN_POINT('Ctrl Pts',(22.9719968871601,-0.992209860101849,
26.5032279082689));
#42760=CARTESIAN_POINT('Ctrl Pts',(22.9719119419221,-0.992202926891772,
26.5045544049738));
#42761=CARTESIAN_POINT('Ctrl Pts',(22.9613264064216,-0.9913389380079,26.669857113936));
#42762=CARTESIAN_POINT('Ctrl Pts',(22.950740870921,-0.949275696035103,26.8337097612191));
#42763=CARTESIAN_POINT('Ctrl Pts',(22.9401553354205,-0.869906177042421,
26.9780551528911));
#42764=CARTESIAN_POINT('Ctrl Pts',(22.92956979992,-0.790536658049743,27.122400544563));
#42765=CARTESIAN_POINT('Ctrl Pts',(22.9189842644194,-0.673860862037187,
27.2472386806237));
#42766=CARTESIAN_POINT('Ctrl Pts',(22.9083987289189,-0.534806228703558,
27.3362709908208));
#42767=CARTESIAN_POINT('Ctrl Pts',(22.8978131934184,-0.395751595369929,
27.425303301018));
#42768=CARTESIAN_POINT('Ctrl Pts',(22.8872276579178,-0.234318124715232,
27.4785297853516));
#42769=CARTESIAN_POINT('Ctrl Pts',(22.8766421224173,-0.06977610285199,27.4900545833647));
#42770=CARTESIAN_POINT('Ctrl Pts',(22.8660565869168,0.0947659190112521,
27.5015793813778));
#42771=CARTESIAN_POINT('Ctrl Pts',(22.8554710514162,0.262416492083034,27.4714024930703));
#42772=CARTESIAN_POINT('Ctrl Pts',(22.8448855159157,0.412494903395397,27.4028763751801));
#42773=CARTESIAN_POINT('Ctrl Pts',(22.8342999804152,0.56257331470776,27.3343502572899));
#42774=CARTESIAN_POINT('Ctrl Pts',(22.8237144449146,0.695079564260698,27.2274749098169));
#42775=CARTESIAN_POINT('Ctrl Pts',(22.8131289094141,0.794071068217059,27.0954671396971));
#42776=CARTESIAN_POINT('Ctrl Pts',(22.8025433739136,0.89306257217342,26.9634593695772));
#42777=CARTESIAN_POINT('Ctrl Pts',(22.791957838413,0.958539330533199,26.8063191768106));
#42778=CARTESIAN_POINT('Ctrl Pts',(22.7813723029125,0.982279771970663,26.6430532899404));
#42779=CARTESIAN_POINT('Ctrl Pts',(22.770786767412,1.00602021340813,26.4797874030702));
#42780=CARTESIAN_POINT('Ctrl Pts',(22.7602012319115,0.988024337923265,26.3103958220965));
#42781=CARTESIAN_POINT('Ctrl Pts',(22.7496156964109,0.930867274580648,26.1556703618835));
#42782=CARTESIAN_POINT('Ctrl Pts',(22.7390301609104,0.87371021123803,26.0009449016704));
#42783=CARTESIAN_POINT('Ctrl Pts',(22.7284446254099,0.777391960037676,25.8608855622181));
#42784=CARTESIAN_POINT('Ctrl Pts',(22.7178590899093,0.652970567212468,25.7523394415226));
#42785=CARTESIAN_POINT('Ctrl Pts',(22.7072735544088,0.528549174387274,25.6437933208272));
#42786=CARTESIAN_POINT('Ctrl Pts',(22.6966880189083,0.376024639937221,25.5667604188887));
#42787=CARTESIAN_POINT('Ctrl Pts',(22.6861024834077,0.21522463077963,25.5310047242798));
#42788=CARTESIAN_POINT('Ctrl Pts',(22.6755169479072,0.0544246216220219,
25.4952490296709));
#42789=CARTESIAN_POINT('Ctrl Pts',(22.6649314124067,-0.114650862243145,
25.5007705423917));
#42790=CARTESIAN_POINT('Ctrl Pts',(22.6543458769061,-0.273577064688015,
25.54624794605));
#42791=CARTESIAN_POINT('Ctrl Pts',(22.6437603414056,-0.432503267132867,
25.5917253497082));
#42792=CARTESIAN_POINT('Ctrl Pts',(22.6331748059051,-0.581280188157419,
25.6771586443039));
#42793=CARTESIAN_POINT('Ctrl Pts',(22.6225892704045,-0.698294921854431,
25.793172996076));
#42794=CARTESIAN_POINT('Ctrl Pts',(22.6057817728151,-0.884088531865305,
25.9773782200491));
#42795=CARTESIAN_POINT('Ctrl Pts',(22.5889742752257,-0.989808265698904,
26.2386796389553));
#42796=CARTESIAN_POINT('Ctrl Pts',(22.5721667776362,-0.992204861021737,
26.5000685690985));
#42797=CARTESIAN_POINT('Ctrl Pts',(22.4278332223638,-0.992581696356067,
26.5000071712556));
#42798=CARTESIAN_POINT('Ctrl Pts',(22.4380067858113,-0.992520308959953,
26.3414407957685));
#42799=CARTESIAN_POINT('Ctrl Pts',(22.4481803492587,-0.953825173771418,
26.1828455329487));
#42800=CARTESIAN_POINT('Ctrl Pts',(22.4583539127062,-0.88068530865534,26.042157092403));
#42801=CARTESIAN_POINT('Ctrl Pts',(22.4689631156045,-0.804413540854797,
25.8954442696148));
#42802=CARTESIAN_POINT('Ctrl Pts',(22.4795723185027,-0.69068398753245,25.7682046698575));
#42803=CARTESIAN_POINT('Ctrl Pts',(22.490181521401,-0.553416234566112,25.6760114004205));
#42804=CARTESIAN_POINT('Ctrl Pts',(22.5007907242993,-0.416148481599767,
25.5838181309836));
#42805=CARTESIAN_POINT('Ctrl Pts',(22.5113999271975,-0.255342528989424,
25.5266711918671));
#42806=CARTESIAN_POINT('Ctrl Pts',(22.5220091300958,-0.0906797366071229,
25.5115649104331));
#42807=CARTESIAN_POINT('Ctrl Pts',(22.5326183329941,0.073983055775169,25.4964586289991));
#42808=CARTESIAN_POINT('Ctrl Pts',(22.5432275358924,0.242502687929425,25.5233930052477));
#42809=CARTESIAN_POINT('Ctrl Pts',(22.5538367387906,0.394253707426228,25.5890714873828));
#42810=CARTESIAN_POINT('Ctrl Pts',(22.5644459416889,0.54600472692304,25.654749969518));
#42811=CARTESIAN_POINT('Ctrl Pts',(22.5750551445872,0.680987133762404,25.7591725575397));
#42812=CARTESIAN_POINT('Ctrl Pts',(22.5856643474855,0.782680163120166,25.8895587635354));
#42813=CARTESIAN_POINT('Ctrl Pts',(22.5962735503837,0.884373192477921,26.019944969531));
#42814=CARTESIAN_POINT('Ctrl Pts',(22.606882753282,0.952776844354082,26.1762947935006));
#42815=CARTESIAN_POINT('Ctrl Pts',(22.6174919561803,0.979519059958022,26.3394722700054));
#42816=CARTESIAN_POINT('Ctrl Pts',(22.6281011590785,1.00626127556196,26.5026497465103));
#42817=CARTESIAN_POINT('Ctrl Pts',(22.6387103619768,0.991342054893685,26.6726548755504));
#42818=CARTESIAN_POINT('Ctrl Pts',(22.6493195648751,0.936587390997702,26.8286803917826));
#42819=CARTESIAN_POINT('Ctrl Pts',(22.6599287677734,0.881832727101723,26.9847059080148));
#42820=CARTESIAN_POINT('Ctrl Pts',(22.6705379706716,0.787242619978021,27.1267518114392));
#42821=CARTESIAN_POINT('Ctrl Pts',(22.6811471735699,0.664394140676646,27.2374328218576));
#42822=CARTESIAN_POINT('Ctrl Pts',(22.6917563764682,0.541545661375256,27.3481138322759));
#42823=CARTESIAN_POINT('Ctrl Pts',(22.7023655793664,0.390438809896197,27.4274299496884));
#42824=CARTESIAN_POINT('Ctrl Pts',(22.7129747822647,0.229567853863308,27.465673516977));
#42825=CARTESIAN_POINT('Ctrl Pts',(22.723583985163,0.0686968978304285,27.5039170842657));
#42826=CARTESIAN_POINT('Ctrl Pts',(22.7341931880613,-0.101938162756261,
27.5010881014307));
#42827=CARTESIAN_POINT('Ctrl Pts',(22.7448023909595,-0.261452963980634,
27.4575328132989));
#42828=CARTESIAN_POINT('Ctrl Pts',(22.7554115938578,-0.420967765205008,
27.4139775251671));
#42829=CARTESIAN_POINT('Ctrl Pts',(22.7660207967561,-0.56936230706707,27.3296959317385));
#42830=CARTESIAN_POINT('Ctrl Pts',(22.7766299996544,-0.688474286903125,
27.2150034246012));
#42831=CARTESIAN_POINT('Ctrl Pts',(22.7872392025526,-0.807586266739185,
27.1003109174639));
#42832=CARTESIAN_POINT('Ctrl Pts',(22.7978484054509,-0.897415684549238,
26.955207496618));
#42833=CARTESIAN_POINT('Ctrl Pts',(22.8084576083492,-0.946968139502241,
26.7974526578902));
#42834=CARTESIAN_POINT('Ctrl Pts',(22.814916146354,-0.977134063994168,26.7014166379228));
#42835=CARTESIAN_POINT('Ctrl Pts',(22.8213746843589,-0.992373431511741,
26.6006920293325));
#42836=CARTESIAN_POINT('Ctrl Pts',(22.8278332223638,-0.99243012155925,26.4999841927042));
#42837=CARTESIAN_POINT('Origin',(18.,0.,26.5));
#42838=CARTESIAN_POINT('',(23.3721667776362,-0.992388032386622,26.499675821275));
#42839=CARTESIAN_POINT('',(23.2278332223638,-0.992528322420212,26.5000239907786));
#42840=CARTESIAN_POINT('',(18.,-0.9925,26.5));
#42841=CARTESIAN_POINT('Ctrl Pts',(23.3721667776362,-0.992388032386622,
26.499675821275));
#42842=CARTESIAN_POINT('Ctrl Pts',(23.3657749250712,-0.992351027245097,
26.5994813785654));
#42843=CARTESIAN_POINT('Ctrl Pts',(23.3593830725062,-0.977461020605066,
26.6994268097226));
#42844=CARTESIAN_POINT('Ctrl Pts',(23.3529912199413,-0.947917745793742,
26.7946503343929));
#42845=CARTESIAN_POINT('Ctrl Pts',(23.3424056844407,-0.898991181681411,
26.9523498417946));
#42846=CARTESIAN_POINT('Ctrl Pts',(23.3318201489402,-0.809875667003528,
27.0970987593237));
#42847=CARTESIAN_POINT('Ctrl Pts',(23.3212346134396,-0.691503973124327,
27.2119684246678));
#42848=CARTESIAN_POINT('Ctrl Pts',(23.3106490779391,-0.573132279245139,
27.3268380900118));
#42849=CARTESIAN_POINT('Ctrl Pts',(23.3000635424386,-0.425504406164642,
27.4118285031709));
#42850=CARTESIAN_POINT('Ctrl Pts',(23.2894780069381,-0.266592626638276,
27.4561726651644));
#42851=CARTESIAN_POINT('Ctrl Pts',(23.2788924714375,-0.107680847111892,
27.500516827158));
#42852=CARTESIAN_POINT('Ctrl Pts',(23.268306935937,0.0625148388603637,27.5042147379859));
#42853=CARTESIAN_POINT('Ctrl Pts',(23.2577214004365,0.223286445894541,27.4670952067496));
#42854=CARTESIAN_POINT('Ctrl Pts',(23.2471358649359,0.384058052928701,27.4299756755133));
#42855=CARTESIAN_POINT('Ctrl Pts',(23.2365503294354,0.535405581024785,27.3520387022128));
#42856=CARTESIAN_POINT('Ctrl Pts',(23.2259647939349,0.658792131885872,27.2425164787066));
#42857=CARTESIAN_POINT('Ctrl Pts',(23.2153792584343,0.782178682746974,27.1329942552003));
#42858=CARTESIAN_POINT('Ctrl Pts',(23.2047937229338,0.877604256373074,26.9918867814884));
#42859=CARTESIAN_POINT('Ctrl Pts',(23.1942081874333,0.933635937153906,26.8367502329998));
#42860=CARTESIAN_POINT('Ctrl Pts',(23.1836226519327,0.989667617934738,26.6816136845112));
#42861=CARTESIAN_POINT('Ctrl Pts',(23.1730371164322,1.0063054058703,26.5124480612458));
#42862=CARTESIAN_POINT('Ctrl Pts',(23.1624515809317,0.981144614563025,26.3492614260964));
#42863=CARTESIAN_POINT('Ctrl Pts',(23.1518660454311,0.955983823255751,26.186074790947));
#42864=CARTESIAN_POINT('Ctrl Pts',(23.1412805099306,0.889024452705641,26.0288671439135));
#42865=CARTESIAN_POINT('Ctrl Pts',(23.1306949744301,0.789132149463115,25.8978837846844));
#42866=CARTESIAN_POINT('Ctrl Pts',(23.1201094389296,0.68923984622059,25.7669004254553));
#42867=CARTESIAN_POINT('Ctrl Pts',(23.109523903429,0.55641461028565,25.6621413540304));
#42868=CARTESIAN_POINT('Ctrl Pts',(23.0989383679285,0.405594721429978,25.5944723567525));
#42869=CARTESIAN_POINT('Ctrl Pts',(23.0883528324279,0.254774832574307,25.5268033594745));
#42870=CARTESIAN_POINT('Ctrl Pts',(23.0777672969274,0.0859602907979053,
25.4962244363435));
#42871=CARTESIAN_POINT('Ctrl Pts',(23.0671817614269,-0.0782820979201608,
25.5094990537566));
#42872=CARTESIAN_POINT('Ctrl Pts',(23.0460106904258,-0.406766875356302,
25.5360482885829));
#42873=CARTESIAN_POINT('Ctrl Pts',(23.0248396194247,-0.7169630405591,25.7380116855861));
#42874=CARTESIAN_POINT('Ctrl Pts',(23.0036685484237,-0.874142114566764,
26.0276698454422));
#42875=CARTESIAN_POINT('Ctrl Pts',(22.9931679581612,-0.952100997889672,
26.1713367224124));
#42876=CARTESIAN_POINT('Ctrl Pts',(22.9826673678987,-0.992417099477605,
26.3365768418982));
#42877=CARTESIAN_POINT('Ctrl Pts',(22.9721667776362,-0.992215768961308,
26.5005746468071));
#42878=CARTESIAN_POINT('Ctrl Pts',(22.8278332223638,-0.99243012155925,26.4999841927042));
#42879=CARTESIAN_POINT('Ctrl Pts',(22.8319838872572,-0.992466554168273,
26.43526296916));
#42880=CARTESIAN_POINT('Ctrl Pts',(22.8361345521506,-0.986232297652164,
26.3705486727048));
#42881=CARTESIAN_POINT('Ctrl Pts',(22.840285217044,-0.973659369893009,26.3070902482045));
#42882=CARTESIAN_POINT('Ctrl Pts',(22.8508944199423,-0.941522653234819,
26.1448889338561));
#42883=CARTESIAN_POINT('Ctrl Pts',(22.8615036228405,-0.867973727822483,
25.990892561769));
#42884=CARTESIAN_POINT('Ctrl Pts',(22.8721128257388,-0.762014392692314,
25.8639490537323));
#42885=CARTESIAN_POINT('Ctrl Pts',(22.8827220286371,-0.65605505756214,25.7370055456956));
#42886=CARTESIAN_POINT('Ctrl Pts',(22.8933312315354,-0.517685312714129,
25.6371149017093));
#42887=CARTESIAN_POINT('Ctrl Pts',(22.9039404344336,-0.363840505997963,
25.5765029360559));
#42888=CARTESIAN_POINT('Ctrl Pts',(22.9145496373319,-0.209995699281814,
25.5158909704025));
#42889=CARTESIAN_POINT('Ctrl Pts',(22.9251588402302,-0.0406758306975135,
25.4945576830821));
#42890=CARTESIAN_POINT('Ctrl Pts',(22.9357680431284,0.123395704799732,25.5151140974939));
#42891=CARTESIAN_POINT('Ctrl Pts',(22.9463772460267,0.287467240296987,25.5356705119057));
#42892=CARTESIAN_POINT('Ctrl Pts',(22.956986448925,0.446290442707186,25.5981166280497));
#42893=CARTESIAN_POINT('Ctrl Pts',(22.9675956518233,0.580426624892681,25.6948095417642));
#42894=CARTESIAN_POINT('Ctrl Pts',(22.9782048547215,0.714562807078176,25.7915024554787));
#42895=CARTESIAN_POINT('Ctrl Pts',(22.9888140576198,0.824011969038968,25.9224421667636));
#42896=CARTESIAN_POINT('Ctrl Pts',(22.9994232605181,0.895378410496085,26.0716027043319));
#42897=CARTESIAN_POINT('Ctrl Pts',(23.0100324634163,0.966744851953198,26.2207632419001));
#42898=CARTESIAN_POINT('Ctrl Pts',(23.0206416663146,1.00002857290664,26.3881446057516));
#42899=CARTESIAN_POINT('Ctrl Pts',(23.0312508692129,0.991155912653363,26.553260658375));
#42900=CARTESIAN_POINT('Ctrl Pts',(23.0418600721112,0.982283252400084,26.7183767109984));
#42901=CARTESIAN_POINT('Ctrl Pts',(23.0524692750094,0.931254210940078,26.8812274523936));
#42902=CARTESIAN_POINT('Ctrl Pts',(23.0630784779077,0.844314333992244,27.0218812569287));
#42903=CARTESIAN_POINT('Ctrl Pts',(23.073687680806,0.75737445704441,27.1625350614638));
#42904=CARTESIAN_POINT('Ctrl Pts',(23.0842968837043,0.634523744608749,27.2809919291387));
#42905=CARTESIAN_POINT('Ctrl Pts',(23.0949060866025,0.490798139339951,27.3627536886845));
#42906=CARTESIAN_POINT('Ctrl Pts',(23.1055152895008,0.347072534071171,27.4445154482302));
#42907=CARTESIAN_POINT('Ctrl Pts',(23.1161244923991,0.182472035969259,27.4895820996468));
#42908=CARTESIAN_POINT('Ctrl Pts',(23.1267336952973,0.0171424268642523,
27.492437845973));
#42909=CARTESIAN_POINT('Ctrl Pts',(23.1373428981956,-0.148187182240773,
27.4952935922991));
#42910=CARTESIAN_POINT('Ctrl Pts',(23.1479521010939,-0.314245902348893,
27.4559384335349));
#42911=CARTESIAN_POINT('Ctrl Pts',(23.1585613039922,-0.460709476942957,
27.3791891257137));
#42912=CARTESIAN_POINT('Ctrl Pts',(23.1691705068904,-0.607173051537012,
27.3024398178925));
#42913=CARTESIAN_POINT('Ctrl Pts',(23.1797797097887,-0.734041480617014,
27.1882963610144));
#42914=CARTESIAN_POINT('Ctrl Pts',(23.190388912687,-0.825787085209699,27.0507289994354));
#42915=CARTESIAN_POINT('Ctrl Pts',(23.2009981155852,-0.917532689802385,
26.9131616378564));
#42916=CARTESIAN_POINT('Ctrl Pts',(23.2116073184835,-0.974155469907755,
26.7521703715764));
#42917=CARTESIAN_POINT('Ctrl Pts',(23.2222165213818,-0.988725251025931,
26.5874592413754));
#42918=CARTESIAN_POINT('Ctrl Pts',(23.2240887550425,-0.991296418237979,
26.558392239339));
#42919=CARTESIAN_POINT('Ctrl Pts',(23.2259609887031,-0.99255794656802,26.5292093911432));
#42920=CARTESIAN_POINT('Ctrl Pts',(23.2278332223638,-0.992528322420212,
26.5000239907786));
#42921=CARTESIAN_POINT('Origin',(18.,0.,26.5));
#42922=CARTESIAN_POINT('',(23.7721667776362,-0.992500262637294,26.5000027623734));
#42923=CARTESIAN_POINT('',(23.6278332223638,-0.992486745736932,26.499974029444));
#42924=CARTESIAN_POINT('',(18.,-0.9925,26.5));
#42925=CARTESIAN_POINT('Ctrl Pts',(23.7721667776362,-0.992500262637294,
26.5000027623734));
#42926=CARTESIAN_POINT('Ctrl Pts',(23.7700535532448,-0.992512026843979,
26.5329256477546));
#42927=CARTESIAN_POINT('Ctrl Pts',(23.7679403288534,-0.990885127798118,
26.5658486953477));
#42928=CARTESIAN_POINT('Ctrl Pts',(23.765827104462,-0.987599253356915,26.5986128659939));
#42929=CARTESIAN_POINT('Ctrl Pts',(23.7552415689615,-0.971139694831468,
26.7627347135987));
#42930=CARTESIAN_POINT('Ctrl Pts',(23.7446560334609,-0.913053206437673,
26.9228700285835));
#42931=CARTESIAN_POINT('Ctrl Pts',(23.7340704979604,-0.820140389914714,
27.0592025885277));
#42932=CARTESIAN_POINT('Ctrl Pts',(23.7234849624599,-0.727227573391749,
27.1955351484718));
#42933=CARTESIAN_POINT('Ctrl Pts',(23.7128994269593,-0.599488428739612,
27.3080649533752));
#42934=CARTESIAN_POINT('Ctrl Pts',(23.7023138914588,-0.452644851679794,
27.3833134291327));
#42935=CARTESIAN_POINT('Ctrl Pts',(23.6917283559583,-0.305801274619976,
27.4585619048902));
#42936=CARTESIAN_POINT('Ctrl Pts',(23.6811428204577,-0.13985326515247,27.4965290515018));
#42937=CARTESIAN_POINT('Ctrl Pts',(23.6705572849572,0.0250760671767568,
27.4923250400148));
#42938=CARTESIAN_POINT('Ctrl Pts',(23.6599717494567,0.190005399506003,27.4881210285279));
#42939=CARTESIAN_POINT('Ctrl Pts',(23.6493862139561,0.353916054696976,27.4417458589422));
#42940=CARTESIAN_POINT('Ctrl Pts',(23.6388006784556,0.49675088812807,27.3592527787064));
#42941=CARTESIAN_POINT('Ctrl Pts',(23.6282151429551,0.63958572155914,27.2767596984705));
#42942=CARTESIAN_POINT('Ctrl Pts',(23.6176296074546,0.761344733230343,27.1581487075844));
#42943=CARTESIAN_POINT('Ctrl Pts',(23.607044071954,0.847292882654172,27.017166939539));
#42944=CARTESIAN_POINT('Ctrl Pts',(23.5964585364535,0.933241032078011,26.8761851714936));
#42945=CARTESIAN_POINT('Ctrl Pts',(23.5858730009529,0.983378319254465,26.7128326262889));
#42946=CARTESIAN_POINT('Ctrl Pts',(23.5752874654524,0.991433494211962,26.5483023044681));
#42947=CARTESIAN_POINT('Ctrl Pts',(23.5647019299519,0.999488669169459,26.3837719826473));
#42948=CARTESIAN_POINT('Ctrl Pts',(23.5541163944514,0.965461731907988,26.2180638842104));
#42949=CARTESIAN_POINT('Ctrl Pts',(23.5435308589508,0.893769977117369,26.0691141465064));
#42950=CARTESIAN_POINT('Ctrl Pts',(23.5329453234503,0.822078222326754,25.9201644088025));
#42951=CARTESIAN_POINT('Ctrl Pts',(23.5223597879498,0.712721650006991,25.7879730318314));
#42952=CARTESIAN_POINT('Ctrl Pts',(23.5117742524492,0.578594147325075,25.6922568328701));
#42953=CARTESIAN_POINT('Ctrl Pts',(23.4906031814482,0.310339141961234,25.5008244349476));
#42954=CARTESIAN_POINT('Ctrl Pts',(23.4694321104471,-0.0569995848512428,
25.4552927490642));
#42955=CARTESIAN_POINT('Ctrl Pts',(23.448261039446,-0.363874645107573,25.5754376959817));
#42956=CARTESIAN_POINT('Ctrl Pts',(23.4376755039455,-0.517312175235725,
25.6355101694404));
#42957=CARTESIAN_POINT('Ctrl Pts',(23.427089968445,-0.655633788724846,25.7370018010994));
#42958=CARTESIAN_POINT('Ctrl Pts',(23.4165044329445,-0.761521951267013,
25.8639404835428));
#42959=CARTESIAN_POINT('Ctrl Pts',(23.4059188974439,-0.867410113809191,
25.9908791659863));
#42960=CARTESIAN_POINT('Ctrl Pts',(23.3953333619434,-0.94086482540441,26.1432648992143));
#42961=CARTESIAN_POINT('Ctrl Pts',(23.3847478264428,-0.97322337442863,26.3047828144655));
#42962=CARTESIAN_POINT('Ctrl Pts',(23.3805541435073,-0.986042895449097,
26.3687715399239));
#42963=CARTESIAN_POINT('Ctrl Pts',(23.3763604605718,-0.992412311393211,
26.4341935752085));
#42964=CARTESIAN_POINT('Ctrl Pts',(23.3721667776362,-0.992388032386622,
26.499675821275));
#42965=CARTESIAN_POINT('Ctrl Pts',(23.2278332223638,-0.992528322420212,
26.5000239907786));
#42966=CARTESIAN_POINT('Ctrl Pts',(23.2365701916014,-0.992390078314509,
26.3638273447456));
#42967=CARTESIAN_POINT('Ctrl Pts',(23.245307160839,-0.964134182439229,26.2275751196904));
#42968=CARTESIAN_POINT('Ctrl Pts',(23.2540441300766,-0.909639323030658,
26.1027808628545));
#42969=CARTESIAN_POINT('Ctrl Pts',(23.2646533329749,-0.843466831786224,
25.9512446086564));
#42970=CARTESIAN_POINT('Ctrl Pts',(23.2752625358732,-0.738605067166374,
25.816603094382));
#42971=CARTESIAN_POINT('Ctrl Pts',(23.2858717387714,-0.607888268779764,
25.7153353623374));
#42972=CARTESIAN_POINT('Ctrl Pts',(23.2964809416697,-0.477171470393162,
25.6140676302928));
#42973=CARTESIAN_POINT('Ctrl Pts',(23.307090144568,-0.32059963823978,25.5461736804781));
#42974=CARTESIAN_POINT('Ctrl Pts',(23.3176993474663,-0.157335909780756,
25.5199631882364));
#42975=CARTESIAN_POINT('Ctrl Pts',(23.3283085503645,0.00592781867827763,
25.4937526959947));
#42976=CARTESIAN_POINT('Ctrl Pts',(23.3389177532628,0.175883443442949,25.509225661326));
#42977=CARTESIAN_POINT('Ctrl Pts',(23.3495269561611,0.331729758096689,25.5644883172769));
#42978=CARTESIAN_POINT('Ctrl Pts',(23.3601361590593,0.487576072750439,25.6197509732278));
#42979=CARTESIAN_POINT('Ctrl Pts',(23.3707453619576,0.6293130772932,25.7148033197982));
#42980=CARTESIAN_POINT('Ctrl Pts',(23.3813545648559,0.739593298274526,25.8380117115344));
#42981=CARTESIAN_POINT('Ctrl Pts',(23.3919637677542,0.849873519255846,25.9612201032705));
#42982=CARTESIAN_POINT('Ctrl Pts',(23.4025729706524,0.928696956675713,26.1125845401724));
#42983=CARTESIAN_POINT('Ctrl Pts',(23.4131821735507,0.966416253498947,26.2735792282247));
#42984=CARTESIAN_POINT('Ctrl Pts',(23.423791376449,1.00413555032218,26.434573916277));
#42985=CARTESIAN_POINT('Ctrl Pts',(23.4344005793472,1.00075070654879,26.6051988554798));
#42986=CARTESIAN_POINT('Ctrl Pts',(23.4450097822455,0.956675999929901,26.7645709206931));
#42987=CARTESIAN_POINT('Ctrl Pts',(23.4556189851438,0.912601293311011,26.9239429859064));
#42988=CARTESIAN_POINT('Ctrl Pts',(23.4662281880421,0.827836723846627,27.0720621771303));
#42989=CARTESIAN_POINT('Ctrl Pts',(23.4768373909403,0.712756795520865,27.1907998924125));
#42990=CARTESIAN_POINT('Ctrl Pts',(23.4874465938386,0.597676867195097,27.3095376076947));
#42991=CARTESIAN_POINT('Ctrl Pts',(23.4980557967369,0.452281580007953,27.3988938470351));
#42992=CARTESIAN_POINT('Ctrl Pts',(23.5086649996351,0.294366151887474,27.4479321228554));
#42993=CARTESIAN_POINT('Ctrl Pts',(23.5192742025334,0.136450723767013,27.4969703986757));
#42994=CARTESIAN_POINT('Ctrl Pts',(23.5298834054317,-0.0339848452867753,
27.5056907109758));
#42995=CARTESIAN_POINT('Ctrl Pts',(23.54049260833,-0.196080607522645,27.4730257634163));
#42996=CARTESIAN_POINT('Ctrl Pts',(23.5511018112282,-0.358176369758524,
27.4403608158567));
#42997=CARTESIAN_POINT('Ctrl Pts',(23.5617110141265,-0.511932325176479,
27.3663106084376));
#42998=CARTESIAN_POINT('Ctrl Pts',(23.5723202170248,-0.638529977060899,
27.2599382930955));
#42999=CARTESIAN_POINT('Ctrl Pts',(23.582929419923,-0.765127628945325,27.1535659777533));
#43000=CARTESIAN_POINT('Ctrl Pts',(23.5935386228213,-0.86456697729621,27.0148715544882));
#43001=CARTESIAN_POINT('Ctrl Pts',(23.6041478257196,-0.924677442800011,
26.8608301091859));
#43002=CARTESIAN_POINT('Ctrl Pts',(23.6120429579343,-0.9694103107819,26.7461959006717));
#43003=CARTESIAN_POINT('Ctrl Pts',(23.6199380901491,-0.992362825760545,
26.6230625044533));
#43004=CARTESIAN_POINT('Ctrl Pts',(23.6278332223638,-0.992486745736932,
26.499974029444));
#43005=CARTESIAN_POINT('Origin',(18.,0.,26.5));
#43006=CARTESIAN_POINT('',(24.1721667776362,-0.9925,26.5000000000003));
#43007=CARTESIAN_POINT('',(24.0278332223638,-0.992459651580774,26.5000236090481));
#43008=CARTESIAN_POINT('',(18.,-0.9925,26.5));
#43009=CARTESIAN_POINT('Ctrl Pts',(24.1721667776362,-0.99257394234428,26.4999790041826));
#43010=CARTESIAN_POINT('Ctrl Pts',(24.1637466459179,-0.992421357292391,
26.6312298628555));
#43011=CARTESIAN_POINT('Ctrl Pts',(24.1553265141995,-0.966145501910799,
26.7625240981299));
#43012=CARTESIAN_POINT('Ctrl Pts',(24.1469063824812,-0.915423483254653,
26.8835750541215));
#43013=CARTESIAN_POINT('Ctrl Pts',(24.1363208469806,-0.851657292047284,
27.0357566630184));
#43014=CARTESIAN_POINT('Ctrl Pts',(24.1257353114801,-0.749254527386481,
27.171749015222));
#43015=CARTESIAN_POINT('Ctrl Pts',(24.1151497759796,-0.620448439739691,
27.274842905246));
#43016=CARTESIAN_POINT('Ctrl Pts',(24.104564240479,-0.4916423520929,27.37793679527));
#43017=CARTESIAN_POINT('Ctrl Pts',(24.0939787049785,-0.336432941460122,
27.4481322231143));
#43018=CARTESIAN_POINT('Ctrl Pts',(24.083393169478,-0.174056574351007,27.4771290045311));
#43019=CARTESIAN_POINT('Ctrl Pts',(24.0728076339774,-0.0116802072418913,
27.5061257859478));
#43020=CARTESIAN_POINT('Ctrl Pts',(24.0622220984769,0.157863116343561,27.493923920937));
#43021=CARTESIAN_POINT('Ctrl Pts',(24.0516365629764,0.314446804184475,27.4415360214494));
#43022=CARTESIAN_POINT('Ctrl Pts',(24.0410510274758,0.471030492025389,27.3891481219617));
#43023=CARTESIAN_POINT('Ctrl Pts',(24.0304654919753,0.614654544121765,27.2965741879971));
#43024=CARTESIAN_POINT('Ctrl Pts',(24.0198799564748,0.726863976145958,27.1759750337428));
#43025=CARTESIAN_POINT('Ctrl Pts',(24.0092944209742,0.839073408170171,27.0553758794885));
#43026=CARTESIAN_POINT('Ctrl Pts',(23.9987088854737,0.91986822012219,26.9067515049444));
#43027=CARTESIAN_POINT('Ctrl Pts',(23.9881233499732,0.961064596018904,26.7466621840013));
#43028=CARTESIAN_POINT('Ctrl Pts',(23.9775378144726,1.00226097191561,26.5865728630582));
#43029=CARTESIAN_POINT('Ctrl Pts',(23.9669522789721,1.00385891175703,26.4150185957161));
#43030=CARTESIAN_POINT('Ctrl Pts',(23.9563667434716,0.963007589610471,26.2553848048128));
#43031=CARTESIAN_POINT('Ctrl Pts',(23.9351956724705,0.881304945317355,25.9361172230061));
#43032=CARTESIAN_POINT('Ctrl Pts',(23.9140246014695,0.629805253072327,25.6645315469549));
#43033=CARTESIAN_POINT('Ctrl Pts',(23.8928535304684,0.31774316757647,25.5585864400688));
#43034=CARTESIAN_POINT('Ctrl Pts',(23.8822679949679,0.161712124828541,25.5056138866258));
#43035=CARTESIAN_POINT('Ctrl Pts',(23.8716824594673,-0.00945951623209451,
25.494051475474));
#43036=CARTESIAN_POINT('Ctrl Pts',(23.8610969239668,-0.172236578558568,
25.5228500873746));
#43037=CARTESIAN_POINT('Ctrl Pts',(23.8505113884663,-0.335013640885051,
25.5516486992753));
#43038=CARTESIAN_POINT('Ctrl Pts',(23.8399258529657,-0.489396124477372,
25.6208083342283));
#43039=CARTESIAN_POINT('Ctrl Pts',(23.8293403174652,-0.618244943128008,
25.7234391998311));
#43040=CARTESIAN_POINT('Ctrl Pts',(23.8187547819647,-0.747093761778644,
25.826070065434));
#43041=CARTESIAN_POINT('Ctrl Pts',(23.8081692464641,-0.850408915487596,
25.9621721616866));
#43042=CARTESIAN_POINT('Ctrl Pts',(23.7975837109636,-0.914650178013526,
26.1142773999254));
#43043=CARTESIAN_POINT('Ctrl Pts',(23.7891113998545,-0.966066751330558,
26.2360173817735));
#43044=CARTESIAN_POINT('Ctrl Pts',(23.7806390887453,-0.992453097736398,
26.3680087684108));
#43045=CARTESIAN_POINT('Ctrl Pts',(23.7721667776362,-0.992500262637294,
26.5000027623734));
#43046=CARTESIAN_POINT('Ctrl Pts',(23.6278332223638,-0.992486745736932,
26.499974029444));
#43047=CARTESIAN_POINT('Ctrl Pts',(23.6305472930473,-0.992529345096369,
26.457660511137));
#43048=CARTESIAN_POINT('Ctrl Pts',(23.6332613637309,-0.989874188395367,
26.415352301368));
#43049=CARTESIAN_POINT('Ctrl Pts',(23.6359754344144,-0.984478691600277,
26.3733964980608));
#43050=CARTESIAN_POINT('Ctrl Pts',(23.6465846373127,-0.96338789224003,26.2093927995774));
#43051=CARTESIAN_POINT('Ctrl Pts',(23.657193840211,-0.900424710862815,26.0507738699499));
#43052=CARTESIAN_POINT('Ctrl Pts',(23.6678030431092,-0.803295336271083,
25.9169533949645));
#43053=CARTESIAN_POINT('Ctrl Pts',(23.6784122460075,-0.706165961679351,
25.7831329199791));
#43054=CARTESIAN_POINT('Ctrl Pts',(23.6890214489058,-0.574870393873098,
25.6741108996358));
#43055=CARTESIAN_POINT('Ctrl Pts',(23.699630651804,-0.425478158125808,25.6032307555028));
#43056=CARTESIAN_POINT('Ctrl Pts',(23.7102398547023,-0.276085922378518,
25.5323506113697));
#43057=CARTESIAN_POINT('Ctrl Pts',(23.7208490576006,-0.108597018690186,
25.4996123434469));
#43058=CARTESIAN_POINT('Ctrl Pts',(23.7314582604989,0.0564892534135627,
25.5090228533578));
#43059=CARTESIAN_POINT('Ctrl Pts',(23.7420674633972,0.221575525517311,25.5184333632687));
#43060=CARTESIAN_POINT('Ctrl Pts',(23.7526766662954,0.384259166036481,25.5699926510134));
#43061=CARTESIAN_POINT('Ctrl Pts',(23.7632858691937,0.524629001147119,25.6573902729771));
#43062=CARTESIAN_POINT('Ctrl Pts',(23.773895072092,0.664998836257765,25.7447878949408));
#43063=CARTESIAN_POINT('Ctrl Pts',(23.7845042749902,0.783054865959882,25.8680238511235));
#43064=CARTESIAN_POINT('Ctrl Pts',(23.7951134778885,0.864347978339919,26.0120150481234));
#43065=CARTESIAN_POINT('Ctrl Pts',(23.8057226807868,0.945641090719952,26.1560062451233));
#43066=CARTESIAN_POINT('Ctrl Pts',(23.816331883685,0.990171285777908,26.3207526829404));
#43067=CARTESIAN_POINT('Ctrl Pts',(23.8269410865833,0.992488424511603,26.486090717893));
#43068=CARTESIAN_POINT('Ctrl Pts',(23.8375502894816,0.994805563245297,26.6514287528456));
#43069=CARTESIAN_POINT('Ctrl Pts',(23.8481594923799,0.954909645654713,26.8173583849337));
#43070=CARTESIAN_POINT('Ctrl Pts',(23.8587686952781,0.87768361231997,26.9635711569794));
#43071=CARTESIAN_POINT('Ctrl Pts',(23.8693778981764,0.800457578985232,27.1097839290251));
#43072=CARTESIAN_POINT('Ctrl Pts',(23.8799871010747,0.685901429906335,27.2362798410283));
#43073=CARTESIAN_POINT('Ctrl Pts',(23.890596303973,0.54803591965721,27.3275768071205));
#43074=CARTESIAN_POINT('Ctrl Pts',(23.9012055068712,0.410170409408084,27.4188737732127));
#43075=CARTESIAN_POINT('Ctrl Pts',(23.9118147097695,0.248995537988726,27.474971793394));
#43076=CARTESIAN_POINT('Ctrl Pts',(23.9224239126678,0.0842378179768146,
27.4890049195736));
#43077=CARTESIAN_POINT('Ctrl Pts',(23.933033115566,-0.0805199020350873,
27.5030380457532));
#43078=CARTESIAN_POINT('Ctrl Pts',(23.9436423184643,-0.248860470639547,
27.4750062779312));
#43079=CARTESIAN_POINT('Ctrl Pts',(23.9542515213626,-0.400180351350601,
27.4083404798374));
#43080=CARTESIAN_POINT('Ctrl Pts',(23.9648607242609,-0.551500232061663,
27.3416746817435));
#43081=CARTESIAN_POINT('Ctrl Pts',(23.9754699271591,-0.685799424879341,
27.2363748533779));
#43082=CARTESIAN_POINT('Ctrl Pts',(23.9860791300574,-0.786640784900299,
27.1053288498409));
#43083=CARTESIAN_POINT('Ctrl Pts',(23.9966883329557,-0.887482144921262,
26.9742828463039));
#43084=CARTESIAN_POINT('Ctrl Pts',(24.007297535854,-0.954865672145517,26.8174906675955));
#43085=CARTESIAN_POINT('Ctrl Pts',(24.0179067387522,-0.980544162864392,
26.6541424198293));
#43086=CARTESIAN_POINT('Ctrl Pts',(24.0212155666228,-0.988552842364468,
26.6031969114822));
#43087=CARTESIAN_POINT('Ctrl Pts',(24.0245243944933,-0.992504836310417,
26.551613688536));
#43088=CARTESIAN_POINT('Ctrl Pts',(24.0278332223638,-0.992459651580774,
26.5000236090481));
#43089=CARTESIAN_POINT('Origin',(18.,0.,26.5));
#43090=CARTESIAN_POINT('',(24.5721667776362,-0.9925,26.5000000000003));
#43091=CARTESIAN_POINT('',(24.4278332223638,-0.992555410679472,26.4999811860602));
#43092=CARTESIAN_POINT('',(18.,-0.9925,26.5));
#43093=CARTESIAN_POINT('Ctrl Pts',(24.5721667776362,-0.9925,26.5000000000003));
#43094=CARTESIAN_POINT('Ctrl Pts',(24.5554259338597,-0.992499999999917,
26.7609923249232));
#43095=CARTESIAN_POINT('Ctrl Pts',(24.5386850900831,-0.884539443097234,
27.020349130175));
#43096=CARTESIAN_POINT('Ctrl Pts',(24.5219442463066,-0.699346033936665,
27.2042523516589));
#43097=CARTESIAN_POINT('Ctrl Pts',(24.5052034025301,-0.514152624776095,
27.3881555731427));
#43098=CARTESIAN_POINT('Ctrl Pts',(24.4884625587535,-0.254047408344091,
27.4943003359058));
#43099=CARTESIAN_POINT('Ctrl Pts',(24.471721714977,0.00693853867385297,
27.4924757461425));
#43100=CARTESIAN_POINT('Ctrl Pts',(24.4549808712005,0.267924485691796,27.4906511563792));
#43101=CARTESIAN_POINT('Ctrl Pts',(24.4382400274239,0.526520203888397,27.3808800818307));
#43102=CARTESIAN_POINT('Ctrl Pts',(24.4214991836474,0.70912424955959,27.1944055361866));
#43103=CARTESIAN_POINT('Ctrl Pts',(24.4047583398709,0.891728295230784,27.0079309905425));
#43104=CARTESIAN_POINT('Ctrl Pts',(24.3880174960943,0.996052076106294,26.7470900753835));
#43105=CARTESIAN_POINT('Ctrl Pts',(24.3712766523178,0.992402985755312,26.4861232617686));
#43106=CARTESIAN_POINT('Ctrl Pts',(24.3545358085413,0.988753895404331,26.2251564481538));
#43107=CARTESIAN_POINT('Ctrl Pts',(24.3377949647647,0.877177668191286,25.9673344556899));
#43108=CARTESIAN_POINT('Ctrl Pts',(24.3210541209882,0.689431099871355,25.7860385104712));
#43109=CARTESIAN_POINT('Ctrl Pts',(24.3043132772117,0.501684531551424,25.6047425652525));
#43110=CARTESIAN_POINT('Ctrl Pts',(24.2875724334351,0.240120666075239,25.5022448650133));
#43111=CARTESIAN_POINT('Ctrl Pts',(24.2708315896586,-0.0208142595733872,
25.5077182776054));
#43112=CARTESIAN_POINT('Ctrl Pts',(24.2540907458821,-0.281749185222014,
25.5131916901974));
#43113=CARTESIAN_POINT('Ctrl Pts',(24.2373499021055,-0.538784851091028,
25.6265676168681));
#43114=CARTESIAN_POINT('Ctrl Pts',(24.220609058329,-0.718763835149907,25.815577031887));
#43115=CARTESIAN_POINT('Ctrl Pts',(24.2044616314314,-0.89236305911901,25.9978865828699));
#43116=CARTESIAN_POINT('Ctrl Pts',(24.1883142045338,-0.992500000000069,
26.2482591353353));
#43117=CARTESIAN_POINT('Ctrl Pts',(24.1721667776362,-0.9925,26.5000000000003));
#43118=CARTESIAN_POINT('Ctrl Pts',(24.0278332223638,-0.992459651580774,
26.5000236090481));
#43119=CARTESIAN_POINT('Ctrl Pts',(24.0351335973915,-0.992359959035612,
26.3861987312633));
#43120=CARTESIAN_POINT('Ctrl Pts',(24.0424339724193,-0.972802385036297,
26.2723404764931));
#43121=CARTESIAN_POINT('Ctrl Pts',(24.049734347447,-0.934426046269535,26.1652243960929));
#43122=CARTESIAN_POINT('Ctrl Pts',(24.0603435503453,-0.878655984742315,
26.0095589369469));
#43123=CARTESIAN_POINT('Ctrl Pts',(24.0709527532436,-0.783142407474387,
25.8681323354789));
#43124=CARTESIAN_POINT('Ctrl Pts',(24.0815619561419,-0.659575410860569,
25.7582540742907));
#43125=CARTESIAN_POINT('Ctrl Pts',(24.0921711590401,-0.536008414246758,
25.6483758131025));
#43126=CARTESIAN_POINT('Ctrl Pts',(24.1027803619384,-0.384387998287034,
25.5700458921941));
#43127=CARTESIAN_POINT('Ctrl Pts',(24.1133895648367,-0.223271286781966,
25.5328512661348));
#43128=CARTESIAN_POINT('Ctrl Pts',(24.123998767735,-0.0621545752768985,
25.4956566400755));
#43129=CARTESIAN_POINT('Ctrl Pts',(24.1346079706332,0.108458431773511,25.4995973088654));
#43130=CARTESIAN_POINT('Ctrl Pts',(24.1452171735315,0.267686069629295,25.5441909662256));
#43131=CARTESIAN_POINT('Ctrl Pts',(24.1558263764298,0.426913707485089,25.5887846235859));
#43132=CARTESIAN_POINT('Ctrl Pts',(24.166435579328,0.574755976146227,25.6740312695166));
#43133=CARTESIAN_POINT('Ctrl Pts',(24.1770447822263,0.693118166762793,25.7894973977376));
#43134=CARTESIAN_POINT('Ctrl Pts',(24.1876539851246,0.811480357379345,25.9049635259586));
#43135=CARTESIAN_POINT('Ctrl Pts',(24.1982631880229,0.900362469951331,26.0506491364699));
#43136=CARTESIAN_POINT('Ctrl Pts',(24.2088723909211,0.948886046216982,26.2087234780952));
#43137=CARTESIAN_POINT('Ctrl Pts',(24.2194815938194,0.997409622482638,26.3667978197206));
#43138=CARTESIAN_POINT('Ctrl Pts',(24.2300907967177,1.00557466244195,26.53726089246));
#43139=CARTESIAN_POINT('Ctrl Pts',(24.2406999996159,0.972381830639979,26.6992493823315));
#43140=CARTESIAN_POINT('Ctrl Pts',(24.2513092025142,0.939188998838011,26.8612378722031));
#43141=CARTESIAN_POINT('Ctrl Pts',(24.2619184054125,0.86463829527477,27.0147517792067));
#43142=CARTESIAN_POINT('Ctrl Pts',(24.2725276083108,0.757854128603812,27.141002231413));
#43143=CARTESIAN_POINT('Ctrl Pts',(24.283136811209,0.651069961932841,27.2672526836192));
#43144=CARTESIAN_POINT('Ctrl Pts',(24.2937460141073,0.512052332154146,27.3662396810281));
#43145=CARTESIAN_POINT('Ctrl Pts',(24.3043552170056,0.357815883040657,27.4258480084561));
#43146=CARTESIAN_POINT('Ctrl Pts',(24.3149644199038,0.203579433927185,27.4854563358841));
#43147=CARTESIAN_POINT('Ctrl Pts',(24.3255736228021,0.0341241654789235,
27.5056859933312));
#43148=CARTESIAN_POINT('Ctrl Pts',(24.3361828257004,-0.129809955490691,
27.48406103285));
#43149=CARTESIAN_POINT('Ctrl Pts',(24.3467920285987,-0.293744076460323,
27.4624360723688));
#43150=CARTESIAN_POINT('Ctrl Pts',(24.357401231497,-0.452157049951307,27.3989564939593));
#43151=CARTESIAN_POINT('Ctrl Pts',(24.3680104343952,-0.585660397558057,
27.3013916892821));
#43152=CARTESIAN_POINT('Ctrl Pts',(24.3786196372935,-0.719163745164792,
27.203826884605));
#43153=CARTESIAN_POINT('Ctrl Pts',(24.3892288401918,-0.827757466887299,
27.0721768536602));
#43154=CARTESIAN_POINT('Ctrl Pts',(24.39983804309,-0.898150561476123,26.9225545051687));
#43155=CARTESIAN_POINT('Ctrl Pts',(24.4091697695146,-0.960067475233129,
26.7909484989009));
#43156=CARTESIAN_POINT('Ctrl Pts',(24.4185014959392,-0.992429524077198,
26.6454377623415));
#43157=CARTESIAN_POINT('Ctrl Pts',(24.4278332223638,-0.992555410679472,
26.4999811860602));
#43158=CARTESIAN_POINT('Origin',(18.,0.,26.5));
#43159=CARTESIAN_POINT('',(24.9721667776362,-0.99251277648446,26.5000582001704));
#43160=CARTESIAN_POINT('',(24.8278332223638,-0.992417933442169,26.5000080784797));
#43161=CARTESIAN_POINT('',(18.,-0.9925,26.5));
#43162=CARTESIAN_POINT('Ctrl Pts',(24.9721667776362,-0.99251277648446,26.5000582001704));
#43163=CARTESIAN_POINT('Ctrl Pts',(24.9617183667645,-0.99255659087909,26.6628621040987));
#43164=CARTESIAN_POINT('Ctrl Pts',(24.9512699558928,-0.951915057130168,
26.8255137793979));
#43165=CARTESIAN_POINT('Ctrl Pts',(24.9408215450211,-0.874820116044522,
26.9691019472486));
#43166=CARTESIAN_POINT('Ctrl Pts',(24.9302360095206,-0.796713383279699,
27.1145745618789));
#43167=CARTESIAN_POINT('Ctrl Pts',(24.91965047402,-0.681190137660315,27.240480007797));
#43168=CARTESIAN_POINT('Ctrl Pts',(24.9090649385195,-0.543356244838065,
27.3306849446437));
#43169=CARTESIAN_POINT('Ctrl Pts',(24.8984794030189,-0.40552235201583,27.4208898814904));
#43170=CARTESIAN_POINT('Ctrl Pts',(24.8878938675184,-0.24537781199073,27.4753943092657));
#43171=CARTESIAN_POINT('Ctrl Pts',(24.8773083320179,-0.0806281138645919,
27.4889319986692));
#43172=CARTESIAN_POINT('Ctrl Pts',(24.8667227965174,0.0841215842615465,
27.5024696880728));
#43173=CARTESIAN_POINT('Ctrl Pts',(24.8561372610168,0.253476440488729,27.4750406391045));
#43174=CARTESIAN_POINT('Ctrl Pts',(24.8455517255163,0.403905693619946,27.4077887430593));
#43175=CARTESIAN_POINT('Ctrl Pts',(24.8243806545152,0.704764199882382,27.273284950969));
#43176=CARTESIAN_POINT('Ctrl Pts',(24.8032095835142,0.929920293760979,26.9794897705714));
#43177=CARTESIAN_POINT('Ctrl Pts',(24.7820385125131,0.981581218735328,26.6540081893599));
#43178=CARTESIAN_POINT('Ctrl Pts',(24.7714529770126,1.0074116812225,26.4912673987541));
#43179=CARTESIAN_POINT('Ctrl Pts',(24.760867441512,0.989868351483619,26.320605007945));
#43180=CARTESIAN_POINT('Ctrl Pts',(24.7502819060115,0.933964243597536,26.1650400286325));
#43181=CARTESIAN_POINT('Ctrl Pts',(24.739696370511,0.878060135711457,26.0094750493199));
#43182=CARTESIAN_POINT('Ctrl Pts',(24.7291108350104,0.783795249678182,25.8690074815041));
#43183=CARTESIAN_POINT('Ctrl Pts',(24.7185252995099,0.660857833523188,25.759364860452));
#43184=CARTESIAN_POINT('Ctrl Pts',(24.7079397640094,0.537920417368194,25.6497222393999));
#43185=CARTESIAN_POINT('Ctrl Pts',(24.6973542285088,0.386310471091475,25.5709045651114));
#43186=CARTESIAN_POINT('Ctrl Pts',(24.6867686930083,0.225533816953791,25.5333038896536));
#43187=CARTESIAN_POINT('Ctrl Pts',(24.6761831575078,0.0647571628160969,
25.4957032141958));
#43188=CARTESIAN_POINT('Ctrl Pts',(24.6655976220072,-0.10518619918257,25.4993195375686));
#43189=CARTESIAN_POINT('Ctrl Pts',(24.6550120865067,-0.264162719082483,
25.5432895733726));
#43190=CARTESIAN_POINT('Ctrl Pts',(24.6444265510062,-0.423139238982396,
25.5872596091765));
#43191=CARTESIAN_POINT('Ctrl Pts',(24.6338410155057,-0.571148916783561,
25.6715833574117));
#43192=CARTESIAN_POINT('Ctrl Pts',(24.6232554800051,-0.689810539973791,
25.7862078642024));
#43193=CARTESIAN_POINT('Ctrl Pts',(24.6126699445046,-0.808472163164022,
25.9008323709931));
#43194=CARTESIAN_POINT('Ctrl Pts',(24.602084409004,-0.897785731743322,26.0457576363393));
#43195=CARTESIAN_POINT('Ctrl Pts',(24.5914988735035,-0.947124736504967,
26.2032093172979));
#43196=CARTESIAN_POINT('Ctrl Pts',(24.5850548415477,-0.97716026218375,26.299059325409));
#43197=CARTESIAN_POINT('Ctrl Pts',(24.578610809592,-0.992381750402969,26.3995514552194));
#43198=CARTESIAN_POINT('Ctrl Pts',(24.5721667776362,-0.992469460302077,
26.5000248288071));
#43199=CARTESIAN_POINT('Ctrl Pts',(24.4278332223638,-0.992555410679472,
26.4999811860602));
#43200=CARTESIAN_POINT('Ctrl Pts',(24.4291106988375,-0.992572644057889,
26.4800687555315));
#43201=CARTESIAN_POINT('Ctrl Pts',(24.4303881753112,-0.991985754731688,
26.460157339995));
#43202=CARTESIAN_POINT('Ctrl Pts',(24.4316656517849,-0.990787863821187,
26.4402827510437));
#43203=CARTESIAN_POINT('Ctrl Pts',(24.4422748546831,-0.980839604122276,
26.2752280114485));
#43204=CARTESIAN_POINT('Ctrl Pts',(24.4528840575814,-0.928750617269329,
26.1127131982961));
#43205=CARTESIAN_POINT('Ctrl Pts',(24.4634932604797,-0.840896177802749,
25.972628822294));
#43206=CARTESIAN_POINT('Ctrl Pts',(24.4741024633779,-0.753041738336164,
25.8325444462919));
#43207=CARTESIAN_POINT('Ctrl Pts',(24.4847116662762,-0.629421846255941,
25.7148905074399));
#43208=CARTESIAN_POINT('Ctrl Pts',(24.4953208691745,-0.485166585640924,
25.6340669049541));
#43209=CARTESIAN_POINT('Ctrl Pts',(24.5059300720728,-0.340911325025915,
25.5532433024682));
#43210=CARTESIAN_POINT('Ctrl Pts',(24.516539274971,-0.176020695876084,25.5092500363485));
#43211=CARTESIAN_POINT('Ctrl Pts',(24.5271484778693,-0.0106759897366275,
25.5074715297981));
#43212=CARTESIAN_POINT('Ctrl Pts',(24.5377576807676,0.154668716402848,25.5056930232476));
#43213=CARTESIAN_POINT('Ctrl Pts',(24.5483668836659,0.320467499531954,25.5461292762665));
#43214=CARTESIAN_POINT('Ctrl Pts',(24.5589760865641,0.466427917336639,25.6238312155485));
#43215=CARTESIAN_POINT('Ctrl Pts',(24.5695852894624,0.612388335141316,25.7015331548305));
#43216=CARTESIAN_POINT('Ctrl Pts',(24.5801944923606,0.738510387621547,25.8165007803756));
#43217=CARTESIAN_POINT('Ctrl Pts',(24.5908036952589,0.829357746318288,25.954662976188));
#43218=CARTESIAN_POINT('Ctrl Pts',(24.6014128981572,0.920205105015029,26.0928251720005));
#43219=CARTESIAN_POINT('Ctrl Pts',(24.6120221010555,0.97577776992828,26.2541819380803));
#43220=CARTESIAN_POINT('Ctrl Pts',(24.6226313039538,0.98927409224187,26.4189844994011));
#43221=CARTESIAN_POINT('Ctrl Pts',(24.6332405068521,1.00277041455546,26.583787060722));
#43222=CARTESIAN_POINT('Ctrl Pts',(24.6438497097503,0.974190394269388,26.7520354172838));
#43223=CARTESIAN_POINT('Ctrl Pts',(24.6544589126486,0.907031996821316,26.9031373186156));
#43224=CARTESIAN_POINT('Ctrl Pts',(24.6650681155468,0.839873599373236,27.0542392199475));
#43225=CARTESIAN_POINT('Ctrl Pts',(24.6756773184451,0.734136824763144,27.1881946660494));
#43226=CARTESIAN_POINT('Ctrl Pts',(24.6862865213434,0.60276300681002,27.2886085838612));
#43227=CARTESIAN_POINT('Ctrl Pts',(24.6968957242417,0.471389188856896,27.389022501673));
#43228=CARTESIAN_POINT('Ctrl Pts',(24.7075049271399,0.31437832756074,27.4558948911948));
#43229=CARTESIAN_POINT('Ctrl Pts',(24.7181141300382,0.150947294031265,27.4810411078762));
#43230=CARTESIAN_POINT('Ctrl Pts',(24.7287233329365,-0.0124837394982006,
27.5061873245576));
#43231=CARTESIAN_POINT('Ctrl Pts',(24.7393325358348,-0.182334945260984,
27.4896073683986));
#43232=CARTESIAN_POINT('Ctrl Pts',(24.749941738733,-0.337817896889458,27.4333304931585));
#43233=CARTESIAN_POINT('Ctrl Pts',(24.7605509416313,-0.493300848517933,
27.3770536179183));
#43234=CARTESIAN_POINT('Ctrl Pts',(24.7711601445296,-0.634415546012099,
27.281079823597));
#43235=CARTESIAN_POINT('Ctrl Pts',(24.7817693474278,-0.743890681316928,
27.1571555334684));
#43236=CARTESIAN_POINT('Ctrl Pts',(24.7923785503261,-0.853365816621756,
27.0332312433397));
#43237=CARTESIAN_POINT('Ctrl Pts',(24.8029877532244,-0.931201389737248,
26.8813564574038));
#43238=CARTESIAN_POINT('Ctrl Pts',(24.8135969561227,-0.967870950302176,
26.7201194323076));
#43239=CARTESIAN_POINT('Ctrl Pts',(24.818342378203,-0.984272987670209,26.6479992413373));
#43240=CARTESIAN_POINT('Ctrl Pts',(24.8230878002834,-0.992438898982193,
26.5740059376434));
#43241=CARTESIAN_POINT('Ctrl Pts',(24.8278332223638,-0.992417933442169,
26.5000080784797));
#43242=CARTESIAN_POINT('Origin',(18.,0.,26.5));
#43243=CARTESIAN_POINT('',(25.3721667776362,-0.992387361158253,26.5001400376411));
#43244=CARTESIAN_POINT('',(25.2278332223638,-0.99258529737825,26.5000026553357));
#43245=CARTESIAN_POINT('',(18.,-0.9925,26.5));
#43246=CARTESIAN_POINT('Ctrl Pts',(25.3721667776362,-0.992387361158253,
26.5001400376411));
#43247=CARTESIAN_POINT('Ctrl Pts',(25.3659969949381,-0.992306742378732,
26.5965231262208));
#43248=CARTESIAN_POINT('Ctrl Pts',(25.35982721224,-0.978386398123005,26.6928893412557));
#43249=CARTESIAN_POINT('Ctrl Pts',(25.3536574295418,-0.950854057019746,
26.7848684754603));
#43250=CARTESIAN_POINT('Ctrl Pts',(25.3430718940413,-0.903616643901465,
26.9426776622776));
#43251=CARTESIAN_POINT('Ctrl Pts',(25.3324863585408,-0.81631029856865,27.0875728257978));
#43252=CARTESIAN_POINT('Ctrl Pts',(25.3219008230402,-0.699077270305875,
27.2041153036819));
#43253=CARTESIAN_POINT('Ctrl Pts',(25.3113152875397,-0.581844242043086,
27.320657781566));
#43254=CARTESIAN_POINT('Ctrl Pts',(25.3007297520392,-0.434684530850328,
27.408847573814));
#43255=CARTESIAN_POINT('Ctrl Pts',(25.2901442165386,-0.276325837818277,
27.454392080184));
#43256=CARTESIAN_POINT('Ctrl Pts',(25.2689731455376,0.0403915482457888,
27.5454810929239));
#43257=CARTESIAN_POINT('Ctrl Pts',(25.2478020745365,0.40190486166702,27.465988962152));
#43258=CARTESIAN_POINT('Ctrl Pts',(25.2266310035354,0.6511968846158,27.2504417557882));
#43259=CARTESIAN_POINT('Ctrl Pts',(25.2160454680349,0.77584289609019,27.1426681526063));
#43260=CARTESIAN_POINT('Ctrl Pts',(25.2054599325344,0.872433584946467,27.0008807805265));
#43261=CARTESIAN_POINT('Ctrl Pts',(25.1948743970339,0.929964336340446,26.8459099938888));
#43262=CARTESIAN_POINT('Ctrl Pts',(25.1842888615333,0.987495087734426,26.6909392072512));
#43263=CARTESIAN_POINT('Ctrl Pts',(25.1737033260328,1.00596590166611,26.5227850060558));
#43264=CARTESIAN_POINT('Ctrl Pts',(25.1631177905322,0.982646449396851,26.3597165670864));
#43265=CARTESIAN_POINT('Ctrl Pts',(25.1525322550317,0.95932699712759,26.196648128117));
#43266=CARTESIAN_POINT('Ctrl Pts',(25.1419467195312,0.89421727865738,26.0386654513737));
#43267=CARTESIAN_POINT('Ctrl Pts',(25.1313611840307,0.795532045788893,25.9062865704134));
#43268=CARTESIAN_POINT('Ctrl Pts',(25.1207756485301,0.696846812920429,25.7739076894532));
#43269=CARTESIAN_POINT('Ctrl Pts',(25.1101901130296,0.564586065653703,25.667132604276));
#43270=CARTESIAN_POINT('Ctrl Pts',(25.099604577529,0.414699306759659,25.5982787195903));
#43271=CARTESIAN_POINT('Ctrl Pts',(25.0890190420285,0.26481254786558,25.5294248349045));
#43272=CARTESIAN_POINT('Ctrl Pts',(25.078433506528,0.0972997773441754,25.4984921507102));
#43273=CARTESIAN_POINT('Ctrl Pts',(25.0678479710275,-0.0673058880772577,
25.5096426343912));
#43274=CARTESIAN_POINT('Ctrl Pts',(25.0572624355269,-0.231911553498672,
25.5207931180722));
#43275=CARTESIAN_POINT('Ctrl Pts',(25.0466769000264,-0.393610113820115,
25.5740267696286));
#43276=CARTESIAN_POINT('Ctrl Pts',(25.0360913645259,-0.532820336822596,
25.6626037589608));
#43277=CARTESIAN_POINT('Ctrl Pts',(25.0255058290253,-0.672030559825076,
25.7511807482929));
#43278=CARTESIAN_POINT('Ctrl Pts',(25.0149202935248,-0.788752445508594,
25.8751010754009));
#43279=CARTESIAN_POINT('Ctrl Pts',(25.0043347580243,-0.868585547923311,
26.0194826328588));
#43280=CARTESIAN_POINT('Ctrl Pts',(24.9937492225237,-0.948418650338028,
26.1638641903168));
#43281=CARTESIAN_POINT('Ctrl Pts',(24.9831636870232,-0.991362969483945,
26.3287069781248));
#43282=CARTESIAN_POINT('Ctrl Pts',(24.9725781515227,-0.992490019101772,
26.4936482637001));
#43283=CARTESIAN_POINT('Ctrl Pts',(24.9724410268938,-0.992504618860141,
26.4957849069112));
#43284=CARTESIAN_POINT('Ctrl Pts',(24.972303902265,-0.992512201465668,26.4979215666506));
#43285=CARTESIAN_POINT('Ctrl Pts',(24.9721667776362,-0.99251277648446,26.5000582001704));
#43286=CARTESIAN_POINT('Ctrl Pts',(24.8278332223638,-0.992417933442169,
26.5000080784797));
#43287=CARTESIAN_POINT('Ctrl Pts',(24.8336970031817,-0.992392026930725,
26.408571064073));
#43288=CARTESIAN_POINT('Ctrl Pts',(24.8395607839996,-0.979865717223218,
26.3171270939968));
#43289=CARTESIAN_POINT('Ctrl Pts',(24.8454245648175,-0.954931924032951,
26.2292016222704));
#43290=CARTESIAN_POINT('Ctrl Pts',(24.8560337677157,-0.909819789184432,
26.0701201015859));
#43291=CARTESIAN_POINT('Ctrl Pts',(24.866642970614,-0.824091971473027,25.9225563244732));
#43292=CARTESIAN_POINT('Ctrl Pts',(24.8772521735123,-0.70824086874865,25.8045709146488));
#43293=CARTESIAN_POINT('Ctrl Pts',(24.8878613764106,-0.592389766024272,
25.6865855048243));
#43294=CARTESIAN_POINT('Ctrl Pts',(24.8984705793089,-0.446415378286923,
25.5981784622881));
#43295=CARTESIAN_POINT('Ctrl Pts',(24.9090797822071,-0.288183800730977,
25.5501701005367));
#43296=CARTESIAN_POINT('Ctrl Pts',(24.9196889851054,-0.129952223175031,
25.5021617387853));
#43297=CARTESIAN_POINT('Ctrl Pts',(24.9302981880037,0.0405365441995126,
25.4945520578188));
#43298=CARTESIAN_POINT('Ctrl Pts',(24.9409073909019,0.202416042593281,25.5282724216021));
#43299=CARTESIAN_POINT('Ctrl Pts',(24.9515165938002,0.364295540987049,25.5619927853854));
#43300=CARTESIAN_POINT('Ctrl Pts',(24.9621257966985,0.517565770400043,25.6370431939185));
#43301=CARTESIAN_POINT('Ctrl Pts',(24.9727349995968,0.643467683086959,25.7442380786643));
#43302=CARTESIAN_POINT('Ctrl Pts',(24.983344202495,0.769369595773882,25.8514329634102));
#43303=CARTESIAN_POINT('Ctrl Pts',(24.9939534053933,0.867903191734725,25.9907723243687));
#43304=CARTESIAN_POINT('Ctrl Pts',(25.0045626082916,0.927008748489623,26.145202140449));
#43305=CARTESIAN_POINT('Ctrl Pts',(25.0151718111898,0.986114305244514,26.2996319565293));
#43306=CARTESIAN_POINT('Ctrl Pts',(25.0257810140881,1.00579182279347,26.4691522277313));
#43307=CARTESIAN_POINT('Ctrl Pts',(25.0363902169864,0.983632930687616,26.6330150314256));
#43308=CARTESIAN_POINT('Ctrl Pts',(25.0469994198846,0.961474038581758,26.7968778351198));
#43309=CARTESIAN_POINT('Ctrl Pts',(25.0576086227829,0.897478736821098,26.9550831713063));
#43310=CARTESIAN_POINT('Ctrl Pts',(25.0682178256812,0.799479537471402,27.0882679747214));
#43311=CARTESIAN_POINT('Ctrl Pts',(25.0788270285795,0.701480338121717,27.2214527781364));
#43312=CARTESIAN_POINT('Ctrl Pts',(25.0894362314777,0.569477241183014,27.3296170487802));
#43313=CARTESIAN_POINT('Ctrl Pts',(25.100045434376,0.419626367824316,27.3995223467735));
#43314=CARTESIAN_POINT('Ctrl Pts',(25.1106546372743,0.269775494465601,27.4694276447668));
#43315=CARTESIAN_POINT('Ctrl Pts',(25.1212638401726,0.102076844686887,27.5010739701096));
#43316=CARTESIAN_POINT('Ctrl Pts',(25.1318730430708,-0.0629446107456808,
27.4905880661992));
#43317=CARTESIAN_POINT('Ctrl Pts',(25.1424822459691,-0.22796606617824,27.4801021622889));
#43318=CARTESIAN_POINT('Ctrl Pts',(25.1530914488674,-0.390310327264653,
27.4274840291254));
#43319=CARTESIAN_POINT('Ctrl Pts',(25.1637006517656,-0.530107757503696,
27.3391737045169));
#43320=CARTESIAN_POINT('Ctrl Pts',(25.1743098546639,-0.66990518774273,27.2508633799084));
#43321=CARTESIAN_POINT('Ctrl Pts',(25.1849190575622,-0.787155787134396,
27.126860863855));
#43322=CARTESIAN_POINT('Ctrl Pts',(25.1955282604605,-0.867509021980289,
26.9823430705432));
#43323=CARTESIAN_POINT('Ctrl Pts',(25.2061374633587,-0.947862256826192,
26.8378252772315));
#43324=CARTESIAN_POINT('Ctrl Pts',(25.216746666257,-0.991318127126315,26.6727922066615));
#43325=CARTESIAN_POINT('Ctrl Pts',(25.2273558691553,-0.992557982618985,
26.5074425840666));
#43326=CARTESIAN_POINT('Ctrl Pts',(25.2275149868914,-0.99257657807814,26.504962656227));
#43327=CARTESIAN_POINT('Ctrl Pts',(25.2276741046276,-0.992585677358007,
26.5024826571814));
#43328=CARTESIAN_POINT('Ctrl Pts',(25.2278332223638,-0.99258529737825,26.5000026553357));
#43329=CARTESIAN_POINT('Origin',(18.,0.,26.5));
#43330=CARTESIAN_POINT('',(25.7721667776362,-0.9921765548274,26.4993478195649));
#43331=CARTESIAN_POINT('',(25.6278332223638,-0.99242346011951,26.4999876204483));
#43332=CARTESIAN_POINT('',(18.,-0.9925,26.5));
#43333=CARTESIAN_POINT('Ctrl Pts',(25.7721667776362,-0.9921765548274,26.4993478195649));
#43334=CARTESIAN_POINT('Ctrl Pts',(25.7702756231116,-0.992198777860299,
26.528814111564));
#43335=CARTESIAN_POINT('Ctrl Pts',(25.7683844685871,-0.990919946850656,
26.5583087935269));
#43336=CARTESIAN_POINT('Ctrl Pts',(25.7664933140626,-0.988327533930795,
26.5877272816407));
#43337=CARTESIAN_POINT('Ctrl Pts',(25.755907778562,-0.973816779447677,26.7523941273481));
#43338=CARTESIAN_POINT('Ctrl Pts',(25.7453222430615,-0.918150438689142,
26.9146737579895));
#43339=CARTESIAN_POINT('Ctrl Pts',(25.734736707561,-0.826434186032542,27.0515675368345));
#43340=CARTESIAN_POINT('Ctrl Pts',(25.7135656365599,-0.643001680719363,
27.3253550945245));
#43341=CARTESIAN_POINT('Ctrl Pts',(25.6923945655588,-0.315369527813967,
27.4975992450292));
#43342=CARTESIAN_POINT('Ctrl Pts',(25.6712234945578,0.0141607649234293,
27.4934886431632));
#43343=CARTESIAN_POINT('Ctrl Pts',(25.6606379590572,0.178925911292108,27.4914333422301));
#43344=CARTESIAN_POINT('Ctrl Pts',(25.6500524235567,0.344165592618783,27.4452893532044));
#43345=CARTESIAN_POINT('Ctrl Pts',(25.6394668880562,0.488039692138768,27.3638892577079));
#43346=CARTESIAN_POINT('Ctrl Pts',(25.6288813525557,0.631913791658785,27.2824891622114));
#43347=CARTESIAN_POINT('Ctrl Pts',(25.6182958170551,0.754422309372096,27.1658329602441));
#43348=CARTESIAN_POINT('Ctrl Pts',(25.6077102815546,0.841702064697562,27.0261284257574));
#43349=CARTESIAN_POINT('Ctrl Pts',(25.5971247460541,0.928981820023017,26.8864238912708));
#43350=CARTESIAN_POINT('Ctrl Pts',(25.5865392105535,0.981032812960631,26.7236710242649));
#43351=CARTESIAN_POINT('Ctrl Pts',(25.575953675053,0.990910358314731,26.5588517978137));
#43352=CARTESIAN_POINT('Ctrl Pts',(25.5653681395525,1.00078790366883,26.3940325713625));
#43353=CARTESIAN_POINT('Ctrl Pts',(25.5547826040519,0.968492001439414,26.227146985466));
#43354=CARTESIAN_POINT('Ctrl Pts',(25.5441970685514,0.898277408587982,26.0778928100537));
#43355=CARTESIAN_POINT('Ctrl Pts',(25.5336115330509,0.82806281573653,25.9286386346413));
#43356=CARTESIAN_POINT('Ctrl Pts',(25.5230259975503,0.719929532263041,25.7970158697132));
#43357=CARTESIAN_POINT('Ctrl Pts',(25.5124404620498,0.586893434433857,25.6994415131927));
#43358=CARTESIAN_POINT('Ctrl Pts',(25.5018549265493,0.453857336604717,25.6018671566723));
#43359=CARTESIAN_POINT('Ctrl Pts',(25.4912693910487,0.295918424419905,25.5383412085594));
#43360=CARTESIAN_POINT('Ctrl Pts',(25.4806838555482,0.132391755440172,25.5163321704302));
#43361=CARTESIAN_POINT('Ctrl Pts',(25.4700983200477,-0.0311349135395798,
25.494323132301));
#43362=CARTESIAN_POINT('Ctrl Pts',(25.4595127845471,-0.200249339314248,
25.5138310041554));
#43363=CARTESIAN_POINT('Ctrl Pts',(25.4489272490466,-0.354349175992256,
25.572759763783));
#43364=CARTESIAN_POINT('Ctrl Pts',(25.4383417135461,-0.508449012670264,
25.6316885234106));
#43365=CARTESIAN_POINT('Ctrl Pts',(25.4277561780455,-0.647534260251607,
25.7300381708114));
#43366=CARTESIAN_POINT('Ctrl Pts',(25.417170642545,-0.754711704727708,25.8554171695454));
#43367=CARTESIAN_POINT('Ctrl Pts',(25.4065851070445,-0.861889149203809,
25.9807961682795));
#43368=CARTESIAN_POINT('Ctrl Pts',(25.3959995715439,-0.937158790574664,
26.1332045183467));
#43369=CARTESIAN_POINT('Ctrl Pts',(25.3854140360434,-0.971209370808219,
26.2947702984376));
#43370=CARTESIAN_POINT('Ctrl Pts',(25.380998283241,-0.985413559635735,26.3621674127521));
#43371=CARTESIAN_POINT('Ctrl Pts',(25.3765825304386,-0.992445060532609,
26.4311580468119));
#43372=CARTESIAN_POINT('Ctrl Pts',(25.3721667776362,-0.992387361158253,
26.5001400376411));
#43373=CARTESIAN_POINT('Ctrl Pts',(25.2278332223638,-0.99258529737825,26.5000026553357));
#43374=CARTESIAN_POINT('Ctrl Pts',(25.2382833075259,-0.992560342141212,
26.3371281002211));
#43375=CARTESIAN_POINT('Ctrl Pts',(25.248733392688,-0.951649173128032,26.1742414680339));
#43376=CARTESIAN_POINT('Ctrl Pts',(25.2591834778501,-0.874644658184562,
26.0307202723029));
#43377=CARTESIAN_POINT('Ctrl Pts',(25.2697926807484,-0.796467637572248,
25.8850137577537));
#43378=CARTESIAN_POINT('Ctrl Pts',(25.2804018836467,-0.681089755662396,
25.7592669032749));
#43379=CARTESIAN_POINT('Ctrl Pts',(25.2910110865449,-0.542632340541926,
25.6688701160972));
#43380=CARTESIAN_POINT('Ctrl Pts',(25.3016202894432,-0.404174925421455,
25.5784733289195));
#43381=CARTESIAN_POINT('Ctrl Pts',(25.3122294923414,-0.242637977090366,
25.5234266090428));
#43382=CARTESIAN_POINT('Ctrl Pts',(25.3228386952397,-0.0777923234385866,
25.5104672338259));
#43383=CARTESIAN_POINT('Ctrl Pts',(25.333447898138,0.0870533302131832,25.4975078586089));
#43384=CARTESIAN_POINT('Ctrl Pts',(25.3440571010363,0.255207689185642,25.5266358280516));
#43385=CARTESIAN_POINT('Ctrl Pts',(25.3546663039346,0.406090007559484,25.5942861121311));
#43386=CARTESIAN_POINT('Ctrl Pts',(25.3652755068328,0.556972325933344,25.6619363962105));
#43387=CARTESIAN_POINT('Ctrl Pts',(25.3758847097311,0.690582603708582,25.7681089949267));
#43388=CARTESIAN_POINT('Ctrl Pts',(25.3864939126294,0.790568013661987,25.8998092330827));
#43389=CARTESIAN_POINT('Ctrl Pts',(25.3971031155276,0.890553423615392,26.0315094712387));
#43390=CARTESIAN_POINT('Ctrl Pts',(25.4077123184259,0.956913965746965,26.1887373488345));
#43391=CARTESIAN_POINT('Ctrl Pts',(25.4183215213242,0.98152764152502,26.3522494337047));
#43392=CARTESIAN_POINT('Ctrl Pts',(25.4289307242225,1.00614131730307,26.5157615185749));
#43393=CARTESIAN_POINT('Ctrl Pts',(25.4395399271207,0.989008126727611,26.6855578107195));
#43394=CARTESIAN_POINT('Ctrl Pts',(25.450149130019,0.932225035016547,26.8408566047574));
#43395=CARTESIAN_POINT('Ctrl Pts',(25.4607583329173,0.875441943305496,26.9961553987952));
#43396=CARTESIAN_POINT('Ctrl Pts',(25.4713675358156,0.779008950458864,27.1369566947264));
#43397=CARTESIAN_POINT('Ctrl Pts',(25.4819767387138,0.654728681970098,27.2460275423359));
#43398=CARTESIAN_POINT('Ctrl Pts',(25.4925859416121,0.530448413481304,27.3550983899455));
#43399=CARTESIAN_POINT('Ctrl Pts',(25.5031951445104,0.378320869350364,27.4324387892333));
#43400=CARTESIAN_POINT('Ctrl Pts',(25.5138043474086,0.216965241801435,27.4685828951456));
#43401=CARTESIAN_POINT('Ctrl Pts',(25.5244135503069,0.0556096142525066,
27.5047270010579));
#43402=CARTESIAN_POINT('Ctrl Pts',(25.5350227532052,-0.11497409671441,27.4996748135948));
#43403=CARTESIAN_POINT('Ctrl Pts',(25.5456319561035,-0.273907811964552,
27.4540446800138));
#43404=CARTESIAN_POINT('Ctrl Pts',(25.5562411590017,-0.432841527214676,
27.4084145464327));
#43405=CARTESIAN_POINT('Ctrl Pts',(25.5668503619,-0.580125246748027,27.3222064667338));
#43406=CARTESIAN_POINT('Ctrl Pts',(25.5774595647983,-0.697732623652709,
27.2059716189829));
#43407=CARTESIAN_POINT('Ctrl Pts',(25.5880687676965,-0.815340000557391,
27.0897367712321));
#43408=CARTESIAN_POINT('Ctrl Pts',(25.5986779705948,-0.903271034833404,
26.9434751554294));
#43409=CARTESIAN_POINT('Ctrl Pts',(25.6092871734931,-0.950763672578241,
26.7850880211867));
#43410=CARTESIAN_POINT('Ctrl Pts',(25.6154691897833,-0.978437783726829,
26.692795334032));
#43411=CARTESIAN_POINT('Ctrl Pts',(25.6216512060736,-0.992381320457257,
26.5963855119862));
#43412=CARTESIAN_POINT('Ctrl Pts',(25.6278332223638,-0.99242346011951,26.4999876204483));
#43413=CARTESIAN_POINT('Origin',(18.,0.,26.5));
#43414=CARTESIAN_POINT('',(26.1721667776362,-0.993011273520018,26.5001944908134));
#43415=CARTESIAN_POINT('',(26.0278332223638,-0.992541444115404,26.5000219547962));
#43416=CARTESIAN_POINT('',(18.,-0.9925,26.5));
#43417=CARTESIAN_POINT('Ctrl Pts',(26.1721667776362,-0.993011273520018,
26.5001944908134));
#43418=CARTESIAN_POINT('Ctrl Pts',(26.1533831802842,-0.990681442009467,
26.7921974358648));
#43419=CARTESIAN_POINT('Ctrl Pts',(26.1345995829321,-0.855424830611663,
27.0830337592609));
#43420=CARTESIAN_POINT('Ctrl Pts',(26.1158159855801,-0.629544085260756,
27.2686969039528));
#43421=CARTESIAN_POINT('Ctrl Pts',(26.1052304500796,-0.502248519667636,
27.3733277567359));
#43422=CARTESIAN_POINT('Ctrl Pts',(26.0946449145791,-0.346171548785687,
27.4445565592068));
#43423=CARTESIAN_POINT('Ctrl Pts',(26.0840593790785,-0.183705030547387,
27.4750588526323));
#43424=CARTESIAN_POINT('Ctrl Pts',(26.073473843578,-0.0212385123090691,
27.5055611460579));
#43425=CARTESIAN_POINT('Ctrl Pts',(26.0628883080775,0.147617553285602,27.495336930438));
#43426=CARTESIAN_POINT('Ctrl Pts',(26.0523027725769,0.304395987274318,27.4447838493567));
#43427=CARTESIAN_POINT('Ctrl Pts',(26.0417172370764,0.461174421263017,27.3942307682754));
#43428=CARTESIAN_POINT('Ctrl Pts',(26.0311317015759,0.605875223645765,27.3033488217328));
#43429=CARTESIAN_POINT('Ctrl Pts',(26.0205461660753,0.719664201221994,27.1837034248472));
#43430=CARTESIAN_POINT('Ctrl Pts',(26.0099606305748,0.833453178798223,27.0640580279616));
#43431=CARTESIAN_POINT('Ctrl Pts',(25.9993750950743,0.916330331567933,26.915649180733));
#43432=CARTESIAN_POINT('Ctrl Pts',(25.9887895595738,0.958852278036404,26.7562792338966));
#43433=CARTESIAN_POINT('Ctrl Pts',(25.9782040240732,1.00137422450488,26.5969092870601));
#43434=CARTESIAN_POINT('Ctrl Pts',(25.9676184885727,1.00354096467211,26.4265782406157));
#43435=CARTESIAN_POINT('Ctrl Pts',(25.9570329530721,0.964721792019372,26.2662272832873));
#43436=CARTESIAN_POINT('Ctrl Pts',(25.9464474175716,0.925902619366637,26.1058763259588));
#43437=CARTESIAN_POINT('Ctrl Pts',(25.9358618820711,0.846097533893935,25.9555054577463));
#43438=CARTESIAN_POINT('Ctrl Pts',(25.9252763465706,0.73525991827821,25.8332745556996));
#43439=CARTESIAN_POINT('Ctrl Pts',(25.91469081107,0.624422302662473,25.7110436536529));
#43440=CARTESIAN_POINT('Ctrl Pts',(25.9041052755695,0.482552156903705,25.616952717772));
#43441=CARTESIAN_POINT('Ctrl Pts',(25.8935197400689,0.326751952924584,25.5626788394154));
#43442=CARTESIAN_POINT('Ctrl Pts',(25.8829342045684,0.170951748945481,25.5084049610588));
#43443=CARTESIAN_POINT('Ctrl Pts',(25.8723486690679,0.00122148674602748,
25.4939481402265));
#43444=CARTESIAN_POINT('Ctrl Pts',(25.8617631335674,-0.161535973435497,
25.5207232708255));
#43445=CARTESIAN_POINT('Ctrl Pts',(25.8511775980668,-0.324293433617022,
25.5474984014245));
#43446=CARTESIAN_POINT('Ctrl Pts',(25.8405920625663,-0.480078091780619,
25.6155054834548));
#43447=CARTESIAN_POINT('Ctrl Pts',(25.8300065270658,-0.610251400009936,
25.7170823159535));
#43448=CARTESIAN_POINT('Ctrl Pts',(25.8194209915652,-0.740424708239253,
25.8186591484523));
#43449=CARTESIAN_POINT('Ctrl Pts',(25.8088354560647,-0.84498666653429,25.9538057314195));
#43450=CARTESIAN_POINT('Ctrl Pts',(25.7982499205642,-0.910590061577954,
26.1049060532897));
#43451=CARTESIAN_POINT('Ctrl Pts',(25.7895555395882,-0.964473108855015,
26.2290116088253));
#43452=CARTESIAN_POINT('Ctrl Pts',(25.7808611586122,-0.992074386806777,
26.3638796887133));
#43453=CARTESIAN_POINT('Ctrl Pts',(25.7721667776362,-0.9921765548274,26.4993478195649));
#43454=CARTESIAN_POINT('Ctrl Pts',(25.6278332223638,-0.99242346011951,26.4999876204483));
#43455=CARTESIAN_POINT('Ctrl Pts',(25.6322604089718,-0.992453637999935,
26.4309532739789));
#43456=CARTESIAN_POINT('Ctrl Pts',(25.6366875955799,-0.985354402214821,
26.361925046141));
#43457=CARTESIAN_POINT('Ctrl Pts',(25.6411147821879,-0.971063013632482,
26.2944194453005));
#43458=CARTESIAN_POINT('Ctrl Pts',(25.6517239850862,-0.936815475728224,
26.1326506563395));
#43459=CARTESIAN_POINT('Ctrl Pts',(25.6623331879844,-0.861266158706048,
25.9796257311001));
#43460=CARTESIAN_POINT('Ctrl Pts',(25.6729423908827,-0.753661693496502,
25.8540736940781));
#43461=CARTESIAN_POINT('Ctrl Pts',(25.683551593781,-0.646057228286968,25.7285216570561));
#43462=CARTESIAN_POINT('Ctrl Pts',(25.6941607966793,-0.506397614890069,
25.6304425082515));
#43463=CARTESIAN_POINT('Ctrl Pts',(25.7047699995776,-0.351776070742455,
25.571840349425));
#43464=CARTESIAN_POINT('Ctrl Pts',(25.7153792024758,-0.197154526594824,
25.5132381905986));
#43465=CARTESIAN_POINT('Ctrl Pts',(25.7259884053741,-0.0275710516964692,
25.4941130217504));
#43466=CARTESIAN_POINT('Ctrl Pts',(25.7365976082724,0.136218695723237,25.5168056103299));
#43467=CARTESIAN_POINT('Ctrl Pts',(25.7472068111706,0.300008443142944,25.5394981989094));
#43468=CARTESIAN_POINT('Ctrl Pts',(25.7578160140689,0.458004463084008,25.6040085449167));
#43469=CARTESIAN_POINT('Ctrl Pts',(25.7684252169672,0.59086930886453,25.7024410988939));
#43470=CARTESIAN_POINT('Ctrl Pts',(25.7790344198655,0.723734154645037,25.8008736528711));
#43471=CARTESIAN_POINT('Ctrl Pts',(25.7896436227637,0.831467826265013,25.9332284148183));
#43472=CARTESIAN_POINT('Ctrl Pts',(25.800252825662,0.900884585808005,26.0833062227837));
#43473=CARTESIAN_POINT('Ctrl Pts',(25.8108620285603,0.970301345351009,26.2333840307492));
#43474=CARTESIAN_POINT('Ctrl Pts',(25.8214712314585,1.00140119281702,26.401184884733));
#43475=CARTESIAN_POINT('Ctrl Pts',(25.8320804343568,0.9903777559402,26.5661713046231));
#43476=CARTESIAN_POINT('Ctrl Pts',(25.8426896372551,0.979354319063382,26.7311577245132));
#43477=CARTESIAN_POINT('Ctrl Pts',(25.8532988401534,0.926207597843734,26.8933297103096));
#43478=CARTESIAN_POINT('Ctrl Pts',(25.8639080430516,0.837442325363041,27.0328387113249));
#43479=CARTESIAN_POINT('Ctrl Pts',(25.8745172459499,0.748677052882357,27.1723477123403));
#43480=CARTESIAN_POINT('Ctrl Pts',(25.8851264488482,0.624293229140633,27.2891937285746));
#43481=CARTESIAN_POINT('Ctrl Pts',(25.8957356517464,0.47951443670336,27.3690757427456));
#43482=CARTESIAN_POINT('Ctrl Pts',(25.9063448546447,0.334735644266086,27.4489577569167));
#43483=CARTESIAN_POINT('Ctrl Pts',(25.916954057543,0.169561883133259,27.4918757690245));
#43484=CARTESIAN_POINT('Ctrl Pts',(25.9275632604413,0.00420909911851084,
27.4925769608318));
#43485=CARTESIAN_POINT('Ctrl Pts',(25.9381724633395,-0.161143684896257,
27.4932781526391));
#43486=CARTESIAN_POINT('Ctrl Pts',(25.9487816662378,-0.326675491792952,
27.4517625241458));
#43487=CARTESIAN_POINT('Ctrl Pts',(25.9593908691361,-0.472126557242158,
27.3731112508604));
#43488=CARTESIAN_POINT('Ctrl Pts',(25.9700000720343,-0.617577622691365,
27.2944599775749));
#43489=CARTESIAN_POINT('Ctrl Pts',(25.9806092749326,-0.742947946693088,
27.1786730594973));
#43490=CARTESIAN_POINT('Ctrl Pts',(25.9912184778309,-0.832893202112376,
27.0399218963483));
#43491=CARTESIAN_POINT('Ctrl Pts',(26.0018276807292,-0.922838457531644,
26.9011707331994));
#43492=CARTESIAN_POINT('Ctrl Pts',(26.0124368836274,-0.977358644368497,
26.7394553249791));
#43493=CARTESIAN_POINT('Ctrl Pts',(26.0230460865257,-0.98978093665147,26.5745683248608));
#43494=CARTESIAN_POINT('Ctrl Pts',(26.0246417984717,-0.991649352250928,
26.5497679549974));
#43495=CARTESIAN_POINT('Ctrl Pts',(26.0262375104178,-0.992565401903803,
26.5248958353196));
#43496=CARTESIAN_POINT('Ctrl Pts',(26.0278332223638,-0.992541444115404,
26.5000219547962));
#43497=CARTESIAN_POINT('Origin',(8.83329938588935,0.,26.5));
#43498=CARTESIAN_POINT('',(26.2332993858894,-0.764743745002543,26.5001497824216));
#43499=CARTESIAN_POINT('',(26.3667006141106,-0.764336903008391,26.49996577981));
#43500=CARTESIAN_POINT('',(8.83329938588935,-0.76435,26.5000000000004));
#43501=CARTESIAN_POINT('',(26.4075,0.702460755335647,26.1986212829383));
#43502=CARTESIAN_POINT('Ctrl Pts',(26.2332993858894,-0.764743745002462,
26.5001497824216));
#43503=CARTESIAN_POINT('Ctrl Pts',(26.2356868595384,-0.764971803409263,
26.4715667170256));
#43504=CARTESIAN_POINT('Ctrl Pts',(26.248659868688,-0.757224410481673,26.3161737266801));
#43505=CARTESIAN_POINT('Ctrl Pts',(26.2722184133381,-0.650892539114633,
26.0420259586536));
#43506=CARTESIAN_POINT('Ctrl Pts',(26.3039750198397,-0.355044020423166,
25.7866217100636));
#43507=CARTESIAN_POINT('Ctrl Pts',(26.3357316263413,0.0308983993041465,
25.7036133259667));
#43508=CARTESIAN_POINT('Ctrl Pts',(26.3674882328429,0.407379290301616,25.8154783693755));
#43509=CARTESIAN_POINT('Ctrl Pts',(26.3914110240625,0.616973295240833,26.0251266306013));
#43510=CARTESIAN_POINT('Ctrl Pts',(26.4047482797815,0.689468221294098,26.1682460674036));
#43511=CARTESIAN_POINT('Ctrl Pts',(26.4075,0.702460755335573,26.1986212829383));
#43512=CARTESIAN_POINT('',(26.4075,-0.612682133358436,26.0429972363723));
#43513=CARTESIAN_POINT('Origin',(26.4075,0.,26.5));
#43514=CARTESIAN_POINT('Ctrl Pts',(26.3667006141105,-0.764336903008216,
26.49996577981));
#43515=CARTESIAN_POINT('Ctrl Pts',(26.3696912065087,-0.76437156972657,26.4640569586302));
#43516=CARTESIAN_POINT('Ctrl Pts',(26.3832910018052,-0.75307130558971,26.3007912409091));
#43517=CARTESIAN_POINT('Ctrl Pts',(26.3968907971017,-0.688841172942706,
26.1451000824837));
#43518=CARTESIAN_POINT('Ctrl Pts',(26.4075,-0.612682133358295,26.0429972363724));
#43519=CARTESIAN_POINT('Origin',(8.83329938588935,0.,26.5));
#43520=CARTESIAN_POINT('',(25.8332993858893,-0.76410090648093,26.4994977389265));
#43521=CARTESIAN_POINT('',(25.9667006141106,-0.764381917188524,26.5000169079586));
#43522=CARTESIAN_POINT('',(8.83329938588935,-0.76435,26.5000000000004));
#43523=CARTESIAN_POINT('Ctrl Pts',(25.8332993858894,-0.764100906480849,
26.4994977389265));
#43524=CARTESIAN_POINT('Ctrl Pts',(25.8419937668654,-0.764022224237484,
26.3951702166934));
#43525=CARTESIAN_POINT('Ctrl Pts',(25.8612736833419,-0.716885713953257,
26.1648471626025));
#43526=CARTESIAN_POINT('Ctrl Pts',(25.8911391353189,-0.489694400926831,
25.8712018432531));
#43527=CARTESIAN_POINT('Ctrl Pts',(25.9228957418205,-0.129772979866902,
25.714079788392));
#43528=CARTESIAN_POINT('Ctrl Pts',(25.9546523483221,0.262368055635802,25.7474805067894));
#43529=CARTESIAN_POINT('Ctrl Pts',(25.9864089548237,0.590141695668152,25.9648661194057));
#43530=CARTESIAN_POINT('Ctrl Pts',(26.0181655613253,0.774521596165084,26.3122796401661));
#43531=CARTESIAN_POINT('Ctrl Pts',(26.0499221678269,0.769515607711255,26.7058087142711));
#43532=CARTESIAN_POINT('Ctrl Pts',(26.0816787743285,0.5780380710276,27.0486892252408));
#43533=CARTESIAN_POINT('Ctrl Pts',(26.1134353808301,0.243724544676253,27.2586608600213));
#43534=CARTESIAN_POINT('Ctrl Pts',(26.1451919873318,-0.146396766368369,
27.282282661157));
#43535=CARTESIAN_POINT('Ctrl Pts',(26.1851466556847,-0.600082663475827,
27.0752341583171));
#43536=CARTESIAN_POINT('Ctrl Pts',(26.2145157885374,-0.762949481309626,
26.7250288263006));
#43537=CARTESIAN_POINT('Ctrl Pts',(26.2332993858894,-0.764743745002462,
26.5001497824216));
#43538=CARTESIAN_POINT('Ctrl Pts',(25.9667006141105,-0.764381917188349,
26.5000169079586));
#43539=CARTESIAN_POINT('Ctrl Pts',(25.9757141050628,-0.764277698162404,
26.3918127800182));
#43540=CARTESIAN_POINT('Ctrl Pts',(25.9953367989134,-0.713766127520463,
26.1561543088668));
#43541=CARTESIAN_POINT('Ctrl Pts',(26.0255686956621,-0.479811640722421,
25.8637012684045));
#43542=CARTESIAN_POINT('Ctrl Pts',(26.057396304357,-0.116058362262509,25.7115674057289));
#43543=CARTESIAN_POINT('Ctrl Pts',(26.0892239130518,0.276104304993651,25.7524295460381));
#43544=CARTESIAN_POINT('Ctrl Pts',(26.1210515217466,0.600680758111244,25.9762843069252));
#43545=CARTESIAN_POINT('Ctrl Pts',(26.1528791304414,0.778220766932473,26.3283374916096));
#43546=CARTESIAN_POINT('Ctrl Pts',(26.1847067391362,0.765263715417021,26.7224086099901));
#43547=CARTESIAN_POINT('Ctrl Pts',(26.216534347831,0.564984430859093,27.0620420026143));
#43548=CARTESIAN_POINT('Ctrl Pts',(26.2483619565259,0.226402125810272,27.2640883311776));
#43549=CARTESIAN_POINT('Ctrl Pts',(26.2801895652207,-0.167592445455861,
27.2791135571752));
#43550=CARTESIAN_POINT('Ctrl Pts',(26.3120171739155,-0.520576980781025,
27.1033949839955));
#43551=CARTESIAN_POINT('Ctrl Pts',(26.3408541902121,-0.724914826684035,
26.8104148753484));
#43552=CARTESIAN_POINT('Ctrl Pts',(26.3590820036105,-0.764248588657984,
26.591444418708));
#43553=CARTESIAN_POINT('Ctrl Pts',(26.3667006141105,-0.764336903008216,
26.49996577981));
#43554=CARTESIAN_POINT('Origin',(8.83329938588935,0.,26.5));
#43555=CARTESIAN_POINT('',(25.4332993858893,-0.764263253905602,26.5001078466209));
#43556=CARTESIAN_POINT('',(25.5667006141106,-0.76429105465224,26.4999904661865));
#43557=CARTESIAN_POINT('',(8.83329938588935,-0.76435,26.5000000000004));
#43558=CARTESIAN_POINT('Ctrl Pts',(25.4332993858894,-0.764263253905522,
26.5001078466209));
#43559=CARTESIAN_POINT('Ctrl Pts',(25.4377151386918,-0.764307689690715,
26.4469830257742));
#43560=CARTESIAN_POINT('Ctrl Pts',(25.4527164269947,-0.745911257864019,
26.2664836537655));
#43561=CARTESIAN_POINT('Ctrl Pts',(25.4783032507982,-0.605796091498349,
25.9827740341064));
#43562=CARTESIAN_POINT('Ctrl Pts',(25.5100598572998,-0.284456618484401,
25.7555491887942));
#43563=CARTESIAN_POINT('Ctrl Pts',(25.5418164638014,0.106261602193242,25.710478634078));
#43564=CARTESIAN_POINT('Ctrl Pts',(25.5735730703029,0.471160163992154,25.857247576466));
#43565=CARTESIAN_POINT('Ctrl Pts',(25.6053296768046,0.720988905220201,26.1613458949732));
#43566=CARTESIAN_POINT('Ctrl Pts',(25.6370862833062,0.795604641852137,26.5469146534013));
#43567=CARTESIAN_POINT('Ctrl Pts',(25.6688428898078,0.675347181544284,26.9229352697116));
#43568=CARTESIAN_POINT('Ctrl Pts',(25.7005994963094,0.392306217773594,27.1924551729066));
#43569=CARTESIAN_POINT('Ctrl Pts',(25.7429416383115,-0.116715244884512,
27.3346019054481));
#43570=CARTESIAN_POINT('Ctrl Pts',(25.7852837803136,-0.621351287349472,
27.0693025272348));
#43571=CARTESIAN_POINT('Ctrl Pts',(25.8189315413398,-0.757620506138495,
26.6720477734371));
#43572=CARTESIAN_POINT('Ctrl Pts',(25.8314082313648,-0.764118021015047,
26.5221904948858));
#43573=CARTESIAN_POINT('Ctrl Pts',(25.8332993858894,-0.764100906480849,
26.4994977389265));
#43574=CARTESIAN_POINT('Ctrl Pts',(25.5667006141106,-0.764291054652064,
26.4999904661865));
#43575=CARTESIAN_POINT('Ctrl Pts',(25.5711278007186,-0.764314295420762,
26.4468253249029));
#43576=CARTESIAN_POINT('Ctrl Pts',(25.5861641902249,-0.745745270709442,
26.2662725291791));
#43577=CARTESIAN_POINT('Ctrl Pts',(25.6118097826295,-0.605100924877577,
25.9813978095313));
#43578=CARTESIAN_POINT('Ctrl Pts',(25.6436373913244,-0.282434449814925,
25.7547979181797));
#43579=CARTESIAN_POINT('Ctrl Pts',(25.6754650000191,0.109367451560953,25.710611552006));
#43580=CARTESIAN_POINT('Ctrl Pts',(25.707292608714,0.474397953853924,25.8596548254688));
#43581=CARTESIAN_POINT('Ctrl Pts',(25.7391202174087,0.723303440713549,26.1654443336632));
#43582=CARTESIAN_POINT('Ctrl Pts',(25.7709478261036,0.795155838932149,26.553127707192));
#43583=CARTESIAN_POINT('Ctrl Pts',(25.8027754347984,0.672366832289694,26.9278062684317));
#43584=CARTESIAN_POINT('Ctrl Pts',(25.8346030434933,0.384993203039443,27.1977647143017));
#43585=CARTESIAN_POINT('Ctrl Pts',(25.8664306521881,0.00337940660061129,
27.2969215381445));
#43586=CARTESIAN_POINT('Ctrl Pts',(25.8982582608829,-0.379061610834525,
27.2010047503193));
#43587=CARTESIAN_POINT('Ctrl Pts',(25.9300858695777,-0.668714428418505,
26.9334932213543));
#43588=CARTESIAN_POINT('Ctrl Pts',(25.9528999873202,-0.759004503313977,
26.6656787260802));
#43589=CARTESIAN_POINT('Ctrl Pts',(25.9651049021645,-0.764400367702759,
26.5191729286921));
#43590=CARTESIAN_POINT('Ctrl Pts',(25.9667006141105,-0.764381917188349,
26.5000169079586));
#43591=CARTESIAN_POINT('Origin',(8.83329938588935,0.,26.5));
#43592=CARTESIAN_POINT('',(25.0332993858893,-0.764359839502163,26.5000448214614));
#43593=CARTESIAN_POINT('',(25.1667006141106,-0.764415689723997,26.5000020449434));
#43594=CARTESIAN_POINT('',(8.83329938588935,-0.76435,26.5000000000004));
#43595=CARTESIAN_POINT('Ctrl Pts',(25.0332993858894,-0.764359839502083,
26.5000448214614));
#43596=CARTESIAN_POINT('Ctrl Pts',(25.0334365105182,-0.764359396665192,
26.4983993445537));
#43597=CARTESIAN_POINT('Ctrl Pts',(25.0441591706476,-0.763902763666039,
26.3697273014672));
#43598=CARTESIAN_POINT('Ctrl Pts',(25.0654673662775,-0.697329274606203,
26.1141833843906));
#43599=CARTESIAN_POINT('Ctrl Pts',(25.097223972779,-0.427657617209193,25.827880607489));
#43600=CARTESIAN_POINT('Ctrl Pts',(25.1289805792807,-0.0540728476927859,
25.7048907589234));
#43601=CARTESIAN_POINT('Ctrl Pts',(25.1607371857822,0.33294494419036,25.7763569468244));
#43602=CARTESIAN_POINT('Ctrl Pts',(25.1924937922838,0.638517242951082,26.0230477368148));
#43603=CARTESIAN_POINT('Ctrl Pts',(25.2242503987854,0.788945293266577,26.3880474112795));
#43604=CARTESIAN_POINT('Ctrl Pts',(25.256007005287,0.746270734187485,26.7765471503739));
#43605=CARTESIAN_POINT('Ctrl Pts',(25.2983491472892,0.44872275221358,27.2133236857863));
#43606=CARTESIAN_POINT('Ctrl Pts',(25.3406912892913,-0.108098811743075,
27.335761590382));
#43607=CARTESIAN_POINT('Ctrl Pts',(25.3830334312934,-0.561424858091366,
27.0640926021514));
#43608=CARTESIAN_POINT('Ctrl Pts',(25.4103742849926,-0.735087659068443,
26.7758787289326));
#43609=CARTESIAN_POINT('Ctrl Pts',(25.4271296031913,-0.764201167291771,
26.5743349637552));
#43610=CARTESIAN_POINT('Ctrl Pts',(25.4332993858894,-0.764263253905522,
26.5001078466209));
#43611=CARTESIAN_POINT('Ctrl Pts',(25.1667006141106,-0.764415689723821,
26.5000020449434));
#43612=CARTESIAN_POINT('Ctrl Pts',(25.1771506992727,-0.764396471048405,
26.3745681243369));
#43613=CARTESIAN_POINT('Ctrl Pts',(25.1982099873331,-0.700903229582064,
26.1217716260069));
#43614=CARTESIAN_POINT('Ctrl Pts',(25.2298784782917,-0.435669391136255,
25.832701309116));
#43615=CARTESIAN_POINT('Ctrl Pts',(25.2617060869866,-0.0624580063800852,
25.705522587692));
#43616=CARTESIAN_POINT('Ctrl Pts',(25.2935336956813,0.326042097238796,25.7728192026347));
#43617=CARTESIAN_POINT('Ctrl Pts',(25.3253613043762,0.634732321372251,26.0181180212604));
#43618=CARTESIAN_POINT('Ctrl Pts',(25.357188913071,0.78805024694888,26.3813738245058));
#43619=CARTESIAN_POINT('Ctrl Pts',(25.3890165217658,0.748466103221927,26.7736674141299));
#43620=CARTESIAN_POINT('Ctrl Pts',(25.4208441304606,0.525669454106653,27.0989716072131));
#43621=CARTESIAN_POINT('Ctrl Pts',(25.4526717391554,0.174197348243338,27.2776571513812));
#43622=CARTESIAN_POINT('Ctrl Pts',(25.4844993478503,-0.219915476373876,
27.2659846894545));
#43623=CARTESIAN_POINT('Ctrl Pts',(25.5163269565451,-0.560196517256405,
27.0668114530277));
#43624=CARTESIAN_POINT('Ctrl Pts',(25.5437273786318,-0.735091936016483,
26.7758961151728));
#43625=CARTESIAN_POINT('Ctrl Pts',(25.5605185978203,-0.764258601804826,
26.5742289834629));
#43626=CARTESIAN_POINT('Ctrl Pts',(25.5667006141106,-0.764291054652064,
26.4999904661865));
#43627=CARTESIAN_POINT('Origin',(8.83329938588935,0.,26.5));
#43628=CARTESIAN_POINT('',(24.6332993858894,-0.76435,26.5000000000003));
#43629=CARTESIAN_POINT('',(24.7667006141106,-0.764286798414632,26.5000062214473));
#43630=CARTESIAN_POINT('',(8.83329938588935,-0.76435,26.5000000000004));
#43631=CARTESIAN_POINT('Ctrl Pts',(24.6332993858894,-0.764326480586209,
26.5000191213087));
#43632=CARTESIAN_POINT('Ctrl Pts',(24.6397434178451,-0.764258932917326,
26.4226419695689));
#43633=CARTESIAN_POINT('Ctrl Pts',(24.6567729853014,-0.733280117843162,
26.2181201080417));
#43634=CARTESIAN_POINT('Ctrl Pts',(24.6843880882583,-0.553842691960536,
25.9269547568778));
#43635=CARTESIAN_POINT('Ctrl Pts',(24.7161446947598,-0.211884413187848,
25.7321350380964));
#43636=CARTESIAN_POINT('Ctrl Pts',(24.7479013012615,0.180748963367304,25.7237799647362));
#43637=CARTESIAN_POINT('Ctrl Pts',(24.7796579077631,0.531025222621527,25.90587857232));
#43638=CARTESIAN_POINT('Ctrl Pts',(24.8114145142647,0.74881272581408,26.2304117273629));
#43639=CARTESIAN_POINT('Ctrl Pts',(24.8537566562668,0.802855019359397,26.7561378670706));
#43640=CARTESIAN_POINT('Ctrl Pts',(24.8960987982689,0.456057920405105,27.2086564487069));
#43641=CARTESIAN_POINT('Ctrl Pts',(24.9384409402711,-0.0656403540824771,
27.2931517376899));
#43642=CARTESIAN_POINT('Ctrl Pts',(24.9701975467727,-0.435634749553036,
27.1672259159165));
#43643=CARTESIAN_POINT('Ctrl Pts',(25.0018170286454,-0.701384614530829,
26.8775928202282));
#43644=CARTESIAN_POINT('Ctrl Pts',(25.0228509750177,-0.764393582104101,
26.6254243317562));
#43645=CARTESIAN_POINT('Ctrl Pts',(25.0332993858894,-0.764359839502083,
26.5000448214614));
#43646=CARTESIAN_POINT('Ctrl Pts',(24.7667006141106,-0.764286798414457,
26.5000062214473));
#43647=CARTESIAN_POINT('Ctrl Pts',(24.7725643949285,-0.764266847137901,
26.4295882043572));
#43648=CARTESIAN_POINT('Ctrl Pts',(24.7890373786446,-0.737166213800641,
26.2317494504216));
#43649=CARTESIAN_POINT('Ctrl Pts',(24.8161195652591,-0.568633391362849,
25.9416529507056));
#43650=CARTESIAN_POINT('Ctrl Pts',(24.8479471739539,-0.231377401638892,
25.7373992792821));
#43651=CARTESIAN_POINT('Ctrl Pts',(24.8797747826487,0.16251606740706,25.7198180410551));
#43652=CARTESIAN_POINT('Ctrl Pts',(24.9116023913435,0.516628208017037,25.8932128413441));
#43653=CARTESIAN_POINT('Ctrl Pts',(24.9434300000383,0.744278044004932,26.2151394122719));
#43654=CARTESIAN_POINT('Ctrl Pts',(24.9752576087332,0.78974054437337,26.6067952892288));
#43655=CARTESIAN_POINT('Ctrl Pts',(25.007085217428,0.641887217721265,26.9723093911354));
#43656=CARTESIAN_POINT('Ctrl Pts',(25.0389128261228,0.336910188567394,27.2222097244347));
#43657=CARTESIAN_POINT('Ctrl Pts',(25.0707404348176,-0.0505370546315667,
27.2953246930265));
#43658=CARTESIAN_POINT('Ctrl Pts',(25.1025680435124,-0.425613636882587,
27.1737569245123));
#43659=CARTESIAN_POINT('Ctrl Pts',(25.1343956522073,-0.696506822711343,
26.8872642600927));
#43660=CARTESIAN_POINT('Ctrl Pts',(25.15577317574,-0.763941742375046,26.6311655609095));
#43661=CARTESIAN_POINT('Ctrl Pts',(25.1665414963744,-0.764415982356089,
26.5019119587072));
#43662=CARTESIAN_POINT('Ctrl Pts',(25.1667006141106,-0.764415689723821,
26.5000020449434));
#43663=CARTESIAN_POINT('Origin',(8.83329938588935,0.,26.5));
#43664=CARTESIAN_POINT('',(24.2332993858894,-0.76435,26.5000000000003));
#43665=CARTESIAN_POINT('',(24.3667006141106,-0.764392673201869,26.4999855108973));
#43666=CARTESIAN_POINT('',(8.83329938588935,-0.76435,26.5000000000004));
#43667=CARTESIAN_POINT('Ctrl Pts',(24.2332993858894,-0.76435,26.5000000000003));
#43668=CARTESIAN_POINT('Ctrl Pts',(24.2511698941678,-0.764350000000088,
26.28543985601));
#43669=CARTESIAN_POINT('Ctrl Pts',(24.2690404024462,-0.669038051787615,
26.0726183635796));
#43670=CARTESIAN_POINT('Ctrl Pts',(24.2869109107247,-0.508962945483454,
25.9297477377293));
#43671=CARTESIAN_POINT('Ctrl Pts',(24.3047814190031,-0.348887839179292,
25.7868771118791));
#43672=CARTESIAN_POINT('Ctrl Pts',(24.3226519272816,-0.126643857468994,
25.716272808144));
#43673=CARTESIAN_POINT('Ctrl Pts',(24.34052243556,0.0865367472360207,25.7405644768133));
#43674=CARTESIAN_POINT('Ctrl Pts',(24.3583929438384,0.299717351941035,25.7648561454827));
#43675=CARTESIAN_POINT('Ctrl Pts',(24.3762634521169,0.500379634243882,25.8836500997622));
#43676=CARTESIAN_POINT('Ctrl Pts',(24.3941339603953,0.624208573182235,26.0588712436648));
#43677=CARTESIAN_POINT('Ctrl Pts',(24.4120044686738,0.748037512120589,26.2340923875675));
#43678=CARTESIAN_POINT('Ctrl Pts',(24.4298749769522,0.793026254288728,26.4629009717388));
#43679=CARTESIAN_POINT('Ctrl Pts',(24.4477454852306,0.744755289141838,26.671960698403));
#43680=CARTESIAN_POINT('Ctrl Pts',(24.4656159935091,0.696484323994948,26.8810204250673));
#43681=CARTESIAN_POINT('Ctrl Pts',(24.4834865017875,0.555735962611789,27.0669431344933));
#43682=CARTESIAN_POINT('Ctrl Pts',(24.501357010066,0.367621990370684,27.1701380415227));
#43683=CARTESIAN_POINT('Ctrl Pts',(24.5192275183444,0.179508018129579,27.2733329485521));
#43684=CARTESIAN_POINT('Ctrl Pts',(24.5370980266228,-0.0529228659408549,
27.2921276085011));
#43685=CARTESIAN_POINT('Ctrl Pts',(24.5549685349013,-0.255173367133682,
27.2204980743941));
#43686=CARTESIAN_POINT('Ctrl Pts',(24.5728390431797,-0.457423868326509,
27.1488685402871));
#43687=CARTESIAN_POINT('Ctrl Pts',(24.5907095514582,-0.626216181706892,
26.9879756875681));
#43688=CARTESIAN_POINT('Ctrl Pts',(24.6085800597366,-0.707450049624245,
26.7893878881133));
#43689=CARTESIAN_POINT('Ctrl Pts',(24.6168198351208,-0.744905549759095,
26.6978225651764));
#43690=CARTESIAN_POINT('Ctrl Pts',(24.6250596105051,-0.76434999999996,26.5989298885825));
#43691=CARTESIAN_POINT('Ctrl Pts',(24.6332993858894,-0.76435,26.5000000000003));
#43692=CARTESIAN_POINT('Ctrl Pts',(24.3667006141106,-0.764392673201694,
26.4999855108973));
#43693=CARTESIAN_POINT('Ctrl Pts',(24.3679780905843,-0.764405945073535,
26.4846504315273));
#43694=CARTESIAN_POINT('Ctrl Pts',(24.3798647699562,-0.760200367936652,
26.3419676628929));
#43695=CARTESIAN_POINT('Ctrl Pts',(24.4023606522264,-0.675139866205197,
26.076583512025));
#43696=CARTESIAN_POINT('Ctrl Pts',(24.4341882609213,-0.389531207732191,
25.8047584596478));
#43697=CARTESIAN_POINT('Ctrl Pts',(24.4660158696161,-0.00857155315095306,
25.7031173927703));
#43698=CARTESIAN_POINT('Ctrl Pts',(24.4978434783109,0.37448628025374,25.7965404154251));
#43699=CARTESIAN_POINT('Ctrl Pts',(24.5296710870057,0.66587587465148,26.0621590690836));
#43700=CARTESIAN_POINT('Ctrl Pts',(24.5614986957005,0.79426972782966,26.4349541647604));
#43701=CARTESIAN_POINT('Ctrl Pts',(24.5933263043954,0.728239082472559,26.8236714383262));
#43702=CARTESIAN_POINT('Ctrl Pts',(24.6251539130902,0.483947182200952,27.1331591317105));
#43703=CARTESIAN_POINT('Ctrl Pts',(24.656981521785,0.121192768603945,27.2876596181516));
#43704=CARTESIAN_POINT('Ctrl Pts',(24.6888091304798,-0.271227692226556,
27.2493536549575));
#43705=CARTESIAN_POINT('Ctrl Pts',(24.7206367391747,-0.597255961333821,
27.0276179279363));
#43706=CARTESIAN_POINT('Ctrl Pts',(24.7466005670515,-0.743954520432521,
26.7413759004361));
#43707=CARTESIAN_POINT('Ctrl Pts',(24.7619551920302,-0.76430294452074,26.5569938926328));
#43708=CARTESIAN_POINT('Ctrl Pts',(24.7667006141106,-0.764286798414457,
26.5000062214473));
#43709=CARTESIAN_POINT('Origin',(8.83329938588935,0.,26.5));
#43710=CARTESIAN_POINT('',(23.8332993858894,-0.764350202263794,26.5000021273756));
#43711=CARTESIAN_POINT('',(23.9667006141106,-0.764318926635532,26.5000181819409));
#43712=CARTESIAN_POINT('',(8.83329938588935,-0.76435,26.5000000000004));
#43713=CARTESIAN_POINT('Ctrl Pts',(23.8332993858894,-0.764350202263713,
26.5000021273756));
#43714=CARTESIAN_POINT('Ctrl Pts',(23.8417716969985,-0.764313879349882,
26.3983501280956));
#43715=CARTESIAN_POINT('Ctrl Pts',(23.8608295436081,-0.718603697792442,
26.1696958781128));
#43716=CARTESIAN_POINT('Ctrl Pts',(23.8904729257184,-0.495790608642908,
25.8761733171223));
#43717=CARTESIAN_POINT('Ctrl Pts',(23.9222295322199,-0.139108740631515,
25.7163884295363));
#43718=CARTESIAN_POINT('Ctrl Pts',(23.9645716742221,0.388186146399965,25.752006480776));
#43719=CARTESIAN_POINT('Ctrl Pts',(24.0069138162242,0.775559022505738,26.170316831385));
#43720=CARTESIAN_POINT('Ctrl Pts',(24.0492559582264,0.770636562786746,26.6987904001223));
#43721=CARTESIAN_POINT('Ctrl Pts',(24.0810125647279,0.583970020170633,27.0421688606243));
#43722=CARTESIAN_POINT('Ctrl Pts',(24.1127691712296,0.252144193813407,27.2560496256394));
#43723=CARTESIAN_POINT('Ctrl Pts',(24.1445257777311,-0.139564942859222,
27.2842405440908));
#43724=CARTESIAN_POINT('Ctrl Pts',(24.1762823842328,-0.498157324775064,
27.1220625835686));
#43725=CARTESIAN_POINT('Ctrl Pts',(24.2058735869521,-0.718613983320539,
26.8292929532382));
#43726=CARTESIAN_POINT('Ctrl Pts',(24.224879254171,-0.764289435210411,26.6010635220894));
#43727=CARTESIAN_POINT('Ctrl Pts',(24.2332993858894,-0.764406944917652,
26.4999838305765));
#43728=CARTESIAN_POINT('Ctrl Pts',(23.9667006141106,-0.764318926635357,
26.5000181819409));
#43729=CARTESIAN_POINT('Ctrl Pts',(23.9740009891383,-0.764242150819898,
26.4123586904196));
#43730=CARTESIAN_POINT('Ctrl Pts',(23.9919105670644,-0.727291940328121,
26.1972457893952));
#43731=CARTESIAN_POINT('Ctrl Pts',(24.0204293478886,-0.529560802386153,
25.9044660229636));
#43732=CARTESIAN_POINT('Ctrl Pts',(24.0522569565835,-0.179260354208531,
25.7234943099773));
#43733=CARTESIAN_POINT('Ctrl Pts',(24.0840845652783,0.214920155430682,25.7325987437994));
#43734=CARTESIAN_POINT('Ctrl Pts',(24.1159121739731,0.556491655837079,25.9295507049594));
#43735=CARTESIAN_POINT('Ctrl Pts',(24.1477397826679,0.761842918540557,26.2661395101813));
#43736=CARTESIAN_POINT('Ctrl Pts',(24.1795673913627,0.780707245874303,26.6599736149119));
#43737=CARTESIAN_POINT('Ctrl Pts',(24.2113950000576,0.608466952871163,27.0146487428259));
#43738=CARTESIAN_POINT('Ctrl Pts',(24.2432226087524,0.287283702529686,27.2433461074691));
#43739=CARTESIAN_POINT('Ctrl Pts',(24.2750502174472,-0.104221993505796,
27.2900842596193));
#43740=CARTESIAN_POINT('Ctrl Pts',(24.306877826142,-0.470215816038203,27.1434224487661));
#43741=CARTESIAN_POINT('Ctrl Pts',(24.3374279583631,-0.711038177639814,
26.8514693703178));
#43742=CARTESIAN_POINT('Ctrl Pts',(24.357368887686,-0.76429572466314,26.6120053941018));
#43743=CARTESIAN_POINT('Ctrl Pts',(24.3667006141106,-0.764392673201694,
26.4999855108973));
#43744=CARTESIAN_POINT('Origin',(8.83329938588935,0.,26.5));
#43745=CARTESIAN_POINT('',(23.4332993858894,-0.764263770835984,26.4997503415534));
#43746=CARTESIAN_POINT('',(23.5667006141106,-0.764339792548135,26.4999799994015));
#43747=CARTESIAN_POINT('',(8.83329938588935,-0.76435,26.5000000000004));
#43748=CARTESIAN_POINT('Ctrl Pts',(23.4332993858894,-0.764263770835903,
26.4997503415534));
#43749=CARTESIAN_POINT('Ctrl Pts',(23.4374930688249,-0.764282468728799,
26.4493207649479));
#43750=CARTESIAN_POINT('Ctrl Pts',(23.452272287261,-0.746995563910679,26.2717621776462));
#43751=CARTESIAN_POINT('Ctrl Pts',(23.4776370411976,-0.611445654087914,
25.9905566300544));
#43752=CARTESIAN_POINT('Ctrl Pts',(23.5199791831997,-0.185345401108989,
25.6779112752593));
#43753=CARTESIAN_POINT('Ctrl Pts',(23.5623213252019,0.380448766828713,25.7480415404581));
#43754=CARTESIAN_POINT('Ctrl Pts',(23.604663467204,0.717322101045798,26.1552575766811));
#43755=CARTESIAN_POINT('Ctrl Pts',(23.6364200737056,0.795937182645239,26.538105894183));
#43756=CARTESIAN_POINT('Ctrl Pts',(23.6681766802072,0.680101105708285,26.915511993711));
#43757=CARTESIAN_POINT('Ctrl Pts',(23.6999332867088,0.398791784083484,27.1895481978939));
#43758=CARTESIAN_POINT('Ctrl Pts',(23.7316898932104,0.0200962396143968,
27.296692361741));
#43759=CARTESIAN_POINT('Ctrl Pts',(23.763446499712,-0.363306363014758,27.2089739077987));
#43760=CARTESIAN_POINT('Ctrl Pts',(23.7952031062136,-0.658432051321634,
26.9489875409133));
#43761=CARTESIAN_POINT('Ctrl Pts',(23.8184874016061,-0.756830249032618,
26.6777191819525));
#43762=CARTESIAN_POINT('Ctrl Pts',(23.831186161498,-0.764359262184493,26.5253568955782));
#43763=CARTESIAN_POINT('Ctrl Pts',(23.8332993858894,-0.764350202263713,
26.5000021273756));
#43764=CARTESIAN_POINT('Ctrl Pts',(23.5667006141106,-0.76433979254796,26.4999799994015));
#43765=CARTESIAN_POINT('Ctrl Pts',(23.5694146847941,-0.764372599419905,
26.4673932611465));
#43766=CARTESIAN_POINT('Ctrl Pts',(23.5827379583759,-0.754334726260367,
26.3074462255872));
#43767=CARTESIAN_POINT('Ctrl Pts',(23.6066704348561,-0.644950851448086,
26.0318827492551));
#43768=CARTESIAN_POINT('Ctrl Pts',(23.6384980435508,-0.341608481918587,
25.7800006900629));
#43769=CARTESIAN_POINT('Ctrl Pts',(23.6703256522457,0.0453541685624505,
25.7043629215386));
#43770=CARTESIAN_POINT('Ctrl Pts',(23.7021532609405,0.421214845532138,25.8234843570678));
#43771=CARTESIAN_POINT('Ctrl Pts',(23.7339808696353,0.693968879696766,26.1082059785538));
#43772=CARTESIAN_POINT('Ctrl Pts',(23.7658084783301,0.796850455291405,26.4888324966759));
#43773=CARTESIAN_POINT('Ctrl Pts',(23.797636087025,0.704675811632944,26.8721926406151));
#43774=CARTESIAN_POINT('Ctrl Pts',(23.8294636957197,0.440007824081036,27.1644459917676));
#43775=CARTESIAN_POINT('Ctrl Pts',(23.8612913044146,0.0676329737958395,
27.2940536141119));
#43776=CARTESIAN_POINT('Ctrl Pts',(23.8931189131094,-0.321297344429241,
27.229289639095));
#43777=CARTESIAN_POINT('Ctrl Pts',(23.9249465218042,-0.631579222606048,
26.9860072497412));
#43778=CARTESIAN_POINT('Ctrl Pts',(23.9494737554713,-0.751551611982924,
26.7068480384306));
#43779=CARTESIAN_POINT('Ctrl Pts',(23.9633917862401,-0.76435372456793,26.5397490406375));
#43780=CARTESIAN_POINT('Ctrl Pts',(23.9667006141106,-0.764318926635357,
26.5000181819409));
#43781=CARTESIAN_POINT('Origin',(8.83329938588935,0.,26.5));
#43782=CARTESIAN_POINT('',(23.0332993858893,-0.764131106302846,26.5004425504153));
#43783=CARTESIAN_POINT('',(23.1667006141106,-0.76437181183062,26.5000184759214));
#43784=CARTESIAN_POINT('',(8.83329938588935,-0.76435,26.5000000000004));
#43785=CARTESIAN_POINT('Ctrl Pts',(23.0332993858894,-0.764131106302765,
26.5004425504153));
#43786=CARTESIAN_POINT('Ctrl Pts',(23.0437999761519,-0.764286156156834,
26.374143586));
#43787=CARTESIAN_POINT('Ctrl Pts',(23.0754716374155,-0.670638391197475,
25.9903175893888));
#43788=CARTESIAN_POINT('Ctrl Pts',(23.1177288341795,-0.193816666742857,
25.679867151767));
#43789=CARTESIAN_POINT('Ctrl Pts',(23.1600709761817,0.326217167037633,25.7740656400097));
#43790=CARTESIAN_POINT('Ctrl Pts',(23.1918275826833,0.633093647904743,26.0160986765141));
#43791=CARTESIAN_POINT('Ctrl Pts',(23.2235841891849,0.787795093385811,26.3793077395167));
#43792=CARTESIAN_POINT('Ctrl Pts',(23.2553407956864,0.749355516936845,26.7701442457419));
#43793=CARTESIAN_POINT('Ctrl Pts',(23.2870974021881,0.528886386857991,27.0961558251828));
#43794=CARTESIAN_POINT('Ctrl Pts',(23.3188540086896,0.179216412751493,27.2762196807263));
#43795=CARTESIAN_POINT('Ctrl Pts',(23.3506106151912,-0.213999927519153,
27.2676761095181));
#43796=CARTESIAN_POINT('Ctrl Pts',(23.3823672216928,-0.55507609312846,27.071316142874));
#43797=CARTESIAN_POINT('Ctrl Pts',(23.4099301452589,-0.733777314969458,
26.7810545816172));
#43798=CARTESIAN_POINT('Ctrl Pts',(23.4269075333244,-0.764235272216312,
26.5766131906364));
#43799=CARTESIAN_POINT('Ctrl Pts',(23.4332993858894,-0.764263770835903,
26.4997503415534));
#43800=CARTESIAN_POINT('Ctrl Pts',(23.1667006141106,-0.764371811830445,
26.5000184759214));
#43801=CARTESIAN_POINT('Ctrl Pts',(23.1754375833482,-0.764265346458016,
26.395129905246));
#43802=CARTESIAN_POINT('Ctrl Pts',(23.1947837554841,-0.716081099388898,
26.1627815520115));
#43803=CARTESIAN_POINT('Ctrl Pts',(23.2247391305182,-0.488062159497627,
25.8700073891742));
#43804=CARTESIAN_POINT('Ctrl Pts',(23.2565667392131,-0.126322069100469,
25.7131467124763));
#43805=CARTESIAN_POINT('Ctrl Pts',(23.2883943479078,0.266339639077475,25.7488951086002));
#43806=CARTESIAN_POINT('Ctrl Pts',(23.3202219566027,0.593805672595626,25.9685019431627));
#43807=CARTESIAN_POINT('Ctrl Pts',(23.3520495652975,0.775917595190683,26.3182109829992));
#43808=CARTESIAN_POINT('Ctrl Pts',(23.3838771739923,0.768097327165974,26.7124190604186));
#43809=CARTESIAN_POINT('Ctrl Pts',(23.4157047826871,0.572259144787906,27.0546303565756));
#43810=CARTESIAN_POINT('Ctrl Pts',(23.4475323913819,0.236341096138676,27.2610770312554));
#43811=CARTESIAN_POINT('Ctrl Pts',(23.4793600000768,-0.157429464686238,
27.281224247497));
#43812=CARTESIAN_POINT('Ctrl Pts',(23.5111876087716,-0.512663815891357,
27.1101402896911));
#43813=CARTESIAN_POINT('Ctrl Pts',(23.5403011467829,-0.722815200106324,
26.8170287044339));
#43814=CARTESIAN_POINT('Ctrl Pts',(23.5588054818958,-0.764244358559034,
26.5947736274853));
#43815=CARTESIAN_POINT('Ctrl Pts',(23.5667006141106,-0.76433979254796,26.4999799994015));
#43816=CARTESIAN_POINT('Origin',(8.83329938588935,0.,26.5));
#43817=CARTESIAN_POINT('',(22.6332993858894,-0.764122705815582,26.5000528068419));
#43818=CARTESIAN_POINT('',(22.7667006141106,-0.764296184799811,26.4999878263918));
#43819=CARTESIAN_POINT('',(8.83329938588935,-0.76435,26.5000000000004));
#43820=CARTESIAN_POINT('Ctrl Pts',(22.6332993858894,-0.764122705815501,
26.5000528068419));
#43821=CARTESIAN_POINT('Ctrl Pts',(22.6501068834788,-0.762277025578763,
26.2987504101115));
#43822=CARTESIAN_POINT('Ctrl Pts',(22.6774999165688,-0.629581927431558,
25.9707755262326));
#43823=CARTESIAN_POINT('Ctrl Pts',(22.7154784851593,-0.218505020300182,
25.7347197303026));
#43824=CARTESIAN_POINT('Ctrl Pts',(22.7472350916609,0.172123229852927,25.7219629497037));
#43825=CARTESIAN_POINT('Ctrl Pts',(22.7789916981625,0.524512533349801,25.899938058812));
#43826=CARTESIAN_POINT('Ctrl Pts',(22.8107483046641,0.747044085909005,26.2235280520929));
#43827=CARTESIAN_POINT('Ctrl Pts',(22.8425049111657,0.788621357728243,26.6148866059988));
#43828=CARTESIAN_POINT('Ctrl Pts',(22.8742615176673,0.637345306587861,26.9779398241586));
#43829=CARTESIAN_POINT('Ctrl Pts',(22.9060181241689,0.331205804787041,27.2248622579349));
#43830=CARTESIAN_POINT('Ctrl Pts',(22.9377747306705,-0.0561303630539786,
27.2945822717721));
#43831=CARTESIAN_POINT('Ctrl Pts',(22.9695313371721,-0.429102675280415,
27.1716089821991));
#43832=CARTESIAN_POINT('Ctrl Pts',(23.0012879436737,-0.698667848123337,
26.8831857198376));
#43833=CARTESIAN_POINT('Ctrl Pts',(23.0225439599128,-0.763715786563097,
26.6297987621571));
#43834=CARTESIAN_POINT('Ctrl Pts',(23.0332144406513,-0.764129852016441,
26.501464254465));
#43835=CARTESIAN_POINT('Ctrl Pts',(23.0332993858894,-0.764131106302765,
26.5004425504153));
#43836=CARTESIAN_POINT('Ctrl Pts',(22.7667006141106,-0.764296184799636,
26.4999878263918));
#43837=CARTESIAN_POINT('Ctrl Pts',(22.770851279004,-0.764324242497102,26.450144332975));
#43838=CARTESIAN_POINT('Ctrl Pts',(22.7856111467957,-0.747251188337183,
26.2729185987678));
#43839=CARTESIAN_POINT('Ctrl Pts',(22.8109802174856,-0.611807151357293,
25.9893265517215));
#43840=CARTESIAN_POINT('Ctrl Pts',(22.8428078261804,-0.292120759998493,
25.7585414220562));
#43841=CARTESIAN_POINT('Ctrl Pts',(22.8746354348752,0.0990721111926007,
25.7092534679099));
#43842=CARTESIAN_POINT('Ctrl Pts',(22.9064630435701,0.466013717526745,25.853527590453));
#43843=CARTESIAN_POINT('Ctrl Pts',(22.9382906522649,0.718882635243795,26.1560477969637));
#43844=CARTESIAN_POINT('Ctrl Pts',(22.9701182609597,0.795780606359475,26.5427619897895));
#43845=CARTESIAN_POINT('Ctrl Pts',(23.0019458696545,0.677884240092678,26.9190087329192));
#43846=CARTESIAN_POINT('Ctrl Pts',(23.0337734783493,0.394052677220659,27.1926888542512));
#43847=CARTESIAN_POINT('Ctrl Pts',(23.0656010870442,0.0137633349813457,
27.2968098467256));
#43848=CARTESIAN_POINT('Ctrl Pts',(23.0974286957389,-0.369895051057782,
27.2058845602728));
#43849=CARTESIAN_POINT('Ctrl Pts',(23.1292563044338,-0.663009057407268,
26.9421700476339));
#43850=CARTESIAN_POINT('Ctrl Pts',(23.152346943891,-0.757917784391792,26.6723232455195));
#43851=CARTESIAN_POINT('Ctrl Pts',(23.1648283804499,-0.764394626155245,
26.5224949099452));
#43852=CARTESIAN_POINT('Ctrl Pts',(23.1667006141106,-0.764371811830445,
26.5000184759214));
#43853=CARTESIAN_POINT('Origin',(8.83329938588935,0.,26.5));
#43854=CARTESIAN_POINT('',(22.2332993858894,-0.764862580106952,26.5002046409345));
#43855=CARTESIAN_POINT('',(22.3667006141106,-0.764412916483386,26.5000055227705));
#43856=CARTESIAN_POINT('',(8.83329938588935,-0.76435,26.5000000000004));
#43857=CARTESIAN_POINT('Ctrl Pts',(22.2332993858894,-0.764862580106872,
26.5002046409345));
#43858=CARTESIAN_POINT('Ctrl Pts',(22.2352427198047,-0.765032394802853,
26.4769375526074));
#43859=CARTESIAN_POINT('Ctrl Pts',(22.2477715892206,-0.759009646591559,
26.3268520087914));
#43860=CARTESIAN_POINT('Ctrl Pts',(22.2708859941369,-0.660332128994326,
26.055748028139));
#43861=CARTESIAN_POINT('Ctrl Pts',(22.3026426006386,-0.369900855742956,
25.7942086605736));
#43862=CARTESIAN_POINT('Ctrl Pts',(22.3343992071401,0.01423446586742,25.7031404697911));
#43863=CARTESIAN_POINT('Ctrl Pts',(22.3661558136418,0.392945955132557,25.8071038457199));
#43864=CARTESIAN_POINT('Ctrl Pts',(22.3979124201434,0.676990688980436,26.0795167243078));
#43865=CARTESIAN_POINT('Ctrl Pts',(22.4296690266449,0.79534519032439,26.4545957758109));
#43866=CARTESIAN_POINT('Ctrl Pts',(22.4614256331466,0.720445109942096,26.8407072374687));
#43867=CARTESIAN_POINT('Ctrl Pts',(22.4931822396481,0.469247428456909,27.1436757375867));
#43868=CARTESIAN_POINT('Ctrl Pts',(22.5249388461498,0.104827792755421,27.290062570161));
#43869=CARTESIAN_POINT('Ctrl Pts',(22.5566954526513,-0.287175811024369,
27.2433021669895));
#43870=CARTESIAN_POINT('Ctrl Pts',(22.5884520591529,-0.605484443472687,
27.0165142048358));
#43871=CARTESIAN_POINT('Ctrl Pts',(22.6139867035656,-0.747869186885517,
26.731375214218));
#43872=CARTESIAN_POINT('Ctrl Pts',(22.6289358124778,-0.764601882514145,
26.5523150654794));
#43873=CARTESIAN_POINT('Ctrl Pts',(22.6332993858894,-0.764122705815501,
26.5000528068419));
#43874=CARTESIAN_POINT('Ctrl Pts',(22.3667006141106,-0.764412916483211,
26.5000055227705));
#43875=CARTESIAN_POINT('Ctrl Pts',(22.376874177558,-0.764365640456866,26.377889443069));
#43876=CARTESIAN_POINT('Ctrl Pts',(22.3976569439038,-0.703489322056653,
26.1283827371445));
#43877=CARTESIAN_POINT('Ctrl Pts',(22.4290489131478,-0.444327578628173,
25.8384349131801));
#43878=CARTESIAN_POINT('Ctrl Pts',(22.4608765218426,-0.0728050701817948,
25.7064038917784));
#43879=CARTESIAN_POINT('Ctrl Pts',(22.4927041305374,0.316538952499552,25.768632477629));
#43880=CARTESIAN_POINT('Ctrl Pts',(22.5245317392322,0.628399313207805,26.0098881103375));
#43881=CARTESIAN_POINT('Ctrl Pts',(22.5563593479271,0.786437594250266,26.3711152779478));
#43882=CARTESIAN_POINT('Ctrl Pts',(22.5881869566219,0.751968557521462,26.7638913597064));
#43883=CARTESIAN_POINT('Ctrl Pts',(22.6200145653167,0.533429670730638,27.0920710663534));
#43884=CARTESIAN_POINT('Ctrl Pts',(22.6518421740115,0.184315750545256,27.2753212658824));
#43885=CARTESIAN_POINT('Ctrl Pts',(22.6836697827063,-0.209915711095263,
27.2687852466482));
#43886=CARTESIAN_POINT('Ctrl Pts',(22.7154973914012,-0.552763171263273,
27.0740629213976));
#43887=CARTESIAN_POINT('Ctrl Pts',(22.7431743352025,-0.733237616757187,
26.7825386072601));
#43888=CARTESIAN_POINT('Ctrl Pts',(22.7602420761057,-0.764252526323207,
26.5775455442021));
#43889=CARTESIAN_POINT('Ctrl Pts',(22.7667006141106,-0.764296184799636,
26.4999878263918));
#43890=CARTESIAN_POINT('Origin',(8.83329938588935,0.,26.5));
#43891=CARTESIAN_POINT('',(21.8332993858894,-0.764100887066997,26.4995051871397));
#43892=CARTESIAN_POINT('',(21.9667006141106,-0.764284603309852,26.5000031825945));
#43893=CARTESIAN_POINT('',(8.83329938588935,-0.76435,26.5000000000004));
#43894=CARTESIAN_POINT('Ctrl Pts',(21.8332993858894,-0.764100887066916,
26.4995051871397));
#43895=CARTESIAN_POINT('Ctrl Pts',(21.8415496271317,-0.764046362726459,
26.4005484505602));
#43896=CARTESIAN_POINT('Ctrl Pts',(21.8603854038745,-0.720456291582594,
26.1754869405762));
#43897=CARTESIAN_POINT('Ctrl Pts',(21.8898067161178,-0.502746680944055,
25.8815879159468));
#43898=CARTESIAN_POINT('Ctrl Pts',(21.9215633226194,-0.146192340398604,
25.7169678142758));
#43899=CARTESIAN_POINT('Ctrl Pts',(21.953319929121,0.246561806406779,25.7421544657884));
#43900=CARTESIAN_POINT('Ctrl Pts',(21.9850765356226,0.578813148913968,25.9526327978489));
#43901=CARTESIAN_POINT('Ctrl Pts',(22.0168331421242,0.770423302724975,26.2961115189095));
#43902=CARTESIAN_POINT('Ctrl Pts',(22.0485897486258,0.773654319674137,26.6896591625013));
#43903=CARTESIAN_POINT('Ctrl Pts',(22.0803463551274,0.589394342448357,27.0364718445485));
#43904=CARTESIAN_POINT('Ctrl Pts',(22.112102961629,0.259548714643134,27.253394002243));
#43905=CARTESIAN_POINT('Ctrl Pts',(22.1438595681306,-0.129993482523563,
27.2851751585385));
#43906=CARTESIAN_POINT('Ctrl Pts',(22.1842583762174,-0.593002042557325,
27.0854711589097));
#43907=CARTESIAN_POINT('Ctrl Pts',(22.2140716488037,-0.763182399309391,
26.7304138981164));
#43908=CARTESIAN_POINT('Ctrl Pts',(22.2332993858894,-0.764862580106872,
26.5002046409345));
#43909=CARTESIAN_POINT('Ctrl Pts',(21.9667006141106,-0.764284603309676,
26.5000031825944));
#43910=CARTESIAN_POINT('Ctrl Pts',(21.9722878732138,-0.764274911934341,
26.4329053576406));
#43911=CARTESIAN_POINT('Ctrl Pts',(21.9884843352154,-0.738916987458651,
26.238393611413));
#43912=CARTESIAN_POINT('Ctrl Pts',(22.0152900001152,-0.575860605727061,
25.9491098802844));
#43913=CARTESIAN_POINT('Ctrl Pts',(22.04711760881,-0.241294757923752,25.7404789660404));
#43914=CARTESIAN_POINT('Ctrl Pts',(22.0789452175048,0.152336179061179,25.7177666270366));
#43915=CARTESIAN_POINT('Ctrl Pts',(22.1107728261996,0.508677661110342,25.8865324798199));
#43916=CARTESIAN_POINT('Ctrl Pts',(22.1426004348944,0.740503004985982,26.2054653486679));
#43917=CARTESIAN_POINT('Ctrl Pts',(22.1744280435892,0.791065082286333,26.5964955792559));
#43918=CARTESIAN_POINT('Ctrl Pts',(22.2062556522841,0.647987106915214,26.9639052387075));
#43919=CARTESIAN_POINT('Ctrl Pts',(22.2380832609789,0.346292273938845,27.2177583313615));
#43920=CARTESIAN_POINT('Ctrl Pts',(22.2699108696737,-0.0401693572021401,
27.2959156889838));
#43921=CARTESIAN_POINT('Ctrl Pts',(22.3017384783685,-0.416798173548772,
27.1792456431623));
#43922=CARTESIAN_POINT('Ctrl Pts',(22.3335660870633,-0.691401477599888,
26.8963071510852));
#43923=CARTESIAN_POINT('Ctrl Pts',(22.3552201323107,-0.763083116198193,
26.6378078686346));
#43924=CARTESIAN_POINT('Ctrl Pts',(22.3662649746598,-0.764414940877344,
26.5052346228955));
#43925=CARTESIAN_POINT('Ctrl Pts',(22.3667006141106,-0.764412916483211,
26.5000055227705));
#43926=CARTESIAN_POINT('Origin',(8.83329938588935,0.,26.5));
#43927=CARTESIAN_POINT('',(21.4332993858894,-0.764276746822807,26.5000737456655));
#43928=CARTESIAN_POINT('',(21.5667006141106,-0.76440089280987,26.4999880930546));
#43929=CARTESIAN_POINT('',(8.83329938588935,-0.76435,26.5000000000004));
#43930=CARTESIAN_POINT('Ctrl Pts',(21.4332993858894,-0.764276746822727,
26.5000737456655));
#43931=CARTESIAN_POINT('Ctrl Pts',(21.4372709989581,-0.764328306924678,
26.4522928960755));
#43932=CARTESIAN_POINT('Ctrl Pts',(21.4518281475273,-0.748306393941852,
26.277170782625));
#43933=CARTESIAN_POINT('Ctrl Pts',(21.476970831597,-0.616487950568337,25.9955654541219));
#43934=CARTESIAN_POINT('Ctrl Pts',(21.5087274380987,-0.299974232084392,
25.7616653616493));
#43935=CARTESIAN_POINT('Ctrl Pts',(21.5404840446002,0.0897151756284967,
25.7084277022228));
#43936=CARTESIAN_POINT('Ctrl Pts',(21.5722406511019,0.457605408654088,25.8475278794664));
#43937=CARTESIAN_POINT('Ctrl Pts',(21.6039972576034,0.713743622414307,26.1463311637505));
#43938=CARTESIAN_POINT('Ctrl Pts',(21.6357538641051,0.796412224677964,26.5302539135788));
#43939=CARTESIAN_POINT('Ctrl Pts',(21.6675104706066,0.684050486030751,26.9087089312087));
#43940=CARTESIAN_POINT('Ctrl Pts',(21.6992670771083,0.406712042690736,27.184093304612));
#43941=CARTESIAN_POINT('Ctrl Pts',(21.7416092191103,-0.0992230806999048,
27.3368617384697));
#43942=CARTESIAN_POINT('Ctrl Pts',(21.7839513611125,-0.609300801297396,
27.0821815203151));
#43943=CARTESIAN_POINT('Ctrl Pts',(21.8180432618723,-0.755762004372405,
26.6826607782934));
#43944=CARTESIAN_POINT('Ctrl Pts',(21.8309640916311,-0.764116320600975,
26.5275156527689));
#43945=CARTESIAN_POINT('Ctrl Pts',(21.8332993858894,-0.764100887066916,
26.4995051871397));
#43946=CARTESIAN_POINT('Ctrl Pts',(21.5667006141106,-0.764400892809695,
26.4999880930546));
#43947=CARTESIAN_POINT('Ctrl Pts',(21.5677015688696,-0.764409844848788,
26.4879728090667));
#43948=CARTESIAN_POINT('Ctrl Pts',(21.5793117265269,-0.761192076692281,
26.3486113254963));
#43949=CARTESIAN_POINT('Ctrl Pts',(21.6015310870826,-0.6805998376932,26.0854168091196));
#43950=CARTESIAN_POINT('Ctrl Pts',(21.6333586957773,-0.398557419114277,
25.8098932365948));
#43951=CARTESIAN_POINT('Ctrl Pts',(21.6651863044722,-0.0189545325561093,
25.7032967384752));
#43952=CARTESIAN_POINT('Ctrl Pts',(21.697013913167,0.36528811976181,25.791720428934));
#43953=CARTESIAN_POINT('Ctrl Pts',(21.7288415218618,0.660114095329825,26.053519605833));
#43954=CARTESIAN_POINT('Ctrl Pts',(21.7606691305566,0.793354720904365,26.4246100268778));
#43955=CARTESIAN_POINT('Ctrl Pts',(21.7924967392514,0.732394826972873,26.8141547049655));
#43956=CARTESIAN_POINT('Ctrl Pts',(21.8243243479463,0.492156418482947,27.126799346661));
#43957=CARTESIAN_POINT('Ctrl Pts',(21.856151956641,0.131446007206347,27.2860135548564));
#43958=CARTESIAN_POINT('Ctrl Pts',(21.8879795653359,-0.261440279771059,
27.2528242433277));
#43959=CARTESIAN_POINT('Ctrl Pts',(21.9198071740307,-0.590330176718207,
27.0353556235666));
#43960=CARTESIAN_POINT('Ctrl Pts',(21.9460475236223,-0.74234810236243,26.7480215032879));
#43961=CARTESIAN_POINT('Ctrl Pts',(21.9616786703156,-0.764293314117844,
26.5603120924657));
#43962=CARTESIAN_POINT('Ctrl Pts',(21.9667006141106,-0.764284603309676,
26.5000031825944));
#43963=CARTESIAN_POINT('Origin',(8.83329938588935,0.,26.5));
#43964=CARTESIAN_POINT('',(21.0332993858894,-0.764351912162959,26.5000528856107));
#43965=CARTESIAN_POINT('',(21.1667006141106,-0.764310404172143,26.500016603693));
#43966=CARTESIAN_POINT('',(8.83329938588935,-0.76435,26.5000000000004));
#43967=CARTESIAN_POINT('Ctrl Pts',(21.0332993858894,-0.764351912162878,
26.5000528856107));
#43968=CARTESIAN_POINT('Ctrl Pts',(21.043577906285,-0.764279841884346,26.376700035302));
#43969=CARTESIAN_POINT('Ctrl Pts',(21.0644419621812,-0.702702321442688,
26.1260397749937));
#43970=CARTESIAN_POINT('Ctrl Pts',(21.0958915535779,-0.441630110964222,
25.8369778582611));
#43971=CARTESIAN_POINT('Ctrl Pts',(21.1276481600795,-0.0707011018639236,
25.70619654051));
#43972=CARTESIAN_POINT('Ctrl Pts',(21.1594047665811,0.317727575909635,25.7695475431092));
#43973=CARTESIAN_POINT('Ctrl Pts',(21.1911613730827,0.628395710084807,26.009789267304));
#43974=CARTESIAN_POINT('Ctrl Pts',(21.2229179795843,0.786429550765298,26.3715608331863));
#43975=CARTESIAN_POINT('Ctrl Pts',(21.2546745860859,0.751894885449026,26.7608685805538));
#43976=CARTESIAN_POINT('Ctrl Pts',(21.297016728088,0.463552958450529,27.2037765581276));
#43977=CARTESIAN_POINT('Ctrl Pts',(21.3393588700901,-0.0905842644351466,
27.3378408441313));
#43978=CARTESIAN_POINT('Ctrl Pts',(21.3817010120923,-0.549496531103895,
27.0757185921867));
#43979=CARTESIAN_POINT('Ctrl Pts',(21.4094860055252,-0.732071494044401,
26.7865804303052));
#43980=CARTESIAN_POINT('Ctrl Pts',(21.4266854634575,-0.76419088384741,26.5796431366029));
#43981=CARTESIAN_POINT('Ctrl Pts',(21.4332993858894,-0.764276746822727,
26.5000737456655));
#43982=CARTESIAN_POINT('Ctrl Pts',(21.1667006141106,-0.764310404171968,
26.500016603693));
#43983=CARTESIAN_POINT('Ctrl Pts',(21.1737244674237,-0.76424402040046,26.4156747594692));
#43984=CARTESIAN_POINT('Ctrl Pts',(21.1913575236351,-0.729295132890033,
26.2038848342813));
#43985=CARTESIAN_POINT('Ctrl Pts',(21.2195997827447,-0.537275894906149,
25.9114169778345));
#43986=CARTESIAN_POINT('Ctrl Pts',(21.2514273914396,-0.189363322650899,
25.7258960707611));
#43987=CARTESIAN_POINT('Ctrl Pts',(21.2832550001344,0.204902355806668,25.7298633979523));
#43988=CARTESIAN_POINT('Ctrl Pts',(21.3150826088292,0.549011221810531,25.9223478213019));
#43989=CARTESIAN_POINT('Ctrl Pts',(21.346910217524,0.758730940462114,26.2562322391823));
#43990=CARTESIAN_POINT('Ctrl Pts',(21.3787378262188,0.782725486097683,26.6497870977146));
#43991=CARTESIAN_POINT('Ctrl Pts',(21.4105654349136,0.615121378538741,27.0066764755672));
#43992=CARTESIAN_POINT('Ctrl Pts',(21.4423930436085,0.296945416897534,27.2395395733916));
#43993=CARTESIAN_POINT('Ctrl Pts',(21.4742206523033,-0.0939180232535311,
27.2913752372527));
#43994=CARTESIAN_POINT('Ctrl Pts',(21.5060482609981,-0.461791836663578,
27.1494949274779));
#43995=CARTESIAN_POINT('Ctrl Pts',(21.5368749149339,-0.708612051316828,
26.8580906911256));
#43996=CARTESIAN_POINT('Ctrl Pts',(21.5570923659713,-0.76431496144049,26.6153238052581));
#43997=CARTESIAN_POINT('Ctrl Pts',(21.5667006141106,-0.764400892809695,
26.4999880930546));
#43998=CARTESIAN_POINT('Origin',(8.83329938588935,0.,26.5));
#43999=CARTESIAN_POINT('',(20.6332993858894,-0.76435,26.5000000000002));
#44000=CARTESIAN_POINT('',(20.7667006141106,-0.764350239829443,26.4999799548752));
#44001=CARTESIAN_POINT('',(8.83329938588935,-0.76435,26.5000000000004));
#44002=CARTESIAN_POINT('Ctrl Pts',(20.6332993858894,-0.764313550173299,
26.5000165829699));
#44003=CARTESIAN_POINT('Ctrl Pts',(20.6392992781114,-0.764263692888945,
26.4279696684704));
#44004=CARTESIAN_POINT('Ctrl Pts',(20.655884705834,-0.736231422484058,26.2287857300863));
#44005=CARTESIAN_POINT('Ctrl Pts',(20.6830556690571,-0.565714119049419,
25.9386711181391));
#44006=CARTESIAN_POINT('Ctrl Pts',(20.7148122755588,-0.227907934100152,
25.7367375432753));
#44007=CARTESIAN_POINT('Ctrl Pts',(20.7465688820603,0.164464593988673,25.7201672434249));
#44008=CARTESIAN_POINT('Ctrl Pts',(20.778325488562,0.518475108459405,25.8948953645883));
#44009=CARTESIAN_POINT('Ctrl Pts',(20.8100820950635,0.743006763321614,26.2147995709279));
#44010=CARTESIAN_POINT('Ctrl Pts',(20.8524242370657,0.808039650977486,26.739279567674));
#44011=CARTESIAN_POINT('Ctrl Pts',(20.8947663790678,0.470788843887705,27.1989568323787));
#44012=CARTESIAN_POINT('Ctrl Pts',(20.9371085210699,-0.0490268475710841,
27.2943517503612));
#44013=CARTESIAN_POINT('Ctrl Pts',(20.9688651275715,-0.421575592023053,
27.1761967746885));
#44014=CARTESIAN_POINT('Ctrl Pts',(21.0006217340731,-0.694507228865489,
26.8909570819885));
#44015=CARTESIAN_POINT('Ctrl Pts',(21.0220998201791,-0.763472476586269,
26.6344550186812));
#44016=CARTESIAN_POINT('Ctrl Pts',(21.0329923707845,-0.764354064871952,
26.5037373836531));
#44017=CARTESIAN_POINT('Ctrl Pts',(21.0332993858894,-0.764351912162878,
26.5000528856107));
#44018=CARTESIAN_POINT('Ctrl Pts',(20.7667006141106,-0.764350239829268,
26.4999799548753));
#44019=CARTESIAN_POINT('Ctrl Pts',(20.7691381630795,-0.764380522761163,
26.4707144501526));
#44020=CARTESIAN_POINT('Ctrl Pts',(20.7821849149467,-0.755557485350515,
26.3140917378046));
#44021=CARTESIAN_POINT('Ctrl Pts',(20.8058408697121,-0.650995855233153,
26.0403264661764));
#44022=CARTESIAN_POINT('Ctrl Pts',(20.8376684784069,-0.350961365800501,
25.7845131161621));
#44023=CARTESIAN_POINT('Ctrl Pts',(20.8694960871017,0.034982840646634,25.7038394872333));
#44024=CARTESIAN_POINT('Ctrl Pts',(20.9013236957965,0.412363808420875,25.8180531906862));
#44025=CARTESIAN_POINT('Ctrl Pts',(20.9331513044914,0.688804725407329,26.0991965425734));
#44026=CARTESIAN_POINT('Ctrl Pts',(20.9649789131862,0.796637286020959,26.4784501566183));
#44027=CARTESIAN_POINT('Ctrl Pts',(20.996806521881,0.70946580780214,26.8629788269146));
#44028=CARTESIAN_POINT('Ctrl Pts',(21.0286341305758,0.448628471403418,27.1586560983357));
#44029=CARTESIAN_POINT('Ctrl Pts',(21.0604617392707,0.0779740759816852,
27.2931049140583));
#44030=CARTESIAN_POINT('Ctrl Pts',(21.0922893479654,-0.311767123444173,
27.2334143589867));
#44031=CARTESIAN_POINT('Ctrl Pts',(21.1241169566603,-0.625192728165132,
26.9941957242612));
#44032=CARTESIAN_POINT('Ctrl Pts',(21.148920712042,-0.750185963151055,26.7134941345636));
#44033=CARTESIAN_POINT('Ctrl Pts',(21.1631152645254,-0.764344289991763,
26.543069182202));
#44034=CARTESIAN_POINT('Ctrl Pts',(21.1667006141106,-0.764310404171968,
26.500016603693));
#44035=CARTESIAN_POINT('Origin',(8.83329938588935,0.,26.5));
#44036=CARTESIAN_POINT('',(20.2332993858894,-0.76435,26.5000000000001));
#44037=CARTESIAN_POINT('',(20.3667006141106,-0.764361315646495,26.5000195227112));
#44038=CARTESIAN_POINT('',(8.83329938588935,-0.76435,26.5000000000004));
#44039=CARTESIAN_POINT('Ctrl Pts',(20.2332993858894,-0.76435,26.5000000000001));
#44040=CARTESIAN_POINT('Ctrl Pts',(20.2511698941678,-0.764350000000042,
26.2854398560099));
#44041=CARTESIAN_POINT('Ctrl Pts',(20.2690404024462,-0.669038051787523,
26.0726183635795));
#44042=CARTESIAN_POINT('Ctrl Pts',(20.2869109107247,-0.508962945483331,
25.9297477377292));
#44043=CARTESIAN_POINT('Ctrl Pts',(20.3047814190031,-0.348887839179139,
25.786877111879));
#44044=CARTESIAN_POINT('Ctrl Pts',(20.3226519272816,-0.126643857468825,
25.716272808144));
#44045=CARTESIAN_POINT('Ctrl Pts',(20.34052243556,0.0865367472361844,25.7405644768134));
#44046=CARTESIAN_POINT('Ctrl Pts',(20.3583929438384,0.299717351941194,25.7648561454827));
#44047=CARTESIAN_POINT('Ctrl Pts',(20.3762634521169,0.500379634244014,25.8836500997623));
#44048=CARTESIAN_POINT('Ctrl Pts',(20.3941339603953,0.62420857318233,26.058871243665));
#44049=CARTESIAN_POINT('Ctrl Pts',(20.4120044686738,0.748037512120647,26.2340923875676));
#44050=CARTESIAN_POINT('Ctrl Pts',(20.4298749769522,0.793026254288736,26.462900971739));
#44051=CARTESIAN_POINT('Ctrl Pts',(20.4477454852306,0.744755289141801,26.6719606984032));
#44052=CARTESIAN_POINT('Ctrl Pts',(20.4656159935091,0.696484323994866,26.8810204250674));
#44053=CARTESIAN_POINT('Ctrl Pts',(20.4834865017875,0.555735962611667,27.0669431344934));
#44054=CARTESIAN_POINT('Ctrl Pts',(20.501357010066,0.367621990370539,27.1701380415228));
#44055=CARTESIAN_POINT('Ctrl Pts',(20.5192275183444,0.179508018129412,27.2733329485522));
#44056=CARTESIAN_POINT('Ctrl Pts',(20.5370980266228,-0.0529228659410256,
27.2921276085011));
#44057=CARTESIAN_POINT('Ctrl Pts',(20.5549685349013,-0.255173367133837,
27.2204980743941));
#44058=CARTESIAN_POINT('Ctrl Pts',(20.5728390431797,-0.457423868326649,
27.148868540287));
#44059=CARTESIAN_POINT('Ctrl Pts',(20.5907095514582,-0.626216181706997,
26.987975687568));
#44060=CARTESIAN_POINT('Ctrl Pts',(20.6085800597366,-0.707450049624308,
26.7893878881131));
#44061=CARTESIAN_POINT('Ctrl Pts',(20.6168198351209,-0.744905549759135,
26.6978225651763));
#44062=CARTESIAN_POINT('Ctrl Pts',(20.6250596105051,-0.764349999999979,
26.5989298885823));
#44063=CARTESIAN_POINT('Ctrl Pts',(20.6332993858894,-0.76435,26.5000000000002));
#44064=CARTESIAN_POINT('Ctrl Pts',(20.3667006141106,-0.764361315646319,
26.5000195227112));
#44065=CARTESIAN_POINT('Ctrl Pts',(20.3751610616335,-0.764255842813653,
26.3984466142992));
#44066=CARTESIAN_POINT('Ctrl Pts',(20.3942307120548,-0.718344923715845,
26.1694111801766));
#44067=CARTESIAN_POINT('Ctrl Pts',(20.4239095653743,-0.496229785355027,
25.8764205252295));
#44068=CARTESIAN_POINT('Ctrl Pts',(20.4557371740691,-0.136564365409659,
25.7148595442031));
#44069=CARTESIAN_POINT('Ctrl Pts',(20.4875647827639,0.256529822285824,25.7454883622458));
#44070=CARTESIAN_POINT('Ctrl Pts',(20.5193923914588,0.586829621236875,25.9608095356299));
#44071=CARTESIAN_POINT('Ctrl Pts',(20.5512200001536,0.773482934822817,26.3081158923556));
#44072=CARTESIAN_POINT('Ctrl Pts',(20.5830476088484,0.77080002362345,26.7023924030459));
#44073=CARTESIAN_POINT('Ctrl Pts',(20.6148752175432,0.579437621297725,27.047126497488));
#44074=CARTESIAN_POINT('Ctrl Pts',(20.646702826238,0.2462381767104,27.2579327948828));
#44075=CARTESIAN_POINT('Ctrl Pts',(20.6785304349328,-0.147236426742641,
27.2832092925066));
#44076=CARTESIAN_POINT('Ctrl Pts',(20.7103580436277,-0.504669912886847,
27.1167687088815));
#44077=CARTESIAN_POINT('Ctrl Pts',(20.7397481033536,-0.720654954004773,
26.8236626255095));
#44078=CARTESIAN_POINT('Ctrl Pts',(20.7585289601812,-0.764248719144938,
26.5980898101897));
#44079=CARTESIAN_POINT('Ctrl Pts',(20.7667006141106,-0.764350239829268,
26.4999799548753));
#44080=CARTESIAN_POINT('Origin',(8.83329938588935,0.,26.5));
#44081=CARTESIAN_POINT('',(19.8332993858894,-0.764344534536135,26.5000129791237));
#44082=CARTESIAN_POINT('',(19.9667006141106,-0.764302553547059,26.4999854764565));
#44083=CARTESIAN_POINT('',(8.83329938588935,-0.76435,26.5000000000004));
#44084=CARTESIAN_POINT('Ctrl Pts',(19.8332993858894,-0.764344534536054,
26.5000129791237));
#44085=CARTESIAN_POINT('Ctrl Pts',(19.8413275572648,-0.764313373082258,
26.403688836108));
#44086=CARTESIAN_POINT('Ctrl Pts',(19.8599412641407,-0.722113350608405,
26.1803405233073));
#44087=CARTESIAN_POINT('Ctrl Pts',(19.8891405065173,-0.508737507276705,
25.8866858826192));
#44088=CARTESIAN_POINT('Ctrl Pts',(19.9208971130188,-0.155477746603945,
25.7194713295494));
#44089=CARTESIAN_POINT('Ctrl Pts',(19.963239255021,0.372447071308012,25.7440463187918));
#44090=CARTESIAN_POINT('Ctrl Pts',(20.0055813970231,0.768489532327075,26.154158088483));
#44091=CARTESIAN_POINT('Ctrl Pts',(20.0479235390252,0.774628079308121,26.6826189306506));
#44092=CARTESIAN_POINT('Ctrl Pts',(20.0796801455268,0.595188665990073,27.0298287551329));
#44093=CARTESIAN_POINT('Ctrl Pts',(20.1114367520284,0.267911625081069,27.2506071489466));
#44094=CARTESIAN_POINT('Ctrl Pts',(20.14319335853,-0.12312173971539,27.2869896069711));
#44095=CARTESIAN_POINT('Ctrl Pts',(20.1749499650316,-0.485029654910406,
27.132351810277));
#44096=CARTESIAN_POINT('Ctrl Pts',(20.2049853074847,-0.714965243557672,
26.8399360103876));
#44097=CARTESIAN_POINT('Ctrl Pts',(20.2244351144373,-0.764312601055636,
26.6063935603332));
#44098=CARTESIAN_POINT('Ctrl Pts',(20.2332993858894,-0.764425095983041,
26.4999881455073));
#44099=CARTESIAN_POINT('Ctrl Pts',(19.9667006141106,-0.764302553546884,
26.4999854764565));
#44100=CARTESIAN_POINT('Ctrl Pts',(19.9705747572893,-0.764334137460401,
26.4534637195935));
#44101=CARTESIAN_POINT('Ctrl Pts',(19.9850581033664,-0.74871078126693,26.2795647520368));
#44102=CARTESIAN_POINT('Ctrl Pts',(20.0101506523417,-0.618409493726067,
25.9973420056359));
#44103=CARTESIAN_POINT('Ctrl Pts',(20.0419782610365,-0.301757468419426,
25.7624108247258));
#44104=CARTESIAN_POINT('Ctrl Pts',(20.0738058697313,0.0887599484803642,
25.7080296515813));
#44105=CARTESIAN_POINT('Ctrl Pts',(20.1056334784261,0.457550352668162,25.8475101257477));
#44106=CARTESIAN_POINT('Ctrl Pts',(20.137461087121,0.71433976430242,26.1467096627914));
#44107=CARTESIAN_POINT('Ctrl Pts',(20.1692886958158,0.796270251327002,26.5323890117207));
#44108=CARTESIAN_POINT('Ctrl Pts',(20.2011163045106,0.683286543729253,26.9101400497234));
#44109=CARTESIAN_POINT('Ctrl Pts',(20.2329439132054,0.403045242186098,27.1874953774243));
#44110=CARTESIAN_POINT('Ctrl Pts',(20.2647715219002,0.0241449255081358,
27.2965628561519));
#44111=CARTESIAN_POINT('Ctrl Pts',(20.296599130595,-0.360665681930769,27.210644515286));
#44112=CARTESIAN_POINT('Ctrl Pts',(20.3284267392899,-0.657191111310729,
26.9507717875409));
#44113=CARTESIAN_POINT('Ctrl Pts',(20.3517939004617,-0.756786585457168,
26.6789681317309));
#44114=CARTESIAN_POINT('Ctrl Pts',(20.3645518587353,-0.76438810327375,26.5258166607872));
#44115=CARTESIAN_POINT('Ctrl Pts',(20.3667006141106,-0.764361315646319,
26.5000195227112));
#44116=CARTESIAN_POINT('Origin',(8.83329938588935,0.,26.5));
#44117=CARTESIAN_POINT('',(19.4332993858894,-0.764277110167821,26.4997254257785));
#44118=CARTESIAN_POINT('',(19.5667006141106,-0.764407967391875,26.5000088022807));
#44119=CARTESIAN_POINT('',(8.83329938588935,-0.76435,26.5000000000004));
#44120=CARTESIAN_POINT('Ctrl Pts',(19.4332993858894,-0.764277110167741,
26.4997254257785));
#44121=CARTESIAN_POINT('Ctrl Pts',(19.4370489290912,-0.764304303637347,
26.4546467689379));
#44122=CARTESIAN_POINT('Ctrl Pts',(19.4513840077936,-0.749338609732044,
26.2824728008134));
#44123=CARTESIAN_POINT('Ctrl Pts',(19.4763046219965,-0.621973401147041,
26.0034645799642));
#44124=CARTESIAN_POINT('Ctrl Pts',(19.5186467639986,-0.202509532859472,
25.6819702461652));
#44125=CARTESIAN_POINT('Ctrl Pts',(19.5609889060007,0.364628407821791,25.7402441752329));
#44126=CARTESIAN_POINT('Ctrl Pts',(19.6033310480029,0.709950204635276,26.1403209180076));
#44127=CARTESIAN_POINT('Ctrl Pts',(19.6350876545045,0.796560342324164,26.5214401241865));
#44128=CARTESIAN_POINT('Ctrl Pts',(19.6668442610061,0.688648014289257,26.9011877905904));
#44129=CARTESIAN_POINT('Ctrl Pts',(19.6986008675076,0.413135351067633,27.1810512359355));
#44130=CARTESIAN_POINT('Ctrl Pts',(19.7303574740093,0.0367650668537481,
27.2960972980499));
#44131=CARTESIAN_POINT('Ctrl Pts',(19.7621140805108,-0.348389341911593,
27.2164219300026));
#44132=CARTESIAN_POINT('Ctrl Pts',(19.7938706870124,-0.64889140428939,26.962668913525));
#44133=CARTESIAN_POINT('Ctrl Pts',(19.8175991221386,-0.754929961758368,
26.6883853153909));
#44134=CARTESIAN_POINT('Ctrl Pts',(19.8307420217643,-0.764354460978864,
26.5306969165001));
#44135=CARTESIAN_POINT('Ctrl Pts',(19.8332993858894,-0.764344534536054,
26.5000129791237));
#44136=CARTESIAN_POINT('Ctrl Pts',(19.5667006141106,-0.7644079673917,26.5000088022807));
#44137=CARTESIAN_POINT('Ctrl Pts',(19.5765976558434,-0.764338862078803,
26.3812096529835));
#44138=CARTESIAN_POINT('Ctrl Pts',(19.5971039004745,-0.706022523705182,
26.1349974549268));
#44139=CARTESIAN_POINT('Ctrl Pts',(19.6282193480038,-0.452910319833234,
25.8442808501979));
#44140=CARTESIAN_POINT('Ctrl Pts',(19.6600469566987,-0.0831397717704243,
25.7074199475267));
#44141=CARTESIAN_POINT('Ctrl Pts',(19.6918745653935,0.306982059827983,25.7645699379462));
#44142=CARTESIAN_POINT('Ctrl Pts',(19.7237021740883,0.621959603598031,26.0017414198222));
#44143=CARTESIAN_POINT('Ctrl Pts',(19.7555297827831,0.784691405396808,26.3608786158601));
#44144=CARTESIAN_POINT('Ctrl Pts',(19.787357391478,0.755343328467109,26.7540704968485));
#44145=CARTESIAN_POINT('Ctrl Pts',(19.8191850001728,0.54109931163992,27.0850699925406));
#44146=CARTESIAN_POINT('Ctrl Pts',(19.8510126088676,0.194402856255303,27.2728537317685));
#44147=CARTESIAN_POINT('Ctrl Pts',(19.8828402175624,-0.199880302382556,
27.2714552650336));
#44148=CARTESIAN_POINT('Ctrl Pts',(19.9146678262572,-0.545235966749666,
27.0812169145776));
#44149=CARTESIAN_POINT('Ctrl Pts',(19.9426212917733,-0.731334700262787,
26.7891801156537));
#44150=CARTESIAN_POINT('Ctrl Pts',(19.9599655543911,-0.764247646039883,
26.5808618912586));
#44151=CARTESIAN_POINT('Ctrl Pts',(19.9667006141106,-0.764302553546884,
26.4999854764565));
#44152=CARTESIAN_POINT('Origin',(8.83329938588935,0.,26.5));
#44153=CARTESIAN_POINT('',(19.0332993858894,-0.764142366123107,26.5004047868447));
#44154=CARTESIAN_POINT('',(19.1667006141106,-0.764283845776008,26.5000000693701));
#44155=CARTESIAN_POINT('',(8.83329938588935,-0.76435,26.5000000000004));
#44156=CARTESIAN_POINT('Ctrl Pts',(19.0332993858894,-0.764142366123026,
26.5004047868447));
#44157=CARTESIAN_POINT('Ctrl Pts',(19.0433558364182,-0.764299595706694,
26.3793772227263));
#44158=CARTESIAN_POINT('Ctrl Pts',(19.074583357948,-0.676215978146822,26.0010972569083));
#44159=CARTESIAN_POINT('Ctrl Pts',(19.1163964149784,-0.210938010442085,
25.6841029814942));
#44160=CARTESIAN_POINT('Ctrl Pts',(19.1587385569805,0.310953319631399,25.7673975374766));
#44161=CARTESIAN_POINT('Ctrl Pts',(19.1904951634821,0.622827872514436,26.002955234302));
#44162=CARTESIAN_POINT('Ctrl Pts',(19.2222517699837,0.78509669838758,26.3628471470069));
#44163=CARTESIAN_POINT('Ctrl Pts',(19.2540083764853,0.754844992184846,26.7544025197296));
#44164=CARTESIAN_POINT('Ctrl Pts',(19.2857649829869,0.54124693951236,27.0849566894835));
#44165=CARTESIAN_POINT('Ctrl Pts',(19.3175215894885,0.195421936564938,27.2722990237309));
#44166=CARTESIAN_POINT('Ctrl Pts',(19.3492781959901,-0.197887083474027,
27.2719865803867));
#44167=CARTESIAN_POINT('Ctrl Pts',(19.3810348024917,-0.542997981900108,
27.0828076834802));
#44168=CARTESIAN_POINT('Ctrl Pts',(19.4090418657915,-0.730711463169429,
26.7917336743709));
#44169=CARTESIAN_POINT('Ctrl Pts',(19.4264633935907,-0.764227532302173,
26.5819107306037));
#44170=CARTESIAN_POINT('Ctrl Pts',(19.4332993858894,-0.764277110167741,
26.4997254257785));
#44171=CARTESIAN_POINT('Ctrl Pts',(19.1667006141106,-0.764283845936459,
26.50000006937));
#44172=CARTESIAN_POINT('Ctrl Pts',(19.1720113514992,-0.764283645388312,
26.4362228342538));
#44173=CARTESIAN_POINT('Ctrl Pts',(19.1879312917861,-0.740620064377401,
26.245038357094));
#44174=CARTESIAN_POINT('Ctrl Pts',(19.2144604349712,-0.582990039655113,
25.956660350341));
#44175=CARTESIAN_POINT('Ctrl Pts',(19.2462880436661,-0.251171142649758,
25.7436876185539));
#44176=CARTESIAN_POINT('Ctrl Pts',(19.2781156523609,0.142130424215859,25.7158480353013));
#44177=CARTESIAN_POINT('Ctrl Pts',(19.3099432610557,0.500640741350412,25.8799562843406));
#44178=CARTESIAN_POINT('Ctrl Pts',(19.3417708697505,0.736602229450057,26.1958412966923));
#44179=CARTESIAN_POINT('Ctrl Pts',(19.3735984784453,0.792255298302605,26.58617948445));
#44180=CARTESIAN_POINT('Ctrl Pts',(19.4054260871402,0.653976968680098,26.9554223157297));
#44181=CARTESIAN_POINT('Ctrl Pts',(19.437253695835,0.355615559299935,27.2131850637895));
#44182=CARTESIAN_POINT('Ctrl Pts',(19.4690813045298,-0.0297948390643188,
27.2963715394172));
#44183=CARTESIAN_POINT('Ctrl Pts',(19.5009089132246,-0.407911938387894,
27.1846190267216));
#44184=CARTESIAN_POINT('Ctrl Pts',(19.5327365219194,-0.686178733351599,
26.9052827496015));
#44185=CARTESIAN_POINT('Ctrl Pts',(19.5546670888814,-0.762180946991868,
26.6444506321226));
#44186=CARTESIAN_POINT('Ctrl Pts',(19.5659884529451,-0.764412940000839,
26.5085572294674));
#44187=CARTESIAN_POINT('Ctrl Pts',(19.5667006141106,-0.7644079673917,26.5000088022807));
#44188=CARTESIAN_POINT('Origin',(8.83329938588935,0.,26.5));
#44189=CARTESIAN_POINT('',(18.6332993858894,-0.763975585123095,26.5000842874006));
#44190=CARTESIAN_POINT('',(18.7667006141106,-0.76440770353066,26.4999910584554));
#44191=CARTESIAN_POINT('',(8.83329938588935,-0.76435,26.5000000000004));
#44192=CARTESIAN_POINT('Ctrl Pts',(18.6332993858894,-0.763975585123014,
26.5000842874006));
#44193=CARTESIAN_POINT('Ctrl Pts',(18.6496627437451,-0.762198505857026,
26.3040649899126));
#44194=CARTESIAN_POINT('Ctrl Pts',(18.6766116371014,-0.635771178646696,
25.981206808511));
#44195=CARTESIAN_POINT('Ctrl Pts',(18.7141460659582,-0.234472997417264,
25.7394602274647));
#44196=CARTESIAN_POINT('Ctrl Pts',(18.7459026724598,0.155802722384311,25.7185311453641));
#44197=CARTESIAN_POINT('Ctrl Pts',(18.7776592789614,0.511839522475942,25.8890924505991));
#44198=CARTESIAN_POINT('Ctrl Pts',(18.8094158854629,0.741094448594219,26.2079544172491));
#44199=CARTESIAN_POINT('Ctrl Pts',(18.8411724919646,0.790852991429545,26.5983571259894));
#44200=CARTESIAN_POINT('Ctrl Pts',(18.8729290984662,0.647208072939979,26.964496744374));
#44201=CARTESIAN_POINT('Ctrl Pts',(18.9046857049677,0.346303229108121,27.2177720053648));
#44202=CARTESIAN_POINT('Ctrl Pts',(18.9364423114694,-0.0394890010879801,
27.2955829454142));
#44203=CARTESIAN_POINT('Ctrl Pts',(18.9681989179709,-0.414953219279804,
27.1804421773526));
#44204=CARTESIAN_POINT('Ctrl Pts',(18.9999555244725,-0.690495493529877,
26.8977235614153));
#44205=CARTESIAN_POINT('Ctrl Pts',(19.0216556804454,-0.762301751285678,
26.640488566984));
#44206=CARTESIAN_POINT('Ctrl Pts',(19.0327703009176,-0.764134094038398,
26.5067722288323));
#44207=CARTESIAN_POINT('Ctrl Pts',(19.0332993858894,-0.764142366123026,
26.5004047868447));
#44208=CARTESIAN_POINT('Ctrl Pts',(18.7667006141106,-0.764407703530485,
26.4999910584554));
#44209=CARTESIAN_POINT('Ctrl Pts',(18.767425047155,-0.764412829262714,26.4912953170418));
#44210=CARTESIAN_POINT('Ctrl Pts',(18.7787586830977,-0.762139897682738,
26.3552545553671));
#44211=CARTESIAN_POINT('Ctrl Pts',(18.8007015219386,-0.685944244027812,
26.0943205018872));
#44212=CARTESIAN_POINT('Ctrl Pts',(18.8325291306334,-0.407515955991956,
25.8151451928656));
#44213=CARTESIAN_POINT('Ctrl Pts',(18.8643567393282,-0.0293342934702721,
25.7036113634181));
#44214=CARTESIAN_POINT('Ctrl Pts',(18.8961843480231,0.356027933769703,25.7870207074674));
#44215=CARTESIAN_POINT('Ctrl Pts',(18.9280119567179,0.654240229440685,26.0449559544106));
#44216=CARTESIAN_POINT('Ctrl Pts',(18.9598395654127,0.792305003299414,26.4142786901237));
#44217=CARTESIAN_POINT('Ctrl Pts',(18.9916671741075,0.736426211717768,26.8045846285138));
#44218=CARTESIAN_POINT('Ctrl Pts',(19.0234947828023,0.500282087197375,27.1203331318392));
#44219=CARTESIAN_POINT('Ctrl Pts',(19.0553223914972,0.141676926436067,27.2842340274076));
#44220=CARTESIAN_POINT('Ctrl Pts',(19.087150000192,-0.25160847507182,27.2561670030497));
#44221=CARTESIAN_POINT('Ctrl Pts',(19.1189776088868,-0.5833041547505,27.0430024164579));
#44222=CARTESIAN_POINT('Ctrl Pts',(19.145494480193,-0.740694544999679,26.7546667410442));
#44223=CARTESIAN_POINT('Ctrl Pts',(19.1614021486009,-0.764284046021185,
26.5636299301288));
#44224=CARTESIAN_POINT('Ctrl Pts',(19.1667006141106,-0.764283845936459,
26.50000006937));
#44225=CARTESIAN_POINT('Origin',(8.83329938588935,0.,26.5));
#44226=CARTESIAN_POINT('',(18.2332993858894,-0.764965412428307,26.5002633677415));
#44227=CARTESIAN_POINT('',(18.3667006141106,-0.764302619722667,26.5000145152404));
#44228=CARTESIAN_POINT('',(8.83329938588935,-0.76435,26.5000000000004));
#44229=CARTESIAN_POINT('Ctrl Pts',(18.2332993858894,-0.764965412428226,
26.5002633677415));
#44230=CARTESIAN_POINT('Ctrl Pts',(18.234798580071,-0.76508119305691,26.4823116736568));
#44231=CARTESIAN_POINT('Ctrl Pts',(18.2468833097532,-0.760677492458328,
26.3375307285701));
#44232=CARTESIAN_POINT('Ctrl Pts',(18.2695535749358,-0.669488757599245,
26.0696595117695));
#44233=CARTESIAN_POINT('Ctrl Pts',(18.3013101814374,-0.38458849635973,25.8021075061857));
#44234=CARTESIAN_POINT('Ctrl Pts',(18.333066787939,-0.00244655372769168,
25.7030155094137));
#44235=CARTESIAN_POINT('Ctrl Pts',(18.3648233944406,0.378359542695009,25.7990328449791));
#44236=CARTESIAN_POINT('Ctrl Pts',(18.3965800009422,0.668042185748427,26.0654402662492));
#44237=CARTESIAN_POINT('Ctrl Pts',(18.4283366074438,0.794220949673334,26.4379609214166));
#44238=CARTESIAN_POINT('Ctrl Pts',(18.4600932139454,0.7274175711474,26.8255549708114));
#44239=CARTESIAN_POINT('Ctrl Pts',(18.491849820447,0.482615591725175,27.1337143882872));
#44240=CARTESIAN_POINT('Ctrl Pts',(18.5236064269486,0.121339288012704,27.2876956564317));
#44241=CARTESIAN_POINT('Ctrl Pts',(18.5553630334502,-0.271557026497766,
27.2491494235501));
#44242=CARTESIAN_POINT('Ctrl Pts',(18.5871196399518,-0.594542196765398,
27.0290726886231));
#44243=CARTESIAN_POINT('Ctrl Pts',(18.6130984240982,-0.745442993191746,
26.7420693134418));
#44244=CARTESIAN_POINT('Ctrl Pts',(18.6284916727441,-0.764497708236297,
26.5576766569852));
#44245=CARTESIAN_POINT('Ctrl Pts',(18.6332993858894,-0.763975585123014,
26.5000842874006));
#44246=CARTESIAN_POINT('Ctrl Pts',(18.3667006141106,-0.764302619722492,
26.5000145152404));
#44247=CARTESIAN_POINT('Ctrl Pts',(18.373447945709,-0.764247307603586,26.4189908696697));
#44248=CARTESIAN_POINT('Ctrl Pts',(18.3908044802058,-0.731249504241009,
26.2105253289262));
#44249=CARTESIAN_POINT('Ctrl Pts',(18.4187702176008,-0.544899508122728,
25.9184677654519));
#44250=CARTESIAN_POINT('Ctrl Pts',(18.4505978262956,-0.199434270097742,
25.7284293306239));
#44251=CARTESIAN_POINT('Ctrl Pts',(18.4824254349904,0.194849834271444,25.7272587900961));
#44252=CARTESIAN_POINT('Ctrl Pts',(18.5142530436853,0.541437529129979,25.9152430383213));
#44253=CARTESIAN_POINT('Ctrl Pts',(18.5460806523801,0.755490150492264,26.2463663511633));
#44254=CARTESIAN_POINT('Ctrl Pts',(18.5779082610749,0.784610810040825,26.639575151346));
#44255=CARTESIAN_POINT('Ctrl Pts',(18.6097358697697,0.621671362865706,26.9986181728724));
#44256=CARTESIAN_POINT('Ctrl Pts',(18.6415634784645,0.306556707364476,27.2356074676479));
#44257=CARTESIAN_POINT('Ctrl Pts',(18.6733910871593,-0.0835981042838541,
27.2925318396574));
#44258=CARTESIAN_POINT('Ctrl Pts',(18.7052186958542,-0.453289446413202,
27.1554571230883));
#44259=CARTESIAN_POINT('Ctrl Pts',(18.7363218715046,-0.706133725022458,
26.8647089078388));
#44260=CARTESIAN_POINT('Ctrl Pts',(18.7568158442567,-0.764337763756458,
26.6186430211802));
#44261=CARTESIAN_POINT('Ctrl Pts',(18.7667006141106,-0.764407703530485,
26.4999910584554));
#44262=CARTESIAN_POINT('Origin',(8.83329938588935,0.,26.5));
#44263=CARTESIAN_POINT('',(17.8332993858894,-0.7642638282056,26.5001069462646));
#44264=CARTESIAN_POINT('',(17.9667006141106,-0.764094264662737,26.499903563092));
#44265=CARTESIAN_POINT('',(8.83329938588935,-0.76435,26.5000000000004));
#44266=CARTESIAN_POINT('Ctrl Pts',(17.8332993858894,-0.764263828205519,
26.5001069462646));
#44267=CARTESIAN_POINT('Ctrl Pts',(17.841105487398,-0.764502135910798,26.4059835619486));
#44268=CARTESIAN_POINT('Ctrl Pts',(17.8700826599076,-0.702119382636757,
26.0558542073795));
#44269=CARTESIAN_POINT('Ctrl Pts',(17.9096453679177,-0.29613832160412,25.711027047467));
#44270=CARTESIAN_POINT('Ctrl Pts',(17.9519875099199,0.231694148623007,25.7385828611072));
#44271=CARTESIAN_POINT('Ctrl Pts',(17.9837441164214,0.566653359359628,25.9398584184328));
#44272=CARTESIAN_POINT('Ctrl Pts',(18.0155007229231,0.766296209055916,26.2804493550768));
#44273=CARTESIAN_POINT('Ctrl Pts',(18.0472573294246,0.777290647856074,26.673205973088));
#44274=CARTESIAN_POINT('Ctrl Pts',(18.0790139359263,0.6005784561905,27.0241353676862));
#44275=CARTESIAN_POINT('Ctrl Pts',(18.1107705424278,0.275214785933559,27.2477375493297));
#44276=CARTESIAN_POINT('Ctrl Pts',(18.1425271489295,-0.113511804048443,
27.2877520601354));
#44277=CARTESIAN_POINT('Ctrl Pts',(18.1833700967499,-0.585770293594626,
27.095643467088));
#44278=CARTESIAN_POINT('Ctrl Pts',(18.2136275090699,-0.763446181435014,
26.7358189208944));
#44279=CARTESIAN_POINT('Ctrl Pts',(18.2332993858894,-0.764965412428226,
26.5002633677415));
#44280=CARTESIAN_POINT('Ctrl Pts',(17.9667006141106,-0.764094264662562,
26.499903563092));
#44281=CARTESIAN_POINT('Ctrl Pts',(17.9688616413648,-0.763991946430581,
26.4738963283246));
#44282=CARTESIAN_POINT('Ctrl Pts',(17.9816318715174,-0.755722265230173,
26.3202837748946));
#44283=CARTESIAN_POINT('Ctrl Pts',(18.0050113045682,-0.657888459085232,
26.0492639960516));
#44284=CARTESIAN_POINT('Ctrl Pts',(18.036838913263,-0.35974177500854,25.7889256783384));
#44285=CARTESIAN_POINT('Ctrl Pts',(18.0686665219578,0.0243332818644455,
25.7035686117623));
#44286=CARTESIAN_POINT('Ctrl Pts',(18.1004941306526,0.403587040260669,25.8126756400868));
#44287=CARTESIAN_POINT('Ctrl Pts',(18.1323217393475,0.683447187528216,26.0902880943639));
#44288=CARTESIAN_POINT('Ctrl Pts',(18.1641493480422,0.796329325103614,26.468054034611));
#44289=CARTESIAN_POINT('Ctrl Pts',(18.1959769567371,0.71411390092001,26.8537126167479));
#44290=CARTESIAN_POINT('Ctrl Pts',(18.2278045654319,0.457184295086093,27.1527494739896));
#44291=CARTESIAN_POINT('Ctrl Pts',(18.2596321741268,0.0882959257025597,
27.2920241365189));
#44292=CARTESIAN_POINT('Ctrl Pts',(18.2914597828215,-0.302180780501247,
27.237413173922));
#44293=CARTESIAN_POINT('Ctrl Pts',(18.3232873915164,-0.618701763158597,
27.0023010116041));
#44294=CARTESIAN_POINT('Ctrl Pts',(18.3483676686127,-0.748774141274869,
26.7201401454704));
#44295=CARTESIAN_POINT('Ctrl Pts',(18.3628387428108,-0.764334277909349,
26.5463888317932));
#44296=CARTESIAN_POINT('Ctrl Pts',(18.3667006141106,-0.764302619722492,
26.5000145152404));
#44297=CARTESIAN_POINT('Origin',(8.83329938588935,0.,26.5));
#44298=CARTESIAN_POINT('',(17.4332993858894,-0.76329981703839,26.5001479671982));
#44299=CARTESIAN_POINT('',(17.5667006141106,-0.764350395671289,26.5000203280756));
#44300=CARTESIAN_POINT('',(8.83329938588935,-0.76435,26.5000000000004));
#44301=CARTESIAN_POINT('Ctrl Pts',(17.4332993858894,-0.763299817038309,
26.5001479671982));
#44302=CARTESIAN_POINT('Ctrl Pts',(17.4474123947249,-0.762135941631699,
26.3309054434457));
#44303=CARTESIAN_POINT('Ctrl Pts',(17.472110939061,-0.664721913465502,26.0344563923922));
#44304=CARTESIAN_POINT('Ctrl Pts',(17.5073950188975,-0.313656364480858,
25.7685507409244));
#44305=CARTESIAN_POINT('Ctrl Pts',(17.5391516253991,0.072211731487986,25.7064298750071));
#44306=CARTESIAN_POINT('Ctrl Pts',(17.5709082319007,0.444301753746512,25.8383478091969));
#44307=CARTESIAN_POINT('Ctrl Pts',(17.6026648384023,0.70601938612131,26.1311526579745));
#44308=CARTESIAN_POINT('Ctrl Pts',(17.6344214449039,0.796820980869681,26.5140956120801));
#44309=CARTESIAN_POINT('Ctrl Pts',(17.6661780514055,0.692738004319475,26.8933825384317));
#44310=CARTESIAN_POINT('Ctrl Pts',(17.6979346579071,0.420331066798412,27.1770851633445));
#44311=CARTESIAN_POINT('Ctrl Pts',(17.7296912644087,0.0449434652133512,
27.2952930157502));
#44312=CARTESIAN_POINT('Ctrl Pts',(17.7614478709103,-0.34060148631374,27.2205420816171));
#44313=CARTESIAN_POINT('Ctrl Pts',(17.7932044774119,-0.644515709678365,
26.9685741610806));
#44314=CARTESIAN_POINT('Ctrl Pts',(17.8171549824049,-0.753381002992764,
26.6946505652555));
#44315=CARTESIAN_POINT('Ctrl Pts',(17.8305199518974,-0.764178976562752,
26.5336204399747));
#44316=CARTESIAN_POINT('Ctrl Pts',(17.8332993858894,-0.764263828205519,
26.5001069462646));
#44317=CARTESIAN_POINT('Ctrl Pts',(17.5667006141106,-0.764350395671114,
26.5000203280756));
#44318=CARTESIAN_POINT('Ctrl Pts',(17.5748845399189,-0.764254594178374,
26.4017577472398));
#44319=CARTESIAN_POINT('Ctrl Pts',(17.5936776686255,-0.720583009812041,
26.1760195175961));
#44320=CARTESIAN_POINT('Ctrl Pts',(17.6230800002304,-0.504252400540365,
25.882996417912));
#44321=CARTESIAN_POINT('Ctrl Pts',(17.6549076089252,-0.146898168000676,
25.7165983131021));
#44322=CARTESIAN_POINT('Ctrl Pts',(17.68673521762,0.246892880351082,25.7424124008351));
#44323=CARTESIAN_POINT('Ctrl Pts',(17.7185628263148,0.579346349872695,25.9528266796507));
#44324=CARTESIAN_POINT('Ctrl Pts',(17.7503904350096,0.771677592213418,26.2987691287884));
#44325=CARTESIAN_POINT('Ctrl Pts',(17.7822180437045,0.772008340680367,26.6910250850529));
#44326=CARTESIAN_POINT('Ctrl Pts',(17.8246548552975,0.527363192762192,27.1585233970218));
#44327=CARTESIAN_POINT('Ctrl Pts',(17.8777008697889,-0.155425403013523,
27.3905262878577));
#44328=CARTESIAN_POINT('Ctrl Pts',(17.928585857026,-0.696286520605016,26.9592635474336));
#44329=CARTESIAN_POINT('Ctrl Pts',(17.9582524384666,-0.764494260726312,
26.6015745100437));
#44330=CARTESIAN_POINT('Ctrl Pts',(17.9667006141106,-0.764094264662562,
26.499903563092));
#44331=CARTESIAN_POINT('Origin',(8.83329938588935,0.,26.5));
#44332=CARTESIAN_POINT('',(17.0332993858894,-0.765203811462457,26.5004911225311));
#44333=CARTESIAN_POINT('',(17.1667006141106,-0.764310045233437,26.4999834783144));
#44334=CARTESIAN_POINT('',(8.83329938588935,-0.76435,26.5000000000004));
#44335=CARTESIAN_POINT('Ctrl Pts',(17.0332993858894,-0.765203811462376,
26.5004911225311));
#44336=CARTESIAN_POINT('Ctrl Pts',(17.0431337665513,-0.76521128941822,26.382487512764));
#44337=CARTESIAN_POINT('Ctrl Pts',(17.0635536827138,-0.705242476473079,
26.1359384245521));
#44338=CARTESIAN_POINT('Ctrl Pts',(17.0945591343768,-0.456300068822577,
25.846732592974));
#44339=CARTESIAN_POINT('Ctrl Pts',(17.1263157408784,-0.0867895361857581,
25.7077530010661));
#44340=CARTESIAN_POINT('Ctrl Pts',(17.1580723473799,0.30203843095996,25.7629217202603));
#44341=CARTESIAN_POINT('Ctrl Pts',(17.1898289538815,0.618293167806677,25.9971718615475));
#44342=CARTESIAN_POINT('Ctrl Pts',(17.2215855603831,0.78319257186756,26.3542436602263));
#44343=CARTESIAN_POINT('Ctrl Pts',(17.2533421668847,0.757790262318726,26.7467316287404));
#44344=CARTESIAN_POINT('Ctrl Pts',(17.2850987733863,0.546980915086662,27.0790712241793));
#44345=CARTESIAN_POINT('Ctrl Pts',(17.316855379888,0.20403256237055,27.2704274425122));
#44346=CARTESIAN_POINT('Ctrl Pts',(17.3486119863895,-0.190736679054125,
27.2736844177905));
#44347=CARTESIAN_POINT('Ctrl Pts',(17.3803685928912,-0.535201811279513,
27.0890308594029));
#44348=CARTESIAN_POINT('Ctrl Pts',(17.4085977260577,-0.731262683123162,
26.7962743064247));
#44349=CARTESIAN_POINT('Ctrl Pts',(17.4262413237238,-0.763881883206379,
26.5847879095112));
#44350=CARTESIAN_POINT('Ctrl Pts',(17.4332993858894,-0.763299817038309,
26.5001479671982));
#44351=CARTESIAN_POINT('Ctrl Pts',(17.1667006141106,-0.764310045233262,
26.4999834783144));
#44352=CARTESIAN_POINT('Ctrl Pts',(17.1702982355747,-0.764343861225088,
26.4567834827247));
#44353=CARTESIAN_POINT('Ctrl Pts',(17.1845050599371,-0.750124293143909,
26.2862109162653));
#44354=CARTESIAN_POINT('Ctrl Pts',(17.2093210871977,-0.624906846574195,
26.0054427956063));
#44355=CARTESIAN_POINT('Ctrl Pts',(17.2411486958926,-0.311342909206791,
25.7664054968385));
#44356=CARTESIAN_POINT('Ctrl Pts',(17.2729763045874,0.0784326585839467,
25.7069402585764));
#44357=CARTESIAN_POINT('Ctrl Pts',(17.3048039132822,0.449009401771598,25.8416035517627));
#44358=CARTESIAN_POINT('Ctrl Pts',(17.336631521977,0.709675400200942,26.1374313304758));
#44359=CARTESIAN_POINT('Ctrl Pts',(17.3684591306719,0.796625066564042,26.5220108860288));
#44360=CARTESIAN_POINT('Ctrl Pts',(17.4002867393666,0.688572116174983,26.9012010606094));
#44361=CARTESIAN_POINT('Ctrl Pts',(17.4321143480615,0.411970711104484,27.1821864196729));
#44362=CARTESIAN_POINT('Ctrl Pts',(17.4639419567563,0.0345198850269114,
27.296178240544));
#44363=CARTESIAN_POINT('Ctrl Pts',(17.4957695654511,-0.351370292731717,
27.2152882780459));
#44364=CARTESIAN_POINT('Ctrl Pts',(17.5275971741459,-0.651270599572141,
26.9592885385028));
#44365=CARTESIAN_POINT('Ctrl Pts',(17.5512408570324,-0.75560037060335,26.6856230225073));
#44366=CARTESIAN_POINT('Ctrl Pts',(17.5642753370206,-0.764378786100226,
26.5291400918272));
#44367=CARTESIAN_POINT('Ctrl Pts',(17.5667006141106,-0.764350395671114,
26.5000203280756));
#44368=CARTESIAN_POINT('Origin',(8.83329938588935,0.,26.5));
#44369=CARTESIAN_POINT('',(16.6332993858894,-0.764172016402676,26.4996705939536));
#44370=CARTESIAN_POINT('',(16.7667006141106,-0.764401227565655,26.5000117829436));
#44371=CARTESIAN_POINT('',(8.83329938588935,-0.76435,26.5000000000004));
#44372=CARTESIAN_POINT('Ctrl Pts',(16.6332993858894,-0.764172016402596,
26.4996705939536));
#44373=CARTESIAN_POINT('Ctrl Pts',(16.6388551383777,-0.76423249137171,26.4331523910536));
#44374=CARTESIAN_POINT('Ctrl Pts',(16.6549964263666,-0.739381154229132,
26.2401092740816));
#44375=CARTESIAN_POINT('Ctrl Pts',(16.681723249856,-0.577011248722235,25.9502311851775));
#44376=CARTESIAN_POINT('Ctrl Pts',(16.7134798563576,-0.244173820480448,
25.7417844965558));
#44377=CARTESIAN_POINT('Ctrl Pts',(16.7452364628592,0.148607952543154,25.7170324051763));
#44378=CARTESIAN_POINT('Ctrl Pts',(16.7769930693608,0.504838200497434,25.8837420128997));
#44379=CARTESIAN_POINT('Ctrl Pts',(16.8087496758624,0.738401842223993,26.2001912317773));
#44380=CARTESIAN_POINT('Ctrl Pts',(16.840506282364,0.791443309939019,26.5901614741675));
#44381=CARTESIAN_POINT('Ctrl Pts',(16.8722628888656,0.652584945679744,26.9575157041844));
#44382=CARTESIAN_POINT('Ctrl Pts',(16.9040194953672,0.352864424260747,27.2144611647807));
#44383=CARTESIAN_POINT('Ctrl Pts',(16.9357761018688,-0.0295172027510032,
27.2953157045016));
#44384=CARTESIAN_POINT('Ctrl Pts',(16.9781182438709,-0.537397266224523,
27.1491432563852));
#44385=CARTESIAN_POINT('Ctrl Pts',(17.0106260052111,-0.760267862974393,
26.7724256846253));
#44386=CARTESIAN_POINT('Ctrl Pts',(17.0325482310508,-0.765203240292426,
26.5095042963645));
#44387=CARTESIAN_POINT('Ctrl Pts',(17.0332993858894,-0.765203811462376,
26.5004911225311));
#44388=CARTESIAN_POINT('Ctrl Pts',(16.7667006141106,-0.764401227565479,
26.5000117829436));
#44389=CARTESIAN_POINT('Ctrl Pts',(16.7763211341288,-0.764315896056895,
26.3845289078875));
#44390=CARTESIAN_POINT('Ctrl Pts',(16.7965508570452,-0.708503173963334,
26.1416155285519));
#44391=CARTESIAN_POINT('Ctrl Pts',(16.8273897828599,-0.461416157419982,
25.8502381275293));
#44392=CARTESIAN_POINT('Ctrl Pts',(16.8592173915548,-0.0934603563117058,
25.7085705824253));
#44393=CARTESIAN_POINT('Ctrl Pts',(16.8910450002496,0.29737304194578,25.7606322733754));
#44394=CARTESIAN_POINT('Ctrl Pts',(16.9228726089444,0.615414286049196,25.9936793330608));
#44395=CARTESIAN_POINT('Ctrl Pts',(16.9547002176392,0.782811976792353,26.3506655763249));
#44396=CARTESIAN_POINT('Ctrl Pts',(16.986527826334,0.758589843209824,26.7442064932981));
#44397=CARTESIAN_POINT('Ctrl Pts',(17.0183554350289,0.548677074193156,27.0779695742253));
#44398=CARTESIAN_POINT('Ctrl Pts',(17.0501830437237,0.204456953247554,27.270254968634));
#44399=CARTESIAN_POINT('Ctrl Pts',(17.0820106524185,-0.189810955467986,
27.273994290092));
#44400=CARTESIAN_POINT('Ctrl Pts',(17.1138382611133,-0.537616179499631,
27.0882722200051));
#44401=CARTESIAN_POINT('Ctrl Pts',(17.142068248344,-0.729382894522571,26.7958204943258));
#44402=CARTESIAN_POINT('Ctrl Pts',(17.1596890326764,-0.764244139583423,
26.5841780746757));
#44403=CARTESIAN_POINT('Ctrl Pts',(17.1667006141106,-0.764310045233262,
26.4999834783144));
#44404=CARTESIAN_POINT('Origin',(8.83329938588935,0.,26.5));
#44405=CARTESIAN_POINT('',(16.2332993858894,-0.764419552496706,26.4999089030413));
#44406=CARTESIAN_POINT('',(16.3667006141106,-0.764284539029021,26.4999969545263));
#44407=CARTESIAN_POINT('',(8.83329938588935,-0.76435,26.5000000000004));
#44408=CARTESIAN_POINT('Ctrl Pts',(16.2332993858894,-0.764419552496625,
26.4999089030413));
#44409=CARTESIAN_POINT('Ctrl Pts',(16.2345765102041,-0.764440883098184,
26.4845572251809));
#44410=CARTESIAN_POINT('Ctrl Pts',(16.2464391700194,-0.760308610213227,
26.3420005829642));
#44411=CARTESIAN_POINT('Ctrl Pts',(16.2688873653352,-0.675403430232317,
26.0776946475575));
#44412=CARTESIAN_POINT('Ctrl Pts',(16.3006439718369,-0.391057471568795,
25.8055962039035));
#44413=CARTESIAN_POINT('Ctrl Pts',(16.3324005783384,-0.0112469392005812,
25.7034392542279));
#44414=CARTESIAN_POINT('Ctrl Pts',(16.3641571848401,0.371296397184491,25.7948322443979));
#44415=CARTESIAN_POINT('Ctrl Pts',(16.3959137913416,0.663211193852015,26.0587942468411));
#44416=CARTESIAN_POINT('Ctrl Pts',(16.4276703978433,0.79383189911164,26.4291575914007));
#44417=CARTESIAN_POINT('Ctrl Pts',(16.4594270043448,0.730299950020167,26.8187946688532));
#44418=CARTESIAN_POINT('Ctrl Pts',(16.4911836108465,0.490067202099917,27.127082508535));
#44419=CARTESIAN_POINT('Ctrl Pts',(16.5335257528485,0.00755075451268908,
27.3426896078416));
#44420=CARTESIAN_POINT('Ctrl Pts',(16.5758678948507,-0.530671740917147,
27.1546528029804));
#44421=CARTESIAN_POINT('Ctrl Pts',(16.6126542843645,-0.742027902742413,
26.7470388885421));
#44422=CARTESIAN_POINT('Ctrl Pts',(16.6282696028772,-0.764117266668342,
26.5598914421017));
#44423=CARTESIAN_POINT('Ctrl Pts',(16.6332993858894,-0.764172016402596,
26.4996705939536));
#44424=CARTESIAN_POINT('Ctrl Pts',(16.3667006141106,-0.764284539028846,
26.4999969545263));
#44425=CARTESIAN_POINT('Ctrl Pts',(16.3717348297846,-0.764292894067563,
26.4395406561741));
#44426=CARTESIAN_POINT('Ctrl Pts',(16.3873782483568,-0.742275719971854,
26.2516835762977));
#44427=CARTESIAN_POINT('Ctrl Pts',(16.4136308698273,-0.590020482577639,
25.9643030788146));
#44428=CARTESIAN_POINT('Ctrl Pts',(16.4454584785221,-0.261004878818793,
25.7470246919976));
#44429=CARTESIAN_POINT('Ctrl Pts',(16.477286087217,0.131900535795971,25.7140625916236));
#44430=CARTESIAN_POINT('Ctrl Pts',(16.5091136959118,0.492518813396506,25.8734853715362));
#44431=CARTESIAN_POINT('Ctrl Pts',(16.5409413046066,0.732576379744177,26.1862688904977));
#44432=CARTESIAN_POINT('Ctrl Pts',(16.5727689133014,0.793310990324887,26.5758487564716));
#44433=CARTESIAN_POINT('Ctrl Pts',(16.6045965219962,0.659855785944694,26.9468620625921));
#44434=CARTESIAN_POINT('Ctrl Pts',(16.636424130691,0.364878461567863,27.2084906982538));
#44435=CARTESIAN_POINT('Ctrl Pts',(16.6682517393859,-0.0194152617984515,
27.2966921669241));
#44436=CARTESIAN_POINT('Ctrl Pts',(16.7000793480807,-0.398956440272542,
27.1898761627955));
#44437=CARTESIAN_POINT('Ctrl Pts',(16.7319069567755,-0.680839476780989,
26.9141895315969));
#44438=CARTESIAN_POINT('Ctrl Pts',(16.7541140454521,-0.761235069795498,
26.651093842388));
#44439=CARTESIAN_POINT('Ctrl Pts',(16.7657119312305,-0.764409996925297,
26.5118797423986));
#44440=CARTESIAN_POINT('Ctrl Pts',(16.7667006141106,-0.764401227565479,
26.5000117829436));
#44441=CARTESIAN_POINT('Origin',(8.83329938588935,0.,26.5));
#44442=CARTESIAN_POINT('',(15.8332993858894,-0.7642585736457,26.5000568905623));
#44443=CARTESIAN_POINT('',(15.9667006141106,-0.764412740073756,26.4999943266675));
#44444=CARTESIAN_POINT('',(8.83329938588935,-0.76435,26.5000000000004));
#44445=CARTESIAN_POINT('Ctrl Pts',(15.8332993858894,-0.764258573645619,
26.5000568905623));
#44446=CARTESIAN_POINT('Ctrl Pts',(15.8408834175311,-0.764191761169323,
26.4089790323552));
#44447=CARTESIAN_POINT('Ctrl Pts',(15.8590529846733,-0.725349790004131,
26.1906373179569));
#44448=CARTESIAN_POINT('Ctrl Pts',(15.8878080873161,-0.522035840432493,
25.8982408316857));
#44449=CARTESIAN_POINT('Ctrl Pts',(15.9195646938177,-0.17065433029262,25.7215401887988));
#44450=CARTESIAN_POINT('Ctrl Pts',(15.9513213003193,0.222669695330672,25.7351929582878));
#44451=CARTESIAN_POINT('Ctrl Pts',(15.9830779068209,0.561259543601463,25.9341595139798));
#44452=CARTESIAN_POINT('Ctrl Pts',(16.0148345133225,0.763833671200898,26.2730062101543));
#44453=CARTESIAN_POINT('Ctrl Pts',(16.0465911198241,0.778876573811572,26.6635531040737));
#44454=CARTESIAN_POINT('Ctrl Pts',(16.0889332618262,0.548943088162816,27.1394093172736));
#44455=CARTESIAN_POINT('Ctrl Pts',(16.1312754038283,0.016244012154183,27.3425668644846));
#44456=CARTESIAN_POINT('Ctrl Pts',(16.1736175458305,-0.47216734905144,27.1406686581801));
#44457=CARTESIAN_POINT('Ctrl Pts',(16.2040970280173,-0.711000868579955,
26.8514066340567));
#44458=CARTESIAN_POINT('Ctrl Pts',(16.2239909747036,-0.764264082893658,
26.6118006963973));
#44459=CARTESIAN_POINT('Ctrl Pts',(16.2332993858894,-0.764419552496625,
26.4999089030413));
#44460=CARTESIAN_POINT('Ctrl Pts',(15.9667006141106,-0.764412740073581,
26.4999943266675));
#44461=CARTESIAN_POINT('Ctrl Pts',(15.9671485254403,-0.764414872326465,
26.4946179201944));
#44462=CARTESIAN_POINT('Ctrl Pts',(15.9782056396684,-0.763044002953407,
26.3618973388524));
#44463=CARTESIAN_POINT('Ctrl Pts',(15.9998719567947,-0.691172178101171,
26.1032930786494));
#44464=CARTESIAN_POINT('Ctrl Pts',(16.0316995654895,-0.416405297022751,
25.8205134366008));
#44465=CARTESIAN_POINT('Ctrl Pts',(16.0635271741844,-0.0397090735252242,
25.7040612142204));
#44466=CARTESIAN_POINT('Ctrl Pts',(16.0953547828791,0.346707294700135,25.782442049009));
#44467=CARTESIAN_POINT('Ctrl Pts',(16.127182391574,0.648255274330614,26.0364695689265));
#44468=CARTESIAN_POINT('Ctrl Pts',(16.1590100002688,0.791120753270836,26.4039619087403));
#44469=CARTESIAN_POINT('Ctrl Pts',(16.1908376089636,0.740332552174896,26.7949628339619));
#44470=CARTESIAN_POINT('Ctrl Pts',(16.2226652176584,0.508322808619745,27.1137615851986));
#44471=CARTESIAN_POINT('Ctrl Pts',(16.2544928263532,0.151883789093077,27.2823213379676));
#44472=CARTESIAN_POINT('Ctrl Pts',(16.2863204350481,-0.24173394755624,27.2593813665264));
#44473=CARTESIAN_POINT('Ctrl Pts',(16.3181480437429,-0.576179088441399,
27.0505570081939));
#44474=CARTESIAN_POINT('Ctrl Pts',(16.3449414367637,-0.738993578414591,
26.7613115100435));
#44475=CARTESIAN_POINT('Ctrl Pts',(16.3611256268863,-0.764275286498338,
26.5669474216436));
#44476=CARTESIAN_POINT('Ctrl Pts',(16.3667006141106,-0.764284539028846,
26.4999969545263));
#44477=CARTESIAN_POINT('Origin',(8.83329938588935,0.,26.5));
#44478=CARTESIAN_POINT('',(15.4332993858894,-0.764307134319736,26.4999943060657));
#44479=CARTESIAN_POINT('',(15.5667006141106,-0.764296441926655,26.5000122845045));
#44480=CARTESIAN_POINT('',(8.83329938588935,-0.76435,26.5000000000004));
#44481=CARTESIAN_POINT('Ctrl Pts',(15.4332993858894,-0.764307134319656,
26.4999943060657));
#44482=CARTESIAN_POINT('Ctrl Pts',(15.4366047893575,-0.764328149531655,
26.4603037681963));
#44483=CARTESIAN_POINT('Ctrl Pts',(15.4504957283262,-0.751518870125793,
26.2935211503543));
#44484=CARTESIAN_POINT('Ctrl Pts',(15.4749722027953,-0.632243102185288,
26.0148286510498));
#44485=CARTESIAN_POINT('Ctrl Pts',(15.5067288092969,-0.32272804759704,25.7717430319143));
#44486=CARTESIAN_POINT('Ctrl Pts',(15.5384854157985,0.0643873344812935,
25.7056184782728));
#44487=CARTESIAN_POINT('Ctrl Pts',(15.5702420223001,0.43767439511808,25.8341102330364));
#44488=CARTESIAN_POINT('Ctrl Pts',(15.6019986288018,0.700909172129369,26.1230057460524));
#44489=CARTESIAN_POINT('Ctrl Pts',(15.6443407708038,0.831835447076346,26.6350280639177));
#44490=CARTESIAN_POINT('Ctrl Pts',(15.686682912806,0.555510380759211,27.1337120844097));
#44491=CARTESIAN_POINT('Ctrl Pts',(15.7290250548081,0.0519596797800127,
27.2941653019125));
#44492=CARTESIAN_POINT('Ctrl Pts',(15.7607816613097,-0.332552292829113,
27.2241388198563));
#44493=CARTESIAN_POINT('Ctrl Pts',(15.7925382678113,-0.639407707442898,
26.9757578318493));
#44494=CARTESIAN_POINT('Ctrl Pts',(15.8167108426712,-0.752956785112338,
26.6992298118808));
#44495=CARTESIAN_POINT('Ctrl Pts',(15.8302978820306,-0.764285015769663,
26.5361024341171));
#44496=CARTESIAN_POINT('Ctrl Pts',(15.8332993858894,-0.764258573645619,
26.5000568905623));
#44497=CARTESIAN_POINT('Ctrl Pts',(15.5667006141106,-0.764296441926479,
26.5000122845045));
#44498=CARTESIAN_POINT('Ctrl Pts',(15.5731714239944,-0.764252283086693,
26.4223072739739));
#44499=CARTESIAN_POINT('Ctrl Pts',(15.5902514367765,-0.733154199056112,
26.2171666244304));
#44500=CARTESIAN_POINT('Ctrl Pts',(15.6179406524569,-0.552431099026793,
25.9256175124043));
#44501=CARTESIAN_POINT('Ctrl Pts',(15.6497682611517,-0.209471088532158,
25.7310934879338));
#44502=CARTESIAN_POINT('Ctrl Pts',(15.6815958698465,0.184764086958111,25.7247854533105));
#44503=CARTESIAN_POINT('Ctrl Pts',(15.7134234785413,0.533771975425466,25.9082375143023));
#44504=CARTESIAN_POINT('Ctrl Pts',(15.7452510872362,0.752121039795552,26.2365435468138));
#44505=CARTESIAN_POINT('Ctrl Pts',(15.7770786959309,0.78636292888696,26.6293394962914));
#44506=CARTESIAN_POINT('Ctrl Pts',(15.8089063046258,0.628115777091278,26.9904752101765));
#44507=CARTESIAN_POINT('Ctrl Pts',(15.8407339133206,0.316115950726511,27.2315504541211));
#44508=CARTESIAN_POINT('Ctrl Pts',(15.8725615220154,-0.073263993557323,
27.2935538724477));
#44509=CARTESIAN_POINT('Ctrl Pts',(15.9043891307102,-0.444710086519647,
27.1613080221623));
#44510=CARTESIAN_POINT('Ctrl Pts',(15.9357688280753,-0.703602863161262,
26.8713237799752));
#44511=CARTESIAN_POINT('Ctrl Pts',(15.9565393225421,-0.764364367902979,
26.6219631855317));
#44512=CARTESIAN_POINT('Ctrl Pts',(15.9667006141106,-0.764412740073581,
26.4999943266675));
#44513=CARTESIAN_POINT('Origin',(8.83329938588935,0.,26.5));
#44514=CARTESIAN_POINT('',(15.0332993858894,-0.764434241529034,26.5000259538096));
#44515=CARTESIAN_POINT('',(15.1667006141106,-0.764371352146507,26.4999814664004));
#44516=CARTESIAN_POINT('',(8.83329938588935,-0.76435,26.5000000000004));
#44517=CARTESIAN_POINT('Ctrl Pts',(15.0332993858894,-0.764434241528954,
26.5000259538096));
#44518=CARTESIAN_POINT('Ctrl Pts',(15.0429116966845,-0.764309333684609,
26.3846361440151));
#44519=CARTESIAN_POINT('Ctrl Pts',(15.0631095429801,-0.708387433195622,
26.1420365804305));
#44520=CARTESIAN_POINT('Ctrl Pts',(15.0938929247762,-0.462805184149422,
25.8511555714751));
#44521=CARTESIAN_POINT('Ctrl Pts',(15.1256495312778,-0.0945878860313145,
25.7087849914816));
#44522=CARTESIAN_POINT('Ctrl Pts',(15.1574061377794,0.292880226372572,25.7599868189792));
#44523=CARTESIAN_POINT('Ctrl Pts',(15.1997482797815,0.723012441153252,26.067061437389));
#44524=CARTESIAN_POINT('Ctrl Pts',(15.2420904217837,0.833184204547314,26.6264391962602));
#44525=CARTESIAN_POINT('Ctrl Pts',(15.2844325637858,0.551618642248873,27.0736856356996));
#44526=CARTESIAN_POINT('Ctrl Pts',(15.3161891702874,0.21250416882743,27.2679909088782));
#44527=CARTESIAN_POINT('Ctrl Pts',(15.347945776789,-0.182199657223414,27.2758808000015));
#44528=CARTESIAN_POINT('Ctrl Pts',(15.3797023832906,-0.530413882922957,
27.0942833642916));
#44529=CARTESIAN_POINT('Ctrl Pts',(15.408153586324,-0.727612087344244,26.8019865156775));
#44530=CARTESIAN_POINT('Ctrl Pts',(15.426019253857,-0.7642608484367,26.587412486301));
#44531=CARTESIAN_POINT('Ctrl Pts',(15.4332993858894,-0.764307134319656,
26.4999943060657));
#44532=CARTESIAN_POINT('Ctrl Pts',(15.1667006141106,-0.764371352146331,
26.4999814664004));
#44533=CARTESIAN_POINT('Ctrl Pts',(15.1685851196502,-0.764394352807559,
26.4773576674607));
#44534=CARTESIAN_POINT('Ctrl Pts',(15.1810788280881,-0.757868527003245,
26.3273818655522));
#44535=CARTESIAN_POINT('Ctrl Pts',(15.2041817394243,-0.6627532402055,26.0574466090676));
#44536=CARTESIAN_POINT('Ctrl Pts',(15.2360093481191,-0.369486777125133,
25.7939016479567));
#44537=CARTESIAN_POINT('Ctrl Pts',(15.2678369568139,0.0142241267301174,
25.7031982458306));
#44538=CARTESIAN_POINT('Ctrl Pts',(15.2996645655087,0.394453192351198,25.8075391417037));
#44539=CARTESIAN_POINT('Ctrl Pts',(15.3314921742035,0.678126438920626,26.0813833566788));
#44540=CARTESIAN_POINT('Ctrl Pts',(15.3633197828983,0.795805202493795,26.4576982162029));
#44541=CARTESIAN_POINT('Ctrl Pts',(15.3951473915932,0.718683607945039,26.8443678743723));
#44542=CARTESIAN_POINT('Ctrl Pts',(15.426975000288,0.465639785487568,27.1467417965461));
#44543=CARTESIAN_POINT('Ctrl Pts',(15.4588026089828,0.0986148069826778,
27.2908036931327));
#44544=CARTESIAN_POINT('Ctrl Pts',(15.4906302176776,-0.292549495638406,
27.2412895209231));
#44545=CARTESIAN_POINT('Ctrl Pts',(15.5224578263724,-0.612102370814474,
27.0103195556432));
#44546=CARTESIAN_POINT('Ctrl Pts',(15.5478146251834,-0.747316944725573,
26.7267864498628));
#44547=CARTESIAN_POINT('Ctrl Pts',(15.5625622210961,-0.7643246836207,26.5497083625134));
#44548=CARTESIAN_POINT('Ctrl Pts',(15.5667006141106,-0.764296441926479,
26.5000122845045));
#44549=CARTESIAN_POINT('Origin',(8.83329938588935,0.,26.5));
#44550=CARTESIAN_POINT('',(14.6332993858894,-0.764344384160412,26.5000700212582));
#44551=CARTESIAN_POINT('',(14.7667006141106,-0.764340249516096,26.5000200137165));
#44552=CARTESIAN_POINT('',(8.83329938588935,-0.76435,26.5000000000004));
#44553=CARTESIAN_POINT('Ctrl Pts',(14.6332993858894,-0.764344384160332,
26.5000700212582));
#44554=CARTESIAN_POINT('Ctrl Pts',(14.6386330685109,-0.764379701483647,
26.43606499794));
#44555=CARTESIAN_POINT('Ctrl Pts',(14.6545522866329,-0.740679592119133,
26.2449843755321));
#44556=CARTESIAN_POINT('Ctrl Pts',(14.6810570402554,-0.582308270804313,
25.9560467523384));
#44557=CARTESIAN_POINT('Ctrl Pts',(14.712813646757,-0.25306744493287,25.7454437042873));
#44558=CARTESIAN_POINT('Ctrl Pts',(14.7551557887592,0.273719354082281,25.7029676893257));
#44559=CARTESIAN_POINT('Ctrl Pts',(14.7974979307613,0.718507527034393,26.059625474564));
#44560=CARTESIAN_POINT('Ctrl Pts',(14.8398400727634,0.791517698526367,26.5830546085662));
#44561=CARTESIAN_POINT('Ctrl Pts',(14.871596679265,0.657491382035733,26.9501923371599));
#44562=CARTESIAN_POINT('Ctrl Pts',(14.9033532857666,0.360807099282544,27.2106377192428));
#44563=CARTESIAN_POINT('Ctrl Pts',(14.9351098922682,-0.0224710100972664,
27.2962453503641));
#44564=CARTESIAN_POINT('Ctrl Pts',(14.9668664987698,-0.401047778060038,
27.1886822618713));
#44565=CARTESIAN_POINT('Ctrl Pts',(14.9986231052714,-0.681355176354821,
26.912784010108));
#44566=CARTESIAN_POINT('Ctrl Pts',(15.0207674009779,-0.761372084745381,
26.6504566973273));
#44567=CARTESIAN_POINT('Ctrl Pts',(15.0323261611839,-0.764446888165399,
26.5117089108056));
#44568=CARTESIAN_POINT('Ctrl Pts',(15.0332993858894,-0.764434241528954,
26.5000259538096));
#44569=CARTESIAN_POINT('Ctrl Pts',(14.7667006141106,-0.764340249515921,
26.5000200137165));
#44570=CARTESIAN_POINT('Ctrl Pts',(14.7746080182043,-0.764244504017631,
26.4050792053235));
#44571=CARTESIAN_POINT('Ctrl Pts',(14.7931246251962,-0.722720395989046,
26.1826768460789));
#44572=CARTESIAN_POINT('Ctrl Pts',(14.8222504350865,-0.512310886867079,
25.8895633395461));
#44573=CARTESIAN_POINT('Ctrl Pts',(14.8540780437813,-0.156977657442333,
25.71868484189));
#44574=CARTESIAN_POINT('Ctrl Pts',(14.8859056524761,0.236781186430625,25.7390597717421));
#44575=CARTESIAN_POINT('Ctrl Pts',(14.9177332611709,0.572579791078355,25.9457006728515));
#44576=CARTESIAN_POINT('Ctrl Pts',(14.9495608698657,0.768220040382449,26.2880251647402));
#44577=CARTESIAN_POINT('Ctrl Pts',(14.9813884785605,0.775812337104691,26.6822376986926));
#44578=CARTESIAN_POINT('Ctrl Pts',(15.0132160872554,0.593498208699499,27.0318413649756));
#44579=CARTESIAN_POINT('Ctrl Pts',(15.0450436959502,0.265905231604842,27.2512587896549));
#44580=CARTESIAN_POINT('Ctrl Pts',(15.076871304645,-0.126777084163142,27.2867801040696));
#44581=CARTESIAN_POINT('Ctrl Pts',(15.1086989133398,-0.488426401756141,
27.129710259799));
#44582=CARTESIAN_POINT('Ctrl Pts',(15.138642016495,-0.716182649017405,26.8369242782581));
#44583=CARTESIAN_POINT('Ctrl Pts',(15.1579759167519,-0.764264865959882,
26.6047228931048));
#44584=CARTESIAN_POINT('Ctrl Pts',(15.1667006141106,-0.764371352146331,
26.4999814664004));
#44585=CARTESIAN_POINT('Origin',(8.83329938588935,0.,26.5));
#44586=CARTESIAN_POINT('',(14.2332993858894,-0.764405081589298,26.4996880256457));
#44587=CARTESIAN_POINT('',(14.3667006141106,-0.764318529753706,26.4999818788456));
#44588=CARTESIAN_POINT('',(8.83329938588935,-0.76435,26.5000000000004));
#44589=CARTESIAN_POINT('Ctrl Pts',(14.2332993858894,-0.764405081589217,
26.4996880256457));
#44590=CARTESIAN_POINT('Ctrl Pts',(14.2343544403373,-0.764414798326942,
26.4870305763771));
#44591=CARTESIAN_POINT('Ctrl Pts',(14.2459950302857,-0.761012346251615,
26.3474474462872));
#44592=CARTESIAN_POINT('Ctrl Pts',(14.2682211557347,-0.679844423442565,
26.0862248255409));
#44593=CARTESIAN_POINT('Ctrl Pts',(14.3105632977368,-0.304469510421639,
25.714200339602));
#44594=CARTESIAN_POINT('Ctrl Pts',(14.352905439739,0.26548215438068,25.7001862624564));
#44595=CARTESIAN_POINT('Ctrl Pts',(14.3952475817411,0.658687214192637,26.0533127616064));
#44596=CARTESIAN_POINT('Ctrl Pts',(14.4270041882427,0.79286270006155,26.4203960004784));
#44597=CARTESIAN_POINT('Ctrl Pts',(14.4587607947443,0.73390803483815,26.8107518741751));
#44598=CARTESIAN_POINT('Ctrl Pts',(14.4905174012459,0.496053570864849,27.1232515215411));
#44599=CARTESIAN_POINT('Ctrl Pts',(14.5222740077474,0.137281974103891,27.2850326347925));
#44600=CARTESIAN_POINT('Ctrl Pts',(14.5540306142491,-0.254861359535286,
27.2547722853697));
#44601=CARTESIAN_POINT('Ctrl Pts',(14.5857872207506,-0.58507796496343,27.0411158406638));
#44602=CARTESIAN_POINT('Ctrl Pts',(14.6122101446308,-0.740884937302533,
26.7530976530099));
#44603=CARTESIAN_POINT('Ctrl Pts',(14.6280475330103,-0.764309608677931,
26.5630930749048));
#44604=CARTESIAN_POINT('Ctrl Pts',(14.6332993858894,-0.764344384160332,
26.5000700212582));
#44605=CARTESIAN_POINT('Ctrl Pts',(14.3667006141106,-0.76431852975353,26.4999818788456));
#44606=CARTESIAN_POINT('Ctrl Pts',(14.3700217138601,-0.764353313265897,
26.4601036057722));
#44607=CARTESIAN_POINT('Ctrl Pts',(14.3839520165078,-0.751491973744368,
26.292857013788));
#44608=CARTESIAN_POINT('Ctrl Pts',(14.4084915220538,-0.631298059665474,
26.0136275901214));
#44609=CARTESIAN_POINT('Ctrl Pts',(14.4403191307486,-0.3208755434976,25.7705246770357));
#44610=CARTESIAN_POINT('Ctrl Pts',(14.4721467394435,0.0680921626112602,
25.7059856307223));
#44611=CARTESIAN_POINT('Ctrl Pts',(14.5039743481383,0.440391998718261,25.8358085752634));
#44612=CARTESIAN_POINT('Ctrl Pts',(14.5358019568331,0.704890932298469,26.128214934684));
#44613=CARTESIAN_POINT('Ctrl Pts',(14.5676295655279,0.79684386389434,26.5116283189908));
#44614=CARTESIAN_POINT('Ctrl Pts',(14.5994571742227,0.693742189705464,26.8921952771914));
#44615=CARTESIAN_POINT('Ctrl Pts',(14.6312847829175,0.42082354702301,27.1767591177809));
#44616=CARTESIAN_POINT('Ctrl Pts',(14.6631123916124,0.0448940451386551,
27.2956631736732));
#44617=CARTESIAN_POINT('Ctrl Pts',(14.6949400003072,-0.342024799417935,
27.2198016378223));
#44618=CARTESIAN_POINT('Ctrl Pts',(14.726767609002,-0.645221455172022,26.967744198269));
#44619=CARTESIAN_POINT('Ctrl Pts',(14.7506878136031,-0.754389946559197,
26.6922588448303));
#44620=CARTESIAN_POINT('Ctrl Pts',(14.763998815306,-0.764372963801135,26.5324593527946));
#44621=CARTESIAN_POINT('Ctrl Pts',(14.7667006141106,-0.764340249515921,
26.5000200137165));
#44622=CARTESIAN_POINT('Origin',(8.83329938588935,0.,26.5));
#44623=CARTESIAN_POINT('',(13.8332993858894,-0.764305323848687,26.5000357755724));
#44624=CARTESIAN_POINT('',(13.9667006141106,-0.764393063012862,26.5000143835574));
#44625=CARTESIAN_POINT('',(8.83329938588935,-0.76435,26.5000000000004));
#44626=CARTESIAN_POINT('Ctrl Pts',(13.8332993858894,-0.764305323848606,
26.5000357755724));
#44627=CARTESIAN_POINT('Ctrl Pts',(13.8406613476642,-0.764560699159756,
26.4112555362681));
#44628=CARTESIAN_POINT('Ctrl Pts',(13.8691943804402,-0.706795172742057,
26.0666855489971));
#44629=CARTESIAN_POINT('Ctrl Pts',(13.9083129487166,-0.3125600582338,25.7173832361526));
#44630=CARTESIAN_POINT('Ctrl Pts',(13.9506550907188,0.21567771148749,25.7339181115233));
#44631=CARTESIAN_POINT('Ctrl Pts',(13.9824116972203,0.554871109700202,25.9280855750125));
#44632=CARTESIAN_POINT('Ctrl Pts',(14.0141683037219,0.761408101094941,26.2645314575356));
#44633=CARTESIAN_POINT('Ctrl Pts',(14.0459249102235,0.780984108470458,26.6567655146636));
#44634=CARTESIAN_POINT('Ctrl Pts',(14.0776815167251,0.610964975807012,27.0117073152108));
#44635=CARTESIAN_POINT('Ctrl Pts',(14.1094381232267,0.291647913206453,27.241334614104));
#44636=CARTESIAN_POINT('Ctrl Pts',(14.1411947297283,-0.0985343487612529,
27.2908309302356));
#44637=CARTESIAN_POINT('Ctrl Pts',(14.1729513362299,-0.464823397167573,
27.1468777424806));
#44638=CARTESIAN_POINT('Ctrl Pts',(14.2036528882836,-0.70934576818595,26.8564267856704));
#44639=CARTESIAN_POINT('Ctrl Pts',(14.2237689048368,-0.764317308692789,
26.6140248550565));
#44640=CARTESIAN_POINT('Ctrl Pts',(14.2332993858894,-0.764405081589217,
26.4996880256457));
#44641=CARTESIAN_POINT('Ctrl Pts',(13.9667006141106,-0.764393063012687,
26.5000143835574));
#44642=CARTESIAN_POINT('Ctrl Pts',(13.9760446124141,-0.764296506000937,
26.3878473518458));
#44643=CARTESIAN_POINT('Ctrl Pts',(13.9959978136159,-0.710931609772101,
26.1482367165881));
#44644=CARTESIAN_POINT('Ctrl Pts',(14.026560217716,-0.469843647084554,25.856305733657));
#44645=CARTESIAN_POINT('Ctrl Pts',(14.0583878264108,-0.10376507142601,25.7098556010573));
#44646=CARTESIAN_POINT('Ctrl Pts',(14.0902154351057,0.287713530534183,25.7568201526036));
#44647=CARTESIAN_POINT('Ctrl Pts',(14.1220430438004,0.608764471794302,25.9857032188419));
#44648=CARTESIAN_POINT('Ctrl Pts',(14.1538706524953,0.780799627852441,26.3404778937761));
#44649=CARTESIAN_POINT('Ctrl Pts',(14.1856982611901,0.761707549946172,26.734301023437));
#44650=CARTESIAN_POINT('Ctrl Pts',(14.2175258698849,0.556161672732346,27.0707710180205));
#44651=CARTESIAN_POINT('Ctrl Pts',(14.2493534785797,0.214476332390549,27.2675254159133));
#44652=CARTESIAN_POINT('Ctrl Pts',(14.2811810872745,-0.17970937641759,27.2764018941606));
#44653=CARTESIAN_POINT('Ctrl Pts',(14.3130086959694,-0.529905110324446,
27.0952276331628));
#44654=CARTESIAN_POINT('Ctrl Pts',(14.3415152049147,-0.727381888508666,
26.8024596028993));
#44655=CARTESIAN_POINT('Ctrl Pts',(14.3594125109618,-0.76424219786195,26.5874941457083));
#44656=CARTESIAN_POINT('Ctrl Pts',(14.3667006141106,-0.76431852975353,26.4999818788456));
#44657=CARTESIAN_POINT('Origin',(8.83329938588935,0.,26.5));
#44658=CARTESIAN_POINT('',(13.4332993858894,-0.763192368143962,26.5001425072106));
#44659=CARTESIAN_POINT('',(13.5667006141106,-0.764286670935071,26.4999939108431));
#44660=CARTESIAN_POINT('',(8.83329938588935,-0.76435,26.5000000000004));
#44661=CARTESIAN_POINT('Ctrl Pts',(13.4332993858894,-0.763192368143881,
26.5001425072106));
#44662=CARTESIAN_POINT('Ctrl Pts',(13.4469682549912,-0.762179560466138,
26.3361944380773));
#44663=CARTESIAN_POINT('Ctrl Pts',(13.4712226595935,-0.669971224498844,
26.0450308521942));
#44664=CARTESIAN_POINT('Ctrl Pts',(13.5060625996964,-0.328895476366436,
25.7752751551725));
#44665=CARTESIAN_POINT('Ctrl Pts',(13.537819206198,0.0555880103782207,25.7050924387132));
#44666=CARTESIAN_POINT('Ctrl Pts',(13.5695758126996,0.430357382868759,25.8291943247753));
#44667=CARTESIAN_POINT('Ctrl Pts',(13.6013324192012,0.698145424343159,26.1164578631495));
#44668=CARTESIAN_POINT('Ctrl Pts',(13.6330890257028,0.796941593703338,26.497416527793));
#44669=CARTESIAN_POINT('Ctrl Pts',(13.6648456322043,0.700818762673457,26.8787988611799));
#44670=CARTESIAN_POINT('Ctrl Pts',(13.696602238706,0.434409572344521,27.1681398817303));
#44671=CARTESIAN_POINT('Ctrl Pts',(13.7283588452075,0.0615766530934091,
27.2941787708476));
#44672=CARTESIAN_POINT('Ctrl Pts',(13.7601154517091,-0.325445621555236,
27.2275114283046));
#44673=CARTESIAN_POINT('Ctrl Pts',(13.7918720582108,-0.634571402982474,
26.9819618163357));
#44674=CARTESIAN_POINT('Ctrl Pts',(13.8162667029375,-0.751263355401409,
26.7053363730211));
#44675=CARTESIAN_POINT('Ctrl Pts',(13.8300758121637,-0.764193502955155,
26.5389098767338));
#44676=CARTESIAN_POINT('Ctrl Pts',(13.8332993858894,-0.764305323848606,
26.5000357755724));
#44677=CARTESIAN_POINT('Ctrl Pts',(13.5667006141106,-0.764286670934895,
26.4999939108431));
#44678=CARTESIAN_POINT('Ctrl Pts',(13.5714583080699,-0.764302511396769,
26.4428588396704));
#44679=CARTESIAN_POINT('Ctrl Pts',(13.5868252049275,-0.743884224407635,
26.2583291650472));
#44680=CARTESIAN_POINT('Ctrl Pts',(13.6128013046834,-0.59695074073402,25.9720367679793));
#44681=CARTESIAN_POINT('Ctrl Pts',(13.6446289133782,-0.270794296674234,
25.7504896197401));
#44682=CARTESIAN_POINT('Ctrl Pts',(13.676456522073,0.121648250824199,25.7124105991698));
#44683=CARTESIAN_POINT('Ctrl Pts',(13.7082841307678,0.484313256342262,25.86712084016));
#44684=CARTESIAN_POINT('Ctrl Pts',(13.7401117394627,0.728426139452693,26.176749755467));
#44685=CARTESIAN_POINT('Ctrl Pts',(13.7719393481575,0.794231979098091,26.5655051494659));
#44686=CARTESIAN_POINT('Ctrl Pts',(13.8037669568523,0.665622560492644,26.9382259328153));
#44687=CARTESIAN_POINT('Ctrl Pts',(13.8355945655471,0.374079407913512,27.2036760318525));
#44688=CARTESIAN_POINT('Ctrl Pts',(13.8674221742419,-0.00903238784518047,
27.2968775170617));
#44689=CARTESIAN_POINT('Ctrl Pts',(13.8992497829368,-0.389933199833693,
27.1950161587302));
#44690=CARTESIAN_POINT('Ctrl Pts',(13.9310773916315,-0.675384614490799,
26.9230259847075));
#44691=CARTESIAN_POINT('Ctrl Pts',(13.9535610020228,-0.760245312512092,
26.6577374861337));
#44692=CARTESIAN_POINT('Ctrl Pts',(13.9654354095158,-0.764406137113403,
26.5152021264581));
#44693=CARTESIAN_POINT('Ctrl Pts',(13.9667006141106,-0.764393063012687,
26.5000143835574));
#44694=CARTESIAN_POINT('Origin',(8.83329938588935,0.,26.5));
#44695=CARTESIAN_POINT('',(13.0332993858894,-0.765185328759249,26.5005140269729));
#44696=CARTESIAN_POINT('',(13.1667006141106,-0.76441561830137,26.4999977981034));
#44697=CARTESIAN_POINT('',(8.83329938588935,-0.76435,26.5000000000004));
#44698=CARTESIAN_POINT('Ctrl Pts',(13.0332993858894,-0.765185328759169,
26.5005140269729));
#44699=CARTESIAN_POINT('Ctrl Pts',(13.0426896268176,-0.765069612564117,
26.3877758463834));
#44700=CARTESIAN_POINT('Ctrl Pts',(13.0626654032463,-0.709228609067927,
26.1465610485235));
#44701=CARTESIAN_POINT('Ctrl Pts',(13.0932267151756,-0.469871753862732,
25.8564251459149));
#44702=CARTESIAN_POINT('Ctrl Pts',(13.1249833216772,-0.103350723706369,
25.7097428527291));
#44703=CARTESIAN_POINT('Ctrl Pts',(13.1567399281788,0.286546658439126,25.7567620725444));
#44704=CARTESIAN_POINT('Ctrl Pts',(13.1884965346804,0.607634532323689,25.9843423100245));
#44705=CARTESIAN_POINT('Ctrl Pts',(13.220253141182,0.779970642319146,26.3378848789699));
#44706=CARTESIAN_POINT('Ctrl Pts',(13.2520097476836,0.762787909334418,26.7308185076554));
#44707=CARTESIAN_POINT('Ctrl Pts',(13.2837663541852,0.558979957403396,27.0674971466822));
#44708=CARTESIAN_POINT('Ctrl Pts',(13.3155229606868,0.220111430206846,27.265988700436));
#44709=CARTESIAN_POINT('Ctrl Pts',(13.3472795671884,-0.17450318681229,27.2775067174508));
#44710=CARTESIAN_POINT('Ctrl Pts',(13.37903617369,-0.522757319830727,27.1001025909359));
#44711=CARTESIAN_POINT('Ctrl Pts',(13.4077094465903,-0.728082495975273,
26.8069728435505));
#44712=CARTESIAN_POINT('Ctrl Pts',(13.4257971839901,-0.763748250830808,
26.5901259218205));
#44713=CARTESIAN_POINT('Ctrl Pts',(13.4332993858894,-0.763192368143881,
26.5001425072106));
#44714=CARTESIAN_POINT('Ctrl Pts',(13.1667006141106,-0.764415618301195,
26.4999977981034));
#44715=CARTESIAN_POINT('Ctrl Pts',(13.1668720037257,-0.764415956632992,
26.4979405825976));
#44716=CARTESIAN_POINT('Ctrl Pts',(13.1776525962391,-0.76390455814698,26.3685396669369));
#44717=CARTESIAN_POINT('Ctrl Pts',(13.1990423916508,-0.696282751850487,
26.1123330157156));
#44718=CARTESIAN_POINT('Ctrl Pts',(13.2308700003456,-0.425223933001015,
25.8259970563627));
#44719=CARTESIAN_POINT('Ctrl Pts',(13.2626976090404,-0.0500771109931841,
25.7046462144535));
#44720=CARTESIAN_POINT('Ctrl Pts',(13.2945252177352,0.337327785132049,25.777985231033));
#44721=CARTESIAN_POINT('Ctrl Pts',(13.32635282643,0.64216024626656,26.0280618903463));
#44722=CARTESIAN_POINT('Ctrl Pts',(13.3581804351249,0.789802171887619,26.3936614345112));
#44723=CARTESIAN_POINT('Ctrl Pts',(13.3900080438197,0.744113185060425,26.7852909550754));
#44724=CARTESIAN_POINT('Ctrl Pts',(13.4218356525145,0.516277217440969,27.107085822582));
#44725=CARTESIAN_POINT('Ctrl Pts',(13.4536632612093,0.162064862066652,27.2802758113077));
#44726=CARTESIAN_POINT('Ctrl Pts',(13.4854908699041,-0.231818373908386,
27.2624667879633));
#44727=CARTESIAN_POINT('Ctrl Pts',(13.5173184785989,-0.568956187617919,
27.058018116014));
#44728=CARTESIAN_POINT('Ctrl Pts',(13.5443883933344,-0.737244927422413,
26.7679556994413));
#44729=CARTESIAN_POINT('Ctrl Pts',(13.5608491051716,-0.764267188680458,
26.5702645887285));
#44730=CARTESIAN_POINT('Ctrl Pts',(13.5667006141106,-0.764286670934895,
26.4999939108431));
#44731=CARTESIAN_POINT('Origin',(8.83329938588935,0.,26.5));
#44732=CARTESIAN_POINT('',(12.6332993858894,-0.764194707759887,26.4997132521735));
#44733=CARTESIAN_POINT('',(12.7667006141106,-0.764291254740594,26.5000096562347));
#44734=CARTESIAN_POINT('',(8.83329938588935,-0.76435,26.5000000000004));
#44735=CARTESIAN_POINT('Ctrl Pts',(12.6332993858894,-0.764194707759806,
26.4997132521735));
#44736=CARTESIAN_POINT('Ctrl Pts',(12.638410998644,-0.764263423596555,26.4385236355121));
#44737=CARTESIAN_POINT('Ctrl Pts',(12.6541081468992,-0.742061408822202,
26.2507674744643));
#44738=CARTESIAN_POINT('Ctrl Pts',(12.6803908306549,-0.588390470950266,
25.9624273215664));
#44739=CARTESIAN_POINT('Ctrl Pts',(12.7121474371564,-0.259988325015747,
25.7470606431281));
#44740=CARTESIAN_POINT('Ctrl Pts',(12.7439040436581,0.132189409199892,25.7140938108156));
#44741=CARTESIAN_POINT('Ctrl Pts',(12.7756606501597,0.491830546380316,25.8733116970985));
#44742=CARTESIAN_POINT('Ctrl Pts',(12.8074172566613,0.731965703418775,26.1848035737485));
#44743=CARTESIAN_POINT('Ctrl Pts',(12.8391738631629,0.793156876350488,26.5735783512257));
#44744=CARTESIAN_POINT('Ctrl Pts',(12.8709304696645,0.662016937073565,26.9437581615374));
#44745=CARTESIAN_POINT('Ctrl Pts',(12.902687076166,0.367739430229575,27.2069199172065));
#44746=CARTESIAN_POINT('Ctrl Pts',(12.9344436826677,-0.0128663201484088,
27.2957592556109));
#44747=CARTESIAN_POINT('Ctrl Pts',(12.9767858246698,-0.523694256138937,
27.1602477679971));
#44748=CARTESIAN_POINT('Ctrl Pts',(13.0097377257437,-0.757552044794858,
26.7831948742396));
#44749=CARTESIAN_POINT('Ctrl Pts',(13.0321040913171,-0.765200058406782,
26.5148645996986));
#44750=CARTESIAN_POINT('Ctrl Pts',(13.0332993858894,-0.765185328759169,
26.5005140269729));
#44751=CARTESIAN_POINT('Ctrl Pts',(12.7667006141106,-0.764291254740419,
26.5000096562347));
#44752=CARTESIAN_POINT('Ctrl Pts',(12.7728949022798,-0.764258309262706,
26.4256238242962));
#44753=CARTESIAN_POINT('Ctrl Pts',(12.7896983933472,-0.735010668826852,
26.2238090757755));
#44754=CARTESIAN_POINT('Ctrl Pts',(12.817111087313,-0.559868637292059,25.9328646808695));
#44755=CARTESIAN_POINT('Ctrl Pts',(12.8489386960078,-0.219472471696671,
25.7338882618077));
#44756=CARTESIAN_POINT('Ctrl Pts',(12.8807663047026,0.174647037187299,25.7224437167444));
#44757=CARTESIAN_POINT('Ctrl Pts',(12.9125939133974,0.526015750672588,25.9013324868735));
#44758=CARTESIAN_POINT('Ctrl Pts',(12.9444215220922,0.748624239560586,26.2267654685606));
#44759=CARTESIAN_POINT('Ctrl Pts',(12.976249130787,0.787981513819465,26.6190818840437));
#44760=CARTESIAN_POINT('Ctrl Pts',(13.0080767394819,0.634453543543031,26.9822489629997));
#44761=CARTESIAN_POINT('Ctrl Pts',(13.0399043481767,0.325621515054088,27.2273692254711));
#44762=CARTESIAN_POINT('Ctrl Pts',(13.0717319568715,-0.0629174411427496,
27.2944411600796));
#44763=CARTESIAN_POINT('Ctrl Pts',(13.1035595655663,-0.436055216210945,
27.1670466322858));
#44764=CARTESIAN_POINT('Ctrl Pts',(13.135215784646,-0.701019125182456,26.8779350566227));
#44765=CARTESIAN_POINT('Ctrl Pts',(13.1562628008274,-0.764395013528092,
26.6252844516571));
#44766=CARTESIAN_POINT('Ctrl Pts',(13.1667006141106,-0.764415618301195,
26.4999977981034));
#44767=CARTESIAN_POINT('Origin',(8.83329938588935,0.,26.5));
#44768=CARTESIAN_POINT('',(12.2332993858894,-0.76444205887302,26.49989355797));
#44769=CARTESIAN_POINT('',(12.3667006141106,-0.764381481730865,26.4999830130677));
#44770=CARTESIAN_POINT('',(8.83329938588935,-0.76435,26.5000000000004));
#44771=CARTESIAN_POINT('Ctrl Pts',(12.2332993858894,-0.764442058872939,
26.49989355797));
#44772=CARTESIAN_POINT('Ctrl Pts',(12.2341323704704,-0.764453514406101,
26.4898829023171));
#44773=CARTESIAN_POINT('Ctrl Pts',(12.245550890552,-0.76187866258566,26.3526836449442));
#44774=CARTESIAN_POINT('Ctrl Pts',(12.2675549461341,-0.684093539524432,
26.0919220252794));
#44775=CARTESIAN_POINT('Ctrl Pts',(12.2993115526357,-0.405504350759794,
25.8139323651287));
#44776=CARTESIAN_POINT('Ctrl Pts',(12.3310681591373,-0.0279149501101425,
25.7038490903687));
#44777=CARTESIAN_POINT('Ctrl Pts',(12.3628247656389,0.356457281532983,25.7872161726406));
#44778=CARTESIAN_POINT('Ctrl Pts',(12.3945813721405,0.653832357862692,26.0450111516939));
#44779=CARTESIAN_POINT('Ctrl Pts',(12.4263379786421,0.792175442841407,26.4125597423245));
#44780=CARTESIAN_POINT('Ctrl Pts',(12.4580945851437,0.736811757902941,26.8034410837456));
#44781=CARTESIAN_POINT('Ctrl Pts',(12.4898511916453,0.503083492378146,27.1166890097782));
#44782=CARTESIAN_POINT('Ctrl Pts',(12.5321933336474,0.0251849627174119,
27.3423470227353));
#44783=CARTESIAN_POINT('Ctrl Pts',(12.5745354756495,-0.516854899684397,
27.16561535569));
#44784=CARTESIAN_POINT('Ctrl Pts',(12.6117660048971,-0.739349580332478,
26.7576471542168));
#44785=CARTESIAN_POINT('Ctrl Pts',(12.6278254631435,-0.764121121359616,
26.5652399754475));
#44786=CARTESIAN_POINT('Ctrl Pts',(12.6332993858894,-0.764194707759806,
26.4997132521735));
#44787=CARTESIAN_POINT('Ctrl Pts',(12.3667006141106,-0.764381481730689,
26.4999830130677));
#44788=CARTESIAN_POINT('Ctrl Pts',(12.3683085979355,-0.764400131171695,
26.4806796412007));
#44789=CARTESIAN_POINT('Ctrl Pts',(12.3805257846588,-0.758957218875831,
26.334026408485));
#44790=CARTESIAN_POINT('Ctrl Pts',(12.4033521742804,-0.668463625002977,
26.0661201280579));
#44791=CARTESIAN_POINT('Ctrl Pts',(12.4351797829751,-0.378656158975322,
25.7987761594907));
#44792=CARTESIAN_POINT('Ctrl Pts',(12.46700739167,0.00384026553403038,25.7030805476152));
#44793=CARTESIAN_POINT('Ctrl Pts',(12.4988350003648,0.385396654593795,25.8024580443755));
#44794=CARTESIAN_POINT('Ctrl Pts',(12.5306626090596,0.672614119883514,26.0725826314222));
#44795=CARTESIAN_POINT('Ctrl Pts',(12.5624902177544,0.79518642952386,26.4473321394994));
#44796=CARTESIAN_POINT('Ctrl Pts',(12.5943178264493,0.723109846747402,26.8349738956479));
#44797=CARTESIAN_POINT('Ctrl Pts',(12.626145435144,0.474027563748743,27.1406194112225));
#44798=CARTESIAN_POINT('Ctrl Pts',(12.6579730438389,0.108910931026614,27.2894515630053));
#44799=CARTESIAN_POINT('Ctrl Pts',(12.6898006525337,-0.282865351947728,
27.2450386257746));
#44800=CARTESIAN_POINT('Ctrl Pts',(12.7216282612285,-0.605400730631636,
27.0182521746981));
#44801=CARTESIAN_POINT('Ctrl Pts',(12.7472615817541,-0.745813088274415,
26.7334325248592));
#44802=CARTESIAN_POINT('Ctrl Pts',(12.7622856993815,-0.764314736288392,
26.5530273874235));
#44803=CARTESIAN_POINT('Ctrl Pts',(12.7667006141106,-0.764291254740419,
26.5000096562347));
#44804=CARTESIAN_POINT('Origin',(8.83329938588935,0.,26.5));
#44805=CARTESIAN_POINT('',(11.8332993858894,-0.764247147692772,26.500050461596));
#44806=CARTESIAN_POINT('',(11.9667006141106,-0.764330172794767,26.5000194733099));
#44807=CARTESIAN_POINT('',(8.83329938588935,-0.76435,26.5000000000004));
#44808=CARTESIAN_POINT('Ctrl Pts',(11.8332993858894,-0.764247147692691,
26.500050461596));
#44809=CARTESIAN_POINT('Ctrl Pts',(11.8404392777974,-0.764200213145106,
26.4142992027336));
#44810=CARTESIAN_POINT('Ctrl Pts',(11.8581647052059,-0.728620187353754,
26.2013042703026));
#44811=CARTESIAN_POINT('Ctrl Pts',(11.8864756681149,-0.534515160588541,
25.9092978259331));
#44812=CARTESIAN_POINT('Ctrl Pts',(11.9182322746166,-0.186908610932021,
25.7252821486098));
#44813=CARTESIAN_POINT('Ctrl Pts',(11.9499888811181,0.206614996502733,25.7307004175932));
#44814=CARTESIAN_POINT('Ctrl Pts',(11.9817454876198,0.549294672995457,25.9225373664711));
#44815=CARTESIAN_POINT('Ctrl Pts',(12.0135020941213,0.758915838938966,26.2570703655453));
#44816=CARTESIAN_POINT('Ctrl Pts',(12.0452587006229,0.782128837256907,26.6472169046534));
#44817=CARTESIAN_POINT('Ctrl Pts',(12.0876008426251,0.562204459925782,27.1277809604453));
#44818=CARTESIAN_POINT('Ctrl Pts',(12.1299429846272,0.0338737476163272,
27.3420423732096));
#44819=CARTESIAN_POINT('Ctrl Pts',(12.1722851266293,-0.458655982287092,
27.15040988999));
#44820=CARTESIAN_POINT('Ctrl Pts',(12.2032087485499,-0.707058563347677,
26.862068242422));
#44821=CARTESIAN_POINT('Ctrl Pts',(12.2235468349699,-0.764307937938393,
26.617097923109));
#44822=CARTESIAN_POINT('Ctrl Pts',(12.2332993858894,-0.764442058872939,
26.49989355797));
#44823=CARTESIAN_POINT('Ctrl Pts',(11.9667006141106,-0.764330172794591,
26.5000194733099));
#44824=CARTESIAN_POINT('Ctrl Pts',(11.9743314964896,-0.7642422449594,26.4083952726879));
#44825=CARTESIAN_POINT('Ctrl Pts',(11.9925715817669,-0.724832682225659,
26.1893125034889));
#44826=CARTESIAN_POINT('Ctrl Pts',(12.0214208699425,-0.520221631970104,
25.8962907861735));
#44827=CARTESIAN_POINT('Ctrl Pts',(12.0532484786374,-0.167145187013454,
25.720796658319));
#44828=CARTESIAN_POINT('Ctrl Pts',(12.0850760873322,0.226845720661642,25.7360390191599));
#44829=CARTESIAN_POINT('Ctrl Pts',(12.116903696027,0.565308431882582,25.9382867830725));
#44830=CARTESIAN_POINT('Ctrl Pts',(12.1487313047218,0.76539269994308,26.2780329391498));
#44831=CARTESIAN_POINT('Ctrl Pts',(12.1805589134166,0.778121103043664,26.6721130739564));
#44832=CARTESIAN_POINT('Ctrl Pts',(12.2123865221114,0.600377932120684,27.0240626869479));
#44833=CARTESIAN_POINT('Ctrl Pts',(12.2442141308062,0.275671866485382,27.2477301540376));
#44834=CARTESIAN_POINT('Ctrl Pts',(12.2760417395011,-0.116514253498911,
27.2883652643034));
#44835=CARTESIAN_POINT('Ctrl Pts',(12.3078693481959,-0.480179551758527,
27.1360211940663));
#44836=CARTESIAN_POINT('Ctrl Pts',(12.3380889730657,-0.713869945077878,
26.8435516129409));
#44837=CARTESIAN_POINT('Ctrl Pts',(12.3576993950373,-0.764277085342196,
26.6080399949409));
#44838=CARTESIAN_POINT('Ctrl Pts',(12.3667006141106,-0.764381481730689,
26.4999830130677));
#44839=CARTESIAN_POINT('Origin',(8.83329938588935,0.,26.5));
#44840=CARTESIAN_POINT('',(11.4332993858894,-0.764316846204452,26.499991976129));
#44841=CARTESIAN_POINT('',(11.5667006141106,-0.76432783921912,26.4999807307349));
#44842=CARTESIAN_POINT('',(8.83329938588935,-0.76435,26.5000000000004));
#44843=CARTESIAN_POINT('Ctrl Pts',(11.4332993858894,-0.764316846204371,
26.499991976129));
#44844=CARTESIAN_POINT('Ctrl Pts',(11.4361606496238,-0.764339507108424,
26.4656360034336));
#44845=CARTESIAN_POINT('Ctrl Pts',(11.4496074488587,-0.753617458541854,
26.3041929838167));
#44846=CARTESIAN_POINT('Ctrl Pts',(11.4736397835942,-0.64225832786655,26.028166535323));
#44847=CARTESIAN_POINT('Ctrl Pts',(11.5053963900958,-0.337898373364977,
25.7786566049734));
#44848=CARTESIAN_POINT('Ctrl Pts',(11.5371529965974,0.0477483654022483,
25.704444958218));
#44849=CARTESIAN_POINT('Ctrl Pts',(11.568909603099,0.423642753883886,25.8250963957939));
#44850=CARTESIAN_POINT('Ctrl Pts',(11.6006662096006,0.692865902039955,26.1084196418678));
#44851=CARTESIAN_POINT('Ctrl Pts',(11.6430083516027,0.834479137823284,26.6175897852527));
#44852=CARTESIAN_POINT('Ctrl Pts',(11.6853504936048,0.568651082127304,27.1219475346471));
#44853=CARTESIAN_POINT('Ctrl Pts',(11.727692635607,0.0685686419494346,27.2929039515766));
#44854=CARTESIAN_POINT('Ctrl Pts',(11.7594492421086,-0.31732463510849,27.2309398975579));
#44855=CARTESIAN_POINT('Ctrl Pts',(11.7912058486102,-0.629310976686018,
26.9890351986573));
#44856=CARTESIAN_POINT('Ctrl Pts',(11.8158225632038,-0.750814573790938,
26.7099080364726));
#44857=CARTESIAN_POINT('Ctrl Pts',(11.8298537422968,-0.764269797856761,
26.5414331995225));
#44858=CARTESIAN_POINT('Ctrl Pts',(11.8332993858894,-0.764247147692691,
26.500050461596));
#44859=CARTESIAN_POINT('Ctrl Pts',(11.5667006141106,-0.764327839218945,
26.4999807307349));
#44860=CARTESIAN_POINT('Ctrl Pts',(11.5697451921454,-0.764362384129928,
26.4634240836987));
#44861=CARTESIAN_POINT('Ctrl Pts',(11.5833989730785,-0.752814048677305,
26.2995029900743));
#44862=CARTESIAN_POINT('Ctrl Pts',(11.6076619569099,-0.637582094773173,
26.0218949554196));
#44863=CARTESIAN_POINT('Ctrl Pts',(11.6394895656047,-0.330353663928771,
25.7747677489538));
#44864=CARTESIAN_POINT('Ctrl Pts',(11.6713171742995,0.0577400488194873,
25.7051657732641));
#44865=CARTESIAN_POINT('Ctrl Pts',(11.7031447829944,0.431699923094752,25.8301264763938));
#44866=CARTESIAN_POINT('Ctrl Pts',(11.7349723916892,0.69998657563618,26.1190614811315));
#44867=CARTESIAN_POINT('Ctrl Pts',(11.766800000384,0.796927734095428,26.5012441294702));
#44868=CARTESIAN_POINT('Ctrl Pts',(11.7986276090788,0.698793756689006,26.883122234856));
#44869=CARTESIAN_POINT('Ctrl Pts',(11.8304552177736,0.42960626815974,27.1712181579684));
#44870=CARTESIAN_POINT('Ctrl Pts',(11.8622828264684,0.055258051066885,27.2950106345332));
#44871=CARTESIAN_POINT('Ctrl Pts',(11.8941104351633,-0.332616451231466,
27.2241972504773));
#44872=CARTESIAN_POINT('Ctrl Pts',(11.9259380438581,-0.639071777563019,
26.9761119871953));
#44873=CARTESIAN_POINT('Ctrl Pts',(11.9501347701738,-0.753124084686165,
26.698904588869));
#44874=CARTESIAN_POINT('Ctrl Pts',(11.9637222935913,-0.764364490880332,
26.5357802442425));
#44875=CARTESIAN_POINT('Ctrl Pts',(11.9667006141106,-0.764330172794591,
26.5000194733099));
#44876=CARTESIAN_POINT('Origin',(8.83329938588935,0.,26.5));
#44877=CARTESIAN_POINT('',(11.0332993858894,-0.764414335147055,26.5000295538604));
#44878=CARTESIAN_POINT('',(11.1667006141106,-0.764383820028244,26.5000165411639));
#44879=CARTESIAN_POINT('',(8.83329938588935,-0.76435,26.5000000000004));
#44880=CARTESIAN_POINT('Ctrl Pts',(11.0332993858894,-0.764414335146974,
26.5000295538604));
#44881=CARTESIAN_POINT('Ctrl Pts',(11.0424675569507,-0.764269334783866,
26.3899624749499));
#44882=CARTESIAN_POINT('Ctrl Pts',(11.0622212635126,-0.712269135825712,
26.1526701198256));
#44883=CARTESIAN_POINT('Ctrl Pts',(11.092560505575,-0.476282880095,25.8609832951857));
#44884=CARTESIAN_POINT('Ctrl Pts',(11.1243171120767,-0.111125768016633,
25.7109378214796));
#44885=CARTESIAN_POINT('Ctrl Pts',(11.1560737185782,0.277329037821362,25.7540194775561));
#44886=CARTESIAN_POINT('Ctrl Pts',(11.1984158605804,0.713793524031026,26.0520250072723));
#44887=CARTESIAN_POINT('Ctrl Pts',(11.2407580025825,0.835647851523945,26.6089745718114));
#44888=CARTESIAN_POINT('Ctrl Pts',(11.2831001445846,0.563503958616806,27.0620156792366));
#44889=CARTESIAN_POINT('Ctrl Pts',(11.3148567510862,0.228530189829721,27.2633754058293));
#44890=CARTESIAN_POINT('Ctrl Pts',(11.3466133575878,-0.165922069656989,
27.2795239558244));
#44891=CARTESIAN_POINT('Ctrl Pts',(11.3783699640894,-0.517860513634208,
27.1052537424003));
#44892=CARTESIAN_POINT('Ctrl Pts',(11.4072653068566,-0.724305932574169,
26.8126503890575));
#44893=CARTESIAN_POINT('Ctrl Pts',(11.4255751141233,-0.764255670794614,
26.5927394103127));
#44894=CARTESIAN_POINT('Ctrl Pts',(11.4332993858894,-0.764316846204371,
26.499991976129));
#44895=CARTESIAN_POINT('Ctrl Pts',(11.1667006141106,-0.764383820028068,
26.5000165411639));
#44896=CARTESIAN_POINT('Ctrl Pts',(11.1757680906995,-0.764280459239413,
26.3911651193886));
#44897=CARTESIAN_POINT('Ctrl Pts',(11.1954447701866,-0.713308165354942,
26.1548607868991));
#44898=CARTESIAN_POINT('Ctrl Pts',(11.2257306525721,-0.478191357872257,
25.8624826382875));
#44899=CARTESIAN_POINT('Ctrl Pts',(11.2575582612669,-0.114052167341973,
25.7112747852685));
#44900=CARTESIAN_POINT('Ctrl Pts',(11.2893858699617,0.278005165684963,25.7531342228479));
#44901=CARTESIAN_POINT('Ctrl Pts',(11.3212134786565,0.6020112901178,25.977814431644));
#44902=CARTESIAN_POINT('Ctrl Pts',(11.3530410873514,0.778654699980662,26.3303172977978));
#44903=CARTESIAN_POINT('Ctrl Pts',(11.3848686960462,0.764695919842463,26.7243557697161));
#44904=CARTESIAN_POINT('Ctrl Pts',(11.416696304741,0.563551835344745,27.0634755452618));
#44905=CARTESIAN_POINT('Ctrl Pts',(11.4485239134358,0.224459294363696,27.2646655389139));
#44906=CARTESIAN_POINT('Ctrl Pts',(11.4803515221306,-0.169577284164262,
27.2786776649706));
#44907=CARTESIAN_POINT('Ctrl Pts',(11.5121791308255,-0.522104061573776,
27.1020819795649));
#44908=CARTESIAN_POINT('Ctrl Pts',(11.5409621614854,-0.725331388674681,
26.8090972724894));
#44909=CARTESIAN_POINT('Ctrl Pts',(11.5591359892471,-0.7642420081811,26.5908101717706));
#44910=CARTESIAN_POINT('Ctrl Pts',(11.5667006141106,-0.764327839218945,
26.4999807307349));
#44911=CARTESIAN_POINT('Origin',(8.83329938588935,0.,26.5));
#44912=CARTESIAN_POINT('',(10.6332993858894,-0.764353038715178,26.5000780441916));
#44913=CARTESIAN_POINT('',(10.7667006141106,-0.76429020563518,26.4999910099171));
#44914=CARTESIAN_POINT('',(8.83329938588935,-0.76435,26.5000000000004));
#44915=CARTESIAN_POINT('Ctrl Pts',(10.6332993858894,-0.764353038715098,
26.5000780441916));
#44916=CARTESIAN_POINT('Ctrl Pts',(10.6381889287772,-0.76439544040222,26.4414009892152));
#44917=CARTESIAN_POINT('Ctrl Pts',(10.6536640071655,-0.743302438196824,
26.2556450156638));
#44918=CARTESIAN_POINT('Ctrl Pts',(10.6797246210543,-0.593564624338813,
25.9683524714423));
#44919=CARTESIAN_POINT('Ctrl Pts',(10.7114812275559,-0.268803421489938,
25.7509051757754));
#44920=CARTESIAN_POINT('Ctrl Pts',(10.753823369558,0.25697906207964,25.6974138359586));
#44921=CARTESIAN_POINT('Ctrl Pts',(10.7961655115601,0.709133976254987,26.0446849521718));
#44922=CARTESIAN_POINT('Ctrl Pts',(10.8385076535623,0.793082515708411,26.5664714853321));
#44923=CARTESIAN_POINT('Ctrl Pts',(10.8702642600639,0.666769034948869,26.9363337162334));
#44924=CARTESIAN_POINT('Ctrl Pts',(10.9020208665655,0.375600348367009,27.2029310842536));
#44925=CARTESIAN_POINT('Ctrl Pts',(10.9337774730671,-0.00580221503551052,
27.2965412346965));
#44926=CARTESIAN_POINT('Ctrl Pts',(10.9655340795687,-0.386547155848502,
27.1969245830134));
#44927=CARTESIAN_POINT('Ctrl Pts',(10.9972906860703,-0.672567178598631,
26.9269530484939));
#44928=CARTESIAN_POINT('Ctrl Pts',(11.0198791215105,-0.759771192940516,
26.6611311283238));
#44929=CARTESIAN_POINT('Ctrl Pts',(11.0318820214502,-0.764436751652618,
26.517045506391));
#44930=CARTESIAN_POINT('Ctrl Pts',(11.0332993858894,-0.764414335146974,
26.5000295538604));
#44931=CARTESIAN_POINT('Ctrl Pts',(10.7667006141106,-0.764290205635005,
26.4999910099171));
#44932=CARTESIAN_POINT('Ctrl Pts',(10.7711817863553,-0.764312357801265,
26.4461773955807));
#44933=CARTESIAN_POINT('Ctrl Pts',(10.7862721614982,-0.745445842461897,
26.2649750263996));
#44934=CARTESIAN_POINT('Ctrl Pts',(10.8119717395395,-0.603779637374724,
25.9798601046639));
#44935=CARTESIAN_POINT('Ctrl Pts',(10.8437993482343,-0.280537733984753,
25.7540818134411));
#44936=CARTESIAN_POINT('Ctrl Pts',(10.8756269569291,0.111375310126204,25.7108923384462));
#44937=CARTESIAN_POINT('Ctrl Pts',(10.9074545656239,0.476025463481309,25.8608637709017));
#44938=CARTESIAN_POINT('Ctrl Pts',(10.9392821743187,0.724152213281463,26.1672855079379));
#44939=CARTESIAN_POINT('Ctrl Pts',(10.9711097830136,0.795018108239294,26.5551504197647));
#44940=CARTESIAN_POINT('Ctrl Pts',(11.0029373917084,0.671276313132874,26.9295153928038));
#44941=CARTESIAN_POINT('Ctrl Pts',(11.0347650004032,0.383216836026789,27.1987418821097));
#44942=CARTESIAN_POINT('Ctrl Pts',(11.066592609098,0.00135201979696231,
27.2969275583584));
#44943=CARTESIAN_POINT('Ctrl Pts',(11.0984202177928,-0.380843749208507,
27.2000381417591));
#44944=CARTESIAN_POINT('Ctrl Pts',(11.1302478264876,-0.669815072706669,
26.9317906085171));
#44945=CARTESIAN_POINT('Ctrl Pts',(11.1530079585936,-0.759211496005515,
26.6643815455522));
#44946=CARTESIAN_POINT('Ctrl Pts',(11.1651588878012,-0.7644013942722,26.5185243475109));
#44947=CARTESIAN_POINT('Ctrl Pts',(11.1667006141106,-0.764383820028068,
26.5000165411639));
#44948=CARTESIAN_POINT('Origin',(8.83329938588935,0.,26.5));
#44949=CARTESIAN_POINT('',(10.2332993858894,-0.764421590778621,26.4997053810623));
#44950=CARTESIAN_POINT('',(10.3667006141106,-0.764415943136787,26.5000013527853));
#44951=CARTESIAN_POINT('',(8.83329938588935,-0.76435,26.5000000000004));
#44952=CARTESIAN_POINT('Ctrl Pts',(10.2332993858894,-0.764421590778541,
26.4997053810623));
#44953=CARTESIAN_POINT('Ctrl Pts',(10.2339103006036,-0.764425134242162,
26.4923794589594));
#44954=CARTESIAN_POINT('Ctrl Pts',(10.2451067508183,-0.762525940900646,
26.3581546174279));
#44955=CARTESIAN_POINT('Ctrl Pts',(10.2668887365335,-0.688355039348421,
26.1005432767371));
#44956=CARTESIAN_POINT('Ctrl Pts',(10.3092308785357,-0.320848092753299,
25.720744399325));
#44957=CARTESIAN_POINT('Ctrl Pts',(10.3515730205378,0.24868545684196,25.6948054070466));
#44958=CARTESIAN_POINT('Ctrl Pts',(10.3939151625399,0.649194652036547,26.0396255450656));
#44959=CARTESIAN_POINT('Ctrl Pts',(10.4256717690415,0.791023092992396,26.403820353824));
#44960=CARTESIAN_POINT('Ctrl Pts',(10.4574283755431,0.740250732337037,26.7953245403195));
#44961=CARTESIAN_POINT('Ctrl Pts',(10.4891849820447,0.508988374911209,27.1127335787333));
#44962=CARTESIAN_POINT('Ctrl Pts',(10.5209415885463,0.153681120282412,27.2819876542253));
#44963=CARTESIAN_POINT('Ctrl Pts',(10.5526981950479,-0.239009618237098,
27.2599407330431));
#44964=CARTESIAN_POINT('Ctrl Pts',(10.5844548015495,-0.573625316704213,
27.0532418767055));
#44965=CARTESIAN_POINT('Ctrl Pts',(10.6113218651633,-0.738145513096974,
26.7637621146551));
#44966=CARTESIAN_POINT('Ctrl Pts',(10.6276033932766,-0.764303643566683,
26.5684329148525));
#44967=CARTESIAN_POINT('Ctrl Pts',(10.6332993858894,-0.764353038715098,
26.5000780441916));
#44968=CARTESIAN_POINT('Ctrl Pts',(10.3667006141106,-0.764415943136612,
26.5000013527853));
#44969=CARTESIAN_POINT('Ctrl Pts',(10.3772046849093,-0.764402983620275,
26.3739195564708));
#44970=CARTESIAN_POINT('Ctrl Pts',(10.3983179586064,-0.700392143844539,
26.1204813744118));
#44971=CARTESIAN_POINT('Ctrl Pts',(10.4300404352017,-0.433970366467297,
25.8315951210098));
#44972=CARTESIAN_POINT('Ctrl Pts',(10.4618680438965,-0.0604366454286784,
25.7053662648007));
#44973=CARTESIAN_POINT('Ctrl Pts',(10.4936956525913,0.327890997713297,25.7736510102933));
#44974=CARTESIAN_POINT('Ctrl Pts',(10.5255232612861,0.635956180167181,26.0197343462881));
#44975=CARTESIAN_POINT('Ctrl Pts',(10.5573508699809,0.78834948304845,26.3833790164421));
#44976=CARTESIAN_POINT('Ctrl Pts',(10.5891784786757,0.747767468424727,26.775570634129));
#44977=CARTESIAN_POINT('Ctrl Pts',(10.6210060873706,0.524143963013505,27.1003069775249));
#44978=CARTESIAN_POINT('Ctrl Pts',(10.6528336960654,0.172218416622154,27.2780977947564));
#44979=CARTESIAN_POINT('Ctrl Pts',(10.6846613047602,-0.221863437780272,
27.2654227434594));
#44980=CARTESIAN_POINT('Ctrl Pts',(10.716488913455,-0.561636678720128,27.0653844730313));
#44981=CARTESIAN_POINT('Ctrl Pts',(10.7438353499051,-0.735448311725334,
26.7745991910558));
#44982=CARTESIAN_POINT('Ctrl Pts',(10.760572583457,-0.764259912411162,26.5735814590732));
#44983=CARTESIAN_POINT('Ctrl Pts',(10.7667006141106,-0.764290205635005,
26.4999910099171));
#44984=CARTESIAN_POINT('Origin',(8.83329938588935,0.,26.5));
#44985=CARTESIAN_POINT('',(9.83329938588937,-0.764354837691132,26.4999637734947));
#44986=CARTESIAN_POINT('',(9.96670061411062,-0.764287395473983,26.5000068045578));
#44987=CARTESIAN_POINT('',(8.83329938588935,-0.76435,26.5000000000004));
#44988=CARTESIAN_POINT('Ctrl Pts',(9.83329938588939,-0.764354837691052,
26.4999637734947));
#44989=CARTESIAN_POINT('Ctrl Pts',(9.84021720793052,-0.764621482654753,
26.4165337381156));
#44990=CARTESIAN_POINT('Ctrl Pts',(9.86830610097272,-0.711315275771919,
26.0775144141055));
#44991=CARTESIAN_POINT('Ctrl Pts',(9.90698052951547,-0.328871142664085,
25.7240954537507));
#44992=CARTESIAN_POINT('Ctrl Pts',(9.94932267151757,0.199598255234956,25.7295723838951));
#44993=CARTESIAN_POINT('Ctrl Pts',(9.98107927801918,0.542780303630156,25.9165983405945));
#44994=CARTESIAN_POINT('Ctrl Pts',(10.0128358845208,0.756313557236772,26.2486482930385));
#44995=CARTESIAN_POINT('Ctrl Pts',(10.0445924910224,0.784093796915711,26.6403866625412));
#44996=CARTESIAN_POINT('Ctrl Pts',(10.076349097524,0.621540241153639,26.9988089464404));
#44997=CARTESIAN_POINT('Ctrl Pts',(10.1081057040256,0.307098718342552,27.235068614701));
#44998=CARTESIAN_POINT('Ctrl Pts',(10.1398623105272,-0.0819621986926931,
27.2927198636753));
#44999=CARTESIAN_POINT('Ctrl Pts',(10.1716189170288,-0.451183699623203,
27.1564639171439));
#45000=CARTESIAN_POINT('Ctrl Pts',(10.2027646088162,-0.70535559423304,26.8670671390887));
#45001=CARTESIAN_POINT('Ctrl Pts',(10.223324765103,-0.764363735393704,26.619318304422));
#45002=CARTESIAN_POINT('Ctrl Pts',(10.2332993858894,-0.764421590778541,
26.4997053810623));
#45003=CARTESIAN_POINT('Ctrl Pts',(9.96670061411058,-0.764287395473808,
26.5000068045578));
#45004=CARTESIAN_POINT('Ctrl Pts',(9.97261838056512,-0.764265365977669,
26.4289406306763));
#45005=CARTESIAN_POINT('Ctrl Pts',(9.98914534991794,-0.736818813278755,
26.2304523735062));
#45006=CARTESIAN_POINT('Ctrl Pts',(10.016281522169,-0.567211114828819,25.9402081539091));
#45007=CARTESIAN_POINT('Ctrl Pts',(10.0481091308639,-0.229436586427856,
25.7368131175217));
#45008=CARTESIAN_POINT('Ctrl Pts',(10.0799367395587,0.164500331356799,25.7202340098908));
#45009=CARTESIAN_POINT('Ctrl Pts',(10.1117643482535,0.518170209717155,25.8945291116224));
#45010=CARTESIAN_POINT('Ctrl Pts',(10.1435919569483,0.745000323495275,26.2170337856481));
#45011=CARTESIAN_POINT('Ctrl Pts',(10.1754195656431,0.789466300620247,26.608804051599));
#45012=CARTESIAN_POINT('Ctrl Pts',(10.207247174338,0.640683580453765,26.9739408306562));
#45013=CARTESIAN_POINT('Ctrl Pts',(10.2390747830327,0.335071789291362,27.2230644903377));
#45014=CARTESIAN_POINT('Ctrl Pts',(10.2709023917276,-0.0525602054491083,
27.2951935525961));
#45015=CARTESIAN_POINT('Ctrl Pts',(10.3027300004224,-0.427326304238472,
27.1726719786772));
#45016=CARTESIAN_POINT('Ctrl Pts',(10.3345576091172,-0.697489773146787,
26.8854910862812));
#45017=CARTESIAN_POINT('Ctrl Pts',(10.3558811470133,-0.764104306192731,
26.629868829569));
#45018=CARTESIAN_POINT('Ctrl Pts',(10.3665954820111,-0.764416072844531,
26.5012632677334));
#45019=CARTESIAN_POINT('Ctrl Pts',(10.3667006141106,-0.764415943136612,
26.5000013527853));
#45020=CARTESIAN_POINT('Origin',(26.4823223304703,0.,26.5));
#45021=CARTESIAN_POINT('',(26.5,0.85,26.5));
#45022=CARTESIAN_POINT('Origin',(26.5,0.,26.5));
#45023=CARTESIAN_POINT('',(26.4646446609407,0.935355339059328,26.5));
#45024=CARTESIAN_POINT('',(26.4823223304703,0.892677669529664,26.5));
#45025=CARTESIAN_POINT('',(26.4646446609407,-0.935355339059328,26.5));
#45026=CARTESIAN_POINT('Origin',(26.4646446609407,0.,26.5));
#45027=CARTESIAN_POINT('Origin',(26.4646446609407,0.,26.5));
#45028=CARTESIAN_POINT('Origin',(26.45,0.,26.5));
#45029=CARTESIAN_POINT('',(26.4428553390593,-0.957144660940674,26.5));
#45030=CARTESIAN_POINT('',(26.45,-0.95,26.5));
#45031=CARTESIAN_POINT('',(26.4428553390593,-0.887111235409736,26.1407706464662));
#45032=CARTESIAN_POINT('Origin',(26.4428553390593,0.,26.5));
#45033=CARTESIAN_POINT('',(26.4428553390593,0.547713856063688,27.2849429494193));
#45034=CARTESIAN_POINT('Origin',(26.4428553390593,0.,26.5));
#45035=CARTESIAN_POINT('Origin',(26.4428553390593,0.,26.5));
#45036=CARTESIAN_POINT('Origin',(26.5,0.,26.5));
#45037=CARTESIAN_POINT('Origin',(1.375,0.,26.5));
#45038=CARTESIAN_POINT('',(1.35,-5.57214293612048E-17,26.045));
#45039=CARTESIAN_POINT('Origin',(1.35,0.,26.5));
#45040=CARTESIAN_POINT('',(1.4,4.95981953654679E-17,26.095));
#45041=CARTESIAN_POINT('',(1.375,-5.26598123633364E-17,26.07));
#45042=CARTESIAN_POINT('Origin',(1.4,0.,26.5));
#45043=CARTESIAN_POINT('Origin',(2.16,0.,26.5));
#45044=CARTESIAN_POINT('',(3.,-4.95981953654679E-17,26.095));
#45045=CARTESIAN_POINT('Origin',(3.,0.,26.5));
#45046=CARTESIAN_POINT('',(2.16,-4.95981953654679E-17,26.095));
#45047=CARTESIAN_POINT('Origin',(1.35,0.95,26.5));
#45048=CARTESIAN_POINT('',(1.35,-0.95,26.5));
#45049=CARTESIAN_POINT('Origin',(1.35,0.,26.5));
#45050=CARTESIAN_POINT('Origin',(26.4001776695297,0.,26.5));
#45051=CARTESIAN_POINT('',(26.3575,-0.445914884024654,27.3865897013136));
#45052=CARTESIAN_POINT('Ctrl Pts',(26.3575,-0.445914873067339,27.3865896766146));
#45053=CARTESIAN_POINT('Ctrl Pts',(26.3600385435018,-0.48473316469248,27.3658905669609));
#45054=CARTESIAN_POINT('Ctrl Pts',(26.3625749249413,-0.52209630504398,27.3426935917771));
#45055=CARTESIAN_POINT('Ctrl Pts',(26.3651148458502,-0.557748585913535,
27.3171415526578));
#45056=CARTESIAN_POINT('Ctrl Pts',(26.3672683153527,-0.587976337997584,
27.2954772808384));
#45057=CARTESIAN_POINT('Ctrl Pts',(26.3694243291957,-0.61697427499121,27.2721190586853));
#45058=CARTESIAN_POINT('Ctrl Pts',(26.3715863623179,-0.644568450298925,
27.2471307664931));
#45059=CARTESIAN_POINT('Ctrl Pts',(26.3723323070778,-0.654088993838404,
27.2385093048571));
#45060=CARTESIAN_POINT('Ctrl Pts',(26.3730789683657,-0.663442253748417,
27.2296936320192));
#45061=CARTESIAN_POINT('Ctrl Pts',(26.3738264888999,-0.672623694624938,
27.2206895691609));
#45062=CARTESIAN_POINT('Ctrl Pts',(26.3744393486039,-0.680151160265756,
27.2133075280732));
#45063=CARTESIAN_POINT('Ctrl Pts',(26.3750523299018,-0.687557476799255,
27.2058043027306));
#45064=CARTESIAN_POINT('Ctrl Pts',(26.3756651421252,-0.694836304461934,
27.1981882490307));
#45065=CARTESIAN_POINT('Ctrl Pts',(26.3782136366893,-0.725106674441304,
27.1665154613291));
#45066=CARTESIAN_POINT('Ctrl Pts',(26.3807612316211,-0.753200182626468,
27.1328697487299));
#45067=CARTESIAN_POINT('Ctrl Pts',(26.3833137014739,-0.778965752445576,
27.0975076461287));
#45068=CARTESIAN_POINT('Ctrl Pts',(26.3847185728135,-0.793147040638668,
27.0780444566234));
#45069=CARTESIAN_POINT('Ctrl Pts',(26.3861249209455,-0.806622431718545,
27.0580606680849));
#45070=CARTESIAN_POINT('Ctrl Pts',(26.3875337086924,-0.819361091867474,
27.037595384434));
#45071=CARTESIAN_POINT('Ctrl Pts',(26.3882388148024,-0.825736862188447,
27.0273523960361));
#45072=CARTESIAN_POINT('Ctrl Pts',(26.3889445320502,-0.831928009592696,
27.016988757215));
#45073=CARTESIAN_POINT('Ctrl Pts',(26.389650981154,-0.837930241239925,27.0065092037505));
#45074=CARTESIAN_POINT('Ctrl Pts',(26.3903079381786,-0.843511971364541,
26.9967638219154));
#45075=CARTESIAN_POINT('Ctrl Pts',(26.3909656943287,-0.848931490642638,
26.9869156056837));
#45076=CARTESIAN_POINT('Ctrl Pts',(26.3916229242783,-0.854174248581219,
26.9769900217494));
#45077=CARTESIAN_POINT('Ctrl Pts',(26.3941734457713,-0.874519892922855,
26.9384716688187));
#45078=CARTESIAN_POINT('Ctrl Pts',(26.3967204402416,-0.892245792594232,
26.8987257442745));
#45079=CARTESIAN_POINT('Ctrl Pts',(26.3992697018428,-0.907198345124913,
26.8579958866988));
#45080=CARTESIAN_POINT('Ctrl Pts',(26.3995912211097,-0.909084198552438,
26.8528589349072));
#45081=CARTESIAN_POINT('Ctrl Pts',(26.3999127764396,-0.910925876275156,
26.8477063004776));
#45082=CARTESIAN_POINT('Ctrl Pts',(26.4002343794568,-0.91272301636638,26.8425384475368));
#45083=CARTESIAN_POINT('Ctrl Pts',(26.4026046454671,-0.925968228151,26.8044505394169));
#45084=CARTESIAN_POINT('Ctrl Pts',(26.404977501818,-0.936797324660802,26.7655365317526));
#45085=CARTESIAN_POINT('Ctrl Pts',(26.4073576022132,-0.945188176582006,
26.7260336212008));
#45086=CARTESIAN_POINT('Ctrl Pts',(26.4085446489769,-0.949373014178511,
26.7063320144032));
#45087=CARTESIAN_POINT('Ctrl Pts',(26.409733497622,-0.95295076699331,26.6864838163494));
#45088=CARTESIAN_POINT('Ctrl Pts',(26.4109247254682,-0.9559150864139,26.6665183261861));
#45089=CARTESIAN_POINT('Ctrl Pts',(26.4115344172028,-0.957432278154629,
26.6562996309385));
#45090=CARTESIAN_POINT('Ctrl Pts',(26.4121447321872,-0.958788737392734,
26.6460502130111));
#45091=CARTESIAN_POINT('Ctrl Pts',(26.4127557478252,-0.959983365913965,
26.6357740370122));
#45092=CARTESIAN_POINT('Ctrl Pts',(26.4132604827156,-0.960970199405942,
26.6272853106299));
#45093=CARTESIAN_POINT('Ctrl Pts',(26.4137651979061,-0.961845594431708,
26.6187866986054));
#45094=CARTESIAN_POINT('Ctrl Pts',(26.4142697129421,-0.962609265207646,
26.610284282333));
#45095=CARTESIAN_POINT('Ctrl Pts',(26.4168249481992,-0.966477055763842,
26.5672217920562));
#45096=CARTESIAN_POINT('Ctrl Pts',(26.4193769127223,-0.967486752456094,
26.5240309369813));
#45097=CARTESIAN_POINT('Ctrl Pts',(26.4219314366751,-0.965628032162785,
26.4810033974626));
#45098=CARTESIAN_POINT('Ctrl Pts',(26.4242448807101,-0.963944726210391,
26.4420365267346));
#45099=CARTESIAN_POINT('Ctrl Pts',(26.4265604238843,-0.959908265275576,
26.4032027997282));
#45100=CARTESIAN_POINT('Ctrl Pts',(26.4288823965957,-0.953474131147185,
26.3647208517404));
#45101=CARTESIAN_POINT('Ctrl Pts',(26.4300930314562,-0.950119489193485,
26.3446570553377));
#45102=CARTESIAN_POINT('Ctrl Pts',(26.4313054141171,-0.946112458815371,
26.3246889932157));
#45103=CARTESIAN_POINT('Ctrl Pts',(26.4325201583348,-0.941463409934123,
26.3048454980279));
#45104=CARTESIAN_POINT('Ctrl Pts',(26.4332726276574,-0.938583571848533,
26.2925535099993));
#45105=CARTESIAN_POINT('Ctrl Pts',(26.434026003143,-0.935457335204475,26.2803093396821));
#45106=CARTESIAN_POINT('Ctrl Pts',(26.4347804306756,-0.93208672886211,26.2681200827888));
#45107=CARTESIAN_POINT('Ctrl Pts',(26.4352708940567,-0.929895452813088,
26.2601956846323));
#45108=CARTESIAN_POINT('Ctrl Pts',(26.4357617442608,-0.927601043197031,
26.2522954678643));
#45109=CARTESIAN_POINT('Ctrl Pts',(26.4362522637174,-0.925208062189623,
26.2444334515549));
#45110=CARTESIAN_POINT('Ctrl Pts',(26.4384546480274,-0.914463811876937,
26.2091337684695));
#45111=CARTESIAN_POINT('Ctrl Pts',(26.4406544289207,-0.901716958129345,
26.1745378725213));
#45112=CARTESIAN_POINT('Ctrl Pts',(26.4428553390593,-0.88706152092118,26.1408063078486));
#45113=CARTESIAN_POINT('',(26.3575,0.966230510866419,26.2733743026085));
#45114=CARTESIAN_POINT('Ctrl Pts',(26.4428553390593,0.547713856063654,27.2849429494193));
#45115=CARTESIAN_POINT('Ctrl Pts',(26.4398527288292,0.581338330917549,27.2629971879954));
#45116=CARTESIAN_POINT('Ctrl Pts',(26.436860740363,0.613498955065304,27.2389352067906));
#45117=CARTESIAN_POINT('Ctrl Pts',(26.43387340856,0.64405462111651,27.2129570307588));
#45118=CARTESIAN_POINT('Ctrl Pts',(26.4325435063468,0.657657411361345,27.201392050342));
#45119=CARTESIAN_POINT('Ctrl Pts',(26.431214527018,0.670941868034084,27.1894468235091));
#45120=CARTESIAN_POINT('Ctrl Pts',(26.429885944282,0.683894109675807,27.17713688103));
#45121=CARTESIAN_POINT('Ctrl Pts',(26.4286990874112,0.695464677746311,27.1661400951964));
#45122=CARTESIAN_POINT('Ctrl Pts',(26.4275121669376,0.706773475320743,27.1548483470153));
#45123=CARTESIAN_POINT('Ctrl Pts',(26.4263270971742,0.717789124043923,27.1432948309583));
#45124=CARTESIAN_POINT('Ctrl Pts',(26.4231131118946,0.747664270584715,27.1119609536771));
#45125=CARTESIAN_POINT('Ctrl Pts',(26.4199099302131,0.775414440024102,27.0786797677372));
#45126=CARTESIAN_POINT('Ctrl Pts',(26.4167102083011,0.800845389198238,27.0436744066156));
#45127=CARTESIAN_POINT('Ctrl Pts',(26.4158576282968,0.807621577677036,27.03434707388));
#45128=CARTESIAN_POINT('Ctrl Pts',(26.4150052939291,0.814232902380581,27.0248971262858));
#45129=CARTESIAN_POINT('Ctrl Pts',(26.4141530662695,0.820675210986602,27.0153283782149));
#45130=CARTESIAN_POINT('Ctrl Pts',(26.4134180785672,0.826231258770111,27.0070759915688));
#45131=CARTESIAN_POINT('Ctrl Pts',(26.4126831307285,0.831661755957179,26.9987347062046));
#45132=CARTESIAN_POINT('Ctrl Pts',(26.4119492862705,0.83695594675194,26.9903203427592));
#45133=CARTESIAN_POINT('Ctrl Pts',(26.4103406081986,0.848561469622691,26.9718750144373));
#45134=CARTESIAN_POINT('Ctrl Pts',(26.4087359032515,0.859522353428771,26.9530638762961));
#45135=CARTESIAN_POINT('Ctrl Pts',(26.4071342608444,0.869816503695763,26.9339165277584));
#45136=CARTESIAN_POINT('Ctrl Pts',(26.4039408162305,0.890341558838379,26.8957394685182));
#45137=CARTESIAN_POINT('Ctrl Pts',(26.4007595466296,0.908219032919032,26.8562276023525));
#45138=CARTESIAN_POINT('Ctrl Pts',(26.397583234291,0.923418683717435,26.8156799699147));
#45139=CARTESIAN_POINT('Ctrl Pts',(26.3953941841655,0.933893975168751,26.7877353629575));
#45140=CARTESIAN_POINT('Ctrl Pts',(26.3932074885846,0.943096493319833,26.7592980148124));
#45141=CARTESIAN_POINT('Ctrl Pts',(26.3910207848981,0.951003299464193,26.7304596282699));
#45142=CARTESIAN_POINT('Ctrl Pts',(26.3898435664395,0.955259952160194,26.7149343967689));
#45143=CARTESIAN_POINT('Ctrl Pts',(26.3886663456316,0.959140888050434,26.6992928697601));
#45144=CARTESIAN_POINT('Ctrl Pts',(26.3874887538361,0.962641160833331,26.6835490619002));
#45145=CARTESIAN_POINT('Ctrl Pts',(26.3868658035192,0.964492817789051,26.6752205306281));
#45146=CARTESIAN_POINT('Ctrl Pts',(26.3862427493833,0.966237931701423,26.6668633743709));
#45147=CARTESIAN_POINT('Ctrl Pts',(26.3856195368556,0.967875657393992,26.6584796596185));
#45148=CARTESIAN_POINT('Ctrl Pts',(26.3849599332623,0.969609014320487,26.6496063970802));
#45149=CARTESIAN_POINT('Ctrl Pts',(26.3843007260322,0.97122051053719,26.640711093987));
#45150=CARTESIAN_POINT('Ctrl Pts',(26.3836423162498,0.97270880060374,26.631802662497));
#45151=CARTESIAN_POINT('Ctrl Pts',(26.3804362994795,0.979955781192868,26.5884245391464));
#45152=CARTESIAN_POINT('Ctrl Pts',(26.3772457209939,0.984294585326509,26.5446899966097));
#45153=CARTESIAN_POINT('Ctrl Pts',(26.3740633661155,0.985682557969509,26.5008948307824));
#45154=CARTESIAN_POINT('Ctrl Pts',(26.3731793337966,0.98606812548825,26.488728889684));
#45155=CARTESIAN_POINT('Ctrl Pts',(26.3722959360797,0.986225688641236,26.4765581716034));
#45156=CARTESIAN_POINT('Ctrl Pts',(26.3714130183056,0.986153641580633,26.4643888432541));
#45157=CARTESIAN_POINT('Ctrl Pts',(26.3682371159129,0.985894484455392,26.4206151191807));
#45158=CARTESIAN_POINT('Ctrl Pts',(26.3650674234017,0.982668492420396,26.3768591088312));
#45159=CARTESIAN_POINT('Ctrl Pts',(26.3618967427,0.976554405390113,26.3334004690451));
#45160=CARTESIAN_POINT('Ctrl Pts',(26.360431609542,0.973729159809769,26.3133187578467));
#45161=CARTESIAN_POINT('Ctrl Pts',(26.3589662653804,0.970286500015859,26.2933005906444));
#45162=CARTESIAN_POINT('Ctrl Pts',(26.3575,0.96623051086643,26.2733743026086));
#45163=CARTESIAN_POINT('Origin',(26.3575,0.,26.5));
#45164=CARTESIAN_POINT('Ctrl Pts',(9.53886739174684,0.859794713971473,26.0042084108955));
#45165=CARTESIAN_POINT('Ctrl Pts',(9.54945292724737,0.942233552586438,26.1471726709289));
#45166=CARTESIAN_POINT('Ctrl Pts',(9.57062399824843,1.0343832675773,26.4749075185653));
#45167=CARTESIAN_POINT('Ctrl Pts',(9.60238060475003,0.920175290048848,26.97275433311));
#45168=CARTESIAN_POINT('Ctrl Pts',(9.63413721125163,0.582068997229128,27.3555560520742));
#45169=CARTESIAN_POINT('Ctrl Pts',(9.66589381775322,0.101541985274178,27.5293442666035));
#45170=CARTESIAN_POINT('Ctrl Pts',(9.69765042425481,-0.402736095057523,
27.4532967233332));
#45171=CARTESIAN_POINT('Ctrl Pts',(9.72940703075643,-0.810700494112901,
27.142932400863));
#45172=CARTESIAN_POINT('Ctrl Pts',(9.76116363725799,-1.01770239046896,26.6795633494522));
#45173=CARTESIAN_POINT('Ctrl Pts',(9.80350577926016,-0.970730317561869,
25.9949282231766));
#45174=CARTESIAN_POINT('Ctrl Pts',(9.84584792126225,-0.427035532274557,
25.4924965498102));
#45175=CARTESIAN_POINT('Ctrl Pts',(9.8881900632644,0.259176121306736,25.4996082828754));
#45176=CARTESIAN_POINT('Ctrl Pts',(9.91994666976598,0.704794205996023,25.7424594139335));
#45177=CARTESIAN_POINT('Ctrl Pts',(9.95170327626759,0.982064768178995,26.1736225954612));
#45178=CARTESIAN_POINT('Ctrl Pts',(9.98345988276918,1.01813710137885,26.6822905247233));
#45179=CARTESIAN_POINT('Ctrl Pts',(10.0152164892708,0.807063111591556,27.1476978862331));
#45180=CARTESIAN_POINT('Ctrl Pts',(10.0469730957724,0.398764280702476,27.454478445857));
#45181=CARTESIAN_POINT('Ctrl Pts',(10.078729702274,-0.106427006217827,27.5293379534217));
#45182=CARTESIAN_POINT('Ctrl Pts',(10.1104863087756,-0.585857031302619,
27.3524111176363));
#45183=CARTESIAN_POINT('Ctrl Pts',(10.1422429152771,-0.922370055714352,
26.9692618115817));
#45184=CARTESIAN_POINT('Ctrl Pts',(10.1739995217788,-1.03423474310886,26.4689953727654));
#45185=CARTESIAN_POINT('Ctrl Pts',(10.2057561282803,-0.893821386214883,
25.9813098739602));
#45186=CARTESIAN_POINT('Ctrl Pts',(10.2480982702825,-0.416617690923792,
25.4881452427944));
#45187=CARTESIAN_POINT('Ctrl Pts',(10.2904404122846,0.322915308321796,25.4544637489288));
#45188=CARTESIAN_POINT('Ctrl Pts',(10.3327825542867,0.84297205749513,25.9022088748317));
#45189=CARTESIAN_POINT('Ctrl Pts',(10.3645391607883,1.02713471550344,26.3751117958663));
#45190=CARTESIAN_POINT('Ctrl Pts',(10.39629576729,0.961207368148842,26.8834756410901));
#45191=CARTESIAN_POINT('Ctrl Pts',(10.4280523737915,0.660915761234207,27.2956277580859));
#45192=CARTESIAN_POINT('Ctrl Pts',(10.4598089802931,0.199553230693041,27.5154022984479));
#45193=CARTESIAN_POINT('Ctrl Pts',(10.4915655867947,-0.310351339177647,
27.4867746157459));
#45194=CARTESIAN_POINT('Ctrl Pts',(10.5233221932963,-0.744846113467733,
27.2183784426378));
#45195=CARTESIAN_POINT('Ctrl Pts',(10.5550787997979,-0.997351908038651,
26.7740845569543));
#45196=CARTESIAN_POINT('Ctrl Pts',(10.5868354062995,-1.00766660609549,26.2642433819351));
#45197=CARTESIAN_POINT('Ctrl Pts',(10.6185920128011,-0.770737083347005,
25.809661578997));
#45198=CARTESIAN_POINT('Ctrl Pts',(10.6503486193027,-0.34903826235195,25.527308676597));
#45199=CARTESIAN_POINT('Ctrl Pts',(10.6926907613048,0.333684462764655,25.4578507649491));
#45200=CARTESIAN_POINT('Ctrl Pts',(10.735032903307,0.920802605394399,25.9087784588611));
#45201=CARTESIAN_POINT('Ctrl Pts',(10.7773750453091,1.02980885306559,26.5863124866778));
#45202=CARTESIAN_POINT('Ctrl Pts',(10.8091316518107,0.865792198844485,27.0665744925254));
#45203=CARTESIAN_POINT('Ctrl Pts',(10.8408882583123,0.487712887753285,27.4127482189073));
#45204=CARTESIAN_POINT('Ctrl Pts',(10.8726448648139,-0.00753411188962321,
27.5342999613219));
#45205=CARTESIAN_POINT('Ctrl Pts',(10.9044014713155,-0.501927195891623,
27.4049488436461));
#45206=CARTESIAN_POINT('Ctrl Pts',(10.9361580778171,-0.873321024084869,
27.0543937994769));
#45207=CARTESIAN_POINT('Ctrl Pts',(10.9679146843187,-1.03251354487671,26.5691310294889));
#45208=CARTESIAN_POINT('Ctrl Pts',(10.9996712908203,-0.939188918406778,
26.0666902396964));
#45209=CARTESIAN_POINT('Ctrl Pts',(11.0314278973219,-0.618448038849054,
25.6702438941213));
#45210=CARTESIAN_POINT('Ctrl Pts',(11.0631845038235,-0.144295577623383,
25.4754115101961));
#45211=CARTESIAN_POINT('Ctrl Pts',(11.0949411103251,0.360108680627746,25.5313525629285));
#45212=CARTESIAN_POINT('Ctrl Pts',(11.1372832523272,0.92685297651721,25.9183094390236));
#45213=CARTESIAN_POINT('Ctrl Pts',(11.1796253943293,1.0850794696639,26.6415022732033));
#45214=CARTESIAN_POINT('Ctrl Pts',(11.2219675363315,0.731703642215195,27.229771127942));
#45215=CARTESIAN_POINT('Ctrl Pts',(11.253724142833,0.296743917584798,27.4912345002757));
#45216=CARTESIAN_POINT('Ctrl Pts',(11.2854807493346,-0.215447967730317,
27.5122032133915));
#45217=CARTESIAN_POINT('Ctrl Pts',(11.3172373558362,-0.672436134993237,
27.2859152735427));
#45218=CARTESIAN_POINT('Ctrl Pts',(11.3489939623378,-0.967047660490463,
26.8683505693385));
#45219=CARTESIAN_POINT('Ctrl Pts',(11.3807505688394,-1.02503958381233,26.3609462419604));
#45220=CARTESIAN_POINT('Ctrl Pts',(11.412507175341,-0.833965317469191,25.8873294777365));
#45221=CARTESIAN_POINT('Ctrl Pts',(11.4442637818426,-0.438757291247072,
25.5633435997069));
#45222=CARTESIAN_POINT('Ctrl Pts',(11.4760203883442,0.0620007230481136,
25.4669805992429));
#45223=CARTESIAN_POINT('Ctrl Pts',(11.5077769948458,0.550095418630056,25.6236451531699));
#45224=CARTESIAN_POINT('Ctrl Pts',(11.5395336013474,0.899678691404176,25.9915372467506));
#45225=CARTESIAN_POINT('Ctrl Pts',(11.5818757433495,1.08356190788212,26.6526890323327));
#45226=CARTESIAN_POINT('Ctrl Pts',(11.6242178853517,0.738387125023024,27.3075919776769));
#45227=CARTESIAN_POINT('Ctrl Pts',(11.6665600273538,0.089035621292253,27.5295769895203));
#45228=CARTESIAN_POINT('Ctrl Pts',(11.6983166338554,-0.412042520239806,
27.4491173524253));
#45229=CARTESIAN_POINT('Ctrl Pts',(11.730073240357,-0.817153325519727,27.1350067831064));
#45230=CARTESIAN_POINT('Ctrl Pts',(11.7618298468586,-1.02068470593394,26.6674392543729));
#45231=CARTESIAN_POINT('Ctrl Pts',(11.7935864533602,-0.976780670184819,
26.1582942172784));
#45232=CARTESIAN_POINT('Ctrl Pts',(11.8253430598618,-0.694062009399,25.7329797765925));
#45233=CARTESIAN_POINT('Ctrl Pts',(11.8570996663634,-0.242698758880051,
25.494037459927));
#45234=CARTESIAN_POINT('Ctrl Pts',(11.888856272865,0.268287282042353,25.5010730221249));
#45235=CARTESIAN_POINT('Ctrl Pts',(11.9206128793666,0.713253042386499,25.7501711731831));
#45236=CARTESIAN_POINT('Ctrl Pts',(11.9523694858682,0.985443802115579,26.1845585632287));
#45237=CARTESIAN_POINT('Ctrl Pts',(11.9841260923698,1.01558562304907,26.6911595183732));
#45238=CARTESIAN_POINT('Ctrl Pts',(12.0264682343719,0.730016257573543,27.3151666163958));
#45239=CARTESIAN_POINT('Ctrl Pts',(12.068810376374,0.0439846856925677,27.5933826851713));
#45240=CARTESIAN_POINT('Ctrl Pts',(12.1111525183761,-0.59555970749011,27.3445500305032));
#45241=CARTESIAN_POINT('Ctrl Pts',(12.1429091248777,-0.926796127759782,
26.960056219097));
#45242=CARTESIAN_POINT('Ctrl Pts',(12.1746657313793,-1.03405720104669,26.4587825648226));
#45243=CARTESIAN_POINT('Ctrl Pts',(12.2064223378809,-0.888287875944312,
25.9701152745334));
#45244=CARTESIAN_POINT('Ctrl Pts',(12.2381789443825,-0.526542903289158,
25.6091487831361));
#45245=CARTESIAN_POINT('Ctrl Pts',(12.2699355508841,-0.0362472532010614,
25.4662068714475));
#45246=CARTESIAN_POINT('Ctrl Pts',(12.3016921573857,0.462855827725006,25.5744581034156));
#45247=CARTESIAN_POINT('Ctrl Pts',(12.3334487638873,0.84899406708818,25.9092020253238));
#45248=CARTESIAN_POINT('Ctrl Pts',(12.3652053703889,1.0286310290053,26.3864597949332));
#45249=CARTESIAN_POINT('Ctrl Pts',(12.3969619768905,0.956741897977003,26.8940148827339));
#45250=CARTESIAN_POINT('Ctrl Pts',(12.4287185833921,0.653248336737492,27.3007638414404));
#45251=CARTESIAN_POINT('Ctrl Pts',(12.4710607253942,0.0327023948412893,
27.5937782692024));
#45252=CARTESIAN_POINT('Ctrl Pts',(12.5134028673963,-0.671130356429513,
27.3642941591187));
#45253=CARTESIAN_POINT('Ctrl Pts',(12.5557450093985,-0.99970306837254,26.7618203473666));
#45254=CARTESIAN_POINT('Ctrl Pts',(12.5875016159001,-1.00511692324876,26.2543523707434));
#45255=CARTESIAN_POINT('Ctrl Pts',(12.6192582224017,-0.764018502542225,
25.8019678375804));
#45256=CARTESIAN_POINT('Ctrl Pts',(12.6510148289033,-0.337591957320698,
25.5223165935821));
#45257=CARTESIAN_POINT('Ctrl Pts',(12.6827714354049,0.171646482149533,25.4795095273557));
#45258=CARTESIAN_POINT('Ctrl Pts',(12.7145280419065,0.638636511130495,25.6862521873097));
#45259=CARTESIAN_POINT('Ctrl Pts',(12.7462846484081,0.95044934996174,26.090720935364));
#45260=CARTESIAN_POINT('Ctrl Pts',(12.7780412549097,1.02990540953483,26.5955406732408));
#45261=CARTESIAN_POINT('Ctrl Pts',(12.8097978614112,0.859621652443963,27.0762150524315));
#45262=CARTESIAN_POINT('Ctrl Pts',(12.8415544679129,0.477505572712525,27.417927674269));
#45263=CARTESIAN_POINT('Ctrl Pts',(12.8733110744144,-0.0167067740529667,
27.5332845701497));
#45264=CARTESIAN_POINT('Ctrl Pts',(12.9156532164166,-0.680011184951963,
27.3573244060144));
#45265=CARTESIAN_POINT('Ctrl Pts',(12.9579953584187,-1.07020684387626,26.7282053025858));
#45266=CARTESIAN_POINT('Ctrl Pts',(13.0003375004208,-0.933081383677509,
26.055798187033));
#45267=CARTESIAN_POINT('Ctrl Pts',(13.0320941069224,-0.610123262522071,
25.6643251878333));
#45268=CARTESIAN_POINT('Ctrl Pts',(13.063850713424,-0.134199768795049,25.4738598565232));
#45269=CARTESIAN_POINT('Ctrl Pts',(13.0956073199256,0.372077658796297,25.5349137921113));
#45270=CARTESIAN_POINT('Ctrl Pts',(13.1273639264272,0.789006702860459,25.8304242071032));
#45271=CARTESIAN_POINT('Ctrl Pts',(13.1591205329288,1.01278323085218,26.289495312851));
#45272=CARTESIAN_POINT('Ctrl Pts',(13.1908771394304,0.990471642591059,26.7997152729092));
#45273=CARTESIAN_POINT('Ctrl Pts',(13.222633745932,0.725829276801039,27.2368887526424));
#45274=CARTESIAN_POINT('Ctrl Pts',(13.2543903524336,0.285812251560458,27.4946278343466));
#45275=CARTESIAN_POINT('Ctrl Pts',(13.2861469589352,-0.226590453210316,
27.5095838517302));
#45276=CARTESIAN_POINT('Ctrl Pts',(13.3179035654368,-0.678794583544352,
27.2792265604813));
#45277=CARTESIAN_POINT('Ctrl Pts',(13.3602457074389,-1.07250418465013,26.7171523030405));
#45278=CARTESIAN_POINT('Ctrl Pts',(13.4025878494411,-0.965317714357462,
25.9846534572198));
#45279=CARTESIAN_POINT('Ctrl Pts',(13.4449299914432,-0.427067129317259,
25.5589528246334));
#45280=CARTESIAN_POINT('Ctrl Pts',(13.4766865979448,0.0721804151245883,
25.4678213454867));
#45281=CARTESIAN_POINT('Ctrl Pts',(13.5084432044464,0.558814289916099,25.628966268515));
#45282=CARTESIAN_POINT('Ctrl Pts',(13.540199810948,0.906534092576322,26.0019747879583));
#45283=CARTESIAN_POINT('Ctrl Pts',(13.5719564174496,1.03481982305313,26.4966453899845));
#45284=CARTESIAN_POINT('Ctrl Pts',(13.6037130239512,0.910005392756522,26.9918661211764));
#45285=CARTESIAN_POINT('Ctrl Pts',(13.6354696304527,0.564076013020103,27.3675722281905));
#45286=CARTESIAN_POINT('Ctrl Pts',(13.6672262369544,0.0799566012888428,
27.5312323282087));
#45287=CARTESIAN_POINT('Ctrl Pts',(13.6989828434559,-0.422587531096607,
27.4446655231143));
#45288=CARTESIAN_POINT('Ctrl Pts',(13.7307394499576,-0.823983930738844,
27.1258220745904));
#45289=CARTESIAN_POINT('Ctrl Pts',(13.7624960564592,-1.02123471647093,26.6582269669911));
#45290=CARTESIAN_POINT('Ctrl Pts',(13.8048381984613,-0.959949738419397,
25.974722122571));
#45291=CARTESIAN_POINT('Ctrl Pts',(13.8471803404634,-0.405855769996725,
25.4837808096832));
#45292=CARTESIAN_POINT('Ctrl Pts',(13.8895224824656,0.280055116964015,25.5052511620158));
#45293=CARTESIAN_POINT('Ctrl Pts',(13.9212790889671,0.720493983616905,25.7573754604565));
#45294=CARTESIAN_POINT('Ctrl Pts',(13.9530356954688,0.988679976891274,26.1942467084504));
#45295=CARTESIAN_POINT('Ctrl Pts',(13.9847923019703,1.01409920541245,26.703558282598));
#45296=CARTESIAN_POINT('Ctrl Pts',(14.0165489084719,0.793331246795938,27.1644462750661));
#45297=CARTESIAN_POINT('Ctrl Pts',(14.0483055149735,0.378701581549496,27.4626147766054));
#45298=CARTESIAN_POINT('Ctrl Pts',(14.0800621214751,-0.1279457593323,27.5268851942944));
#45299=CARTESIAN_POINT('Ctrl Pts',(14.1118187279767,-0.60356802732903,27.3399635761261));
#45300=CARTESIAN_POINT('Ctrl Pts',(14.1435753344783,-0.931988786459939,
26.9498556145165));
#45301=CARTESIAN_POINT('Ctrl Pts',(14.1753319409799,-1.03335936072766,26.447357633441));
#45302=CARTESIAN_POINT('Ctrl Pts',(14.2070885474815,-0.88277044582558,25.9627175238428));
#45303=CARTESIAN_POINT('Ctrl Pts',(14.2494306894837,-0.395350283369432,
25.4796478538037));
#45304=CARTESIAN_POINT('Ctrl Pts',(14.2917728314857,0.344725633836522,25.4614507300162));
#45305=CARTESIAN_POINT('Ctrl Pts',(14.3341149734879,0.855298044202682,25.9199815737481));
#45306=CARTESIAN_POINT('Ctrl Pts',(14.3658715799895,1.02952342488545,26.3966350892587));
#45307=CARTESIAN_POINT('Ctrl Pts',(14.3976281864911,0.952971445773425,26.9035078630456));
#45308=CARTESIAN_POINT('Ctrl Pts',(14.4293847929927,0.644120061599205,27.3092851902005));
#45309=CARTESIAN_POINT('Ctrl Pts',(14.4611413994943,0.178259121211541,27.5193561719522));
#45310=CARTESIAN_POINT('Ctrl Pts',(14.4928980059959,-0.330934649491577,
27.4800634437489));
#45311=CARTESIAN_POINT('Ctrl Pts',(14.5246546124975,-0.759717250247051,
27.2026329192894));
#45312=CARTESIAN_POINT('Ctrl Pts',(14.5564112189991,-1.00286953121726,26.7531518836361));
#45313=CARTESIAN_POINT('Ctrl Pts',(14.5881678255007,-1.00251198151107,26.243206505289));
#45314=CARTESIAN_POINT('Ctrl Pts',(14.6199244320022,-0.756120833091242,
25.7936827391846));
#45315=CARTESIAN_POINT('Ctrl Pts',(14.6516810385039,-0.328605271270778,
25.5202170164257));
#45316=CARTESIAN_POINT('Ctrl Pts',(14.6940231805059,0.355421546316196,25.4650623819659));
#45317=CARTESIAN_POINT('Ctrl Pts',(14.7363653225081,0.932974057148912,25.9281785615292));
#45318=CARTESIAN_POINT('Ctrl Pts',(14.7787074645102,1.02777695530517,26.6078454883261));
#45319=CARTESIAN_POINT('Ctrl Pts',(14.8104640710118,0.853745269406024,27.0845697581361));
#45320=CARTESIAN_POINT('Ctrl Pts',(14.8422206775134,0.468504017842465,27.4227551989908));
#45321=CARTESIAN_POINT('Ctrl Pts',(14.873977284015,-0.0291783574561754,
27.5339157587969));
#45322=CARTESIAN_POINT('Ctrl Pts',(14.9057338905166,-0.520756093052546,
27.3942462810327));
#45323=CARTESIAN_POINT('Ctrl Pts',(14.9374904970182,-0.884732141731258,
27.035995460237));
#45324=CARTESIAN_POINT('Ctrl Pts',(14.9692471035198,-1.03373418658115,26.5475073792739));
#45325=CARTESIAN_POINT('Ctrl Pts',(15.0010037100214,-0.929914886747041,
26.0471297357535));
#45326=CARTESIAN_POINT('Ctrl Pts',(15.032760316523,-0.60094740010242,25.6574827038516));
#45327=CARTESIAN_POINT('Ctrl Pts',(15.0645169230246,-0.12282132123504,25.4726160843139));
#45328=CARTESIAN_POINT('Ctrl Pts',(15.0962735295262,0.380301726532211,25.5391010896014));
#45329=CARTESIAN_POINT('Ctrl Pts',(15.1386156715283,0.938823638182425,25.9378340768085));
#45330=CARTESIAN_POINT('Ctrl Pts',(15.1809578135304,1.0818804513813,26.6641798944049));
#45331=CARTESIAN_POINT('Ctrl Pts',(15.2232999555326,0.716270690694064,27.2449244370145));
#45332=CARTESIAN_POINT('Ctrl Pts',(15.2550565620342,0.275934307007477,27.4972276798087));
#45333=CARTESIAN_POINT('Ctrl Pts',(15.2868131685358,-0.236584234701834,
27.5074726159503));
#45334=CARTESIAN_POINT('Ctrl Pts',(15.3185697750374,-0.688736545824772,
27.2716703592064));
#45335=CARTESIAN_POINT('Ctrl Pts',(15.350326381539,-0.974544725908092,26.848031459493));
#45336=CARTESIAN_POINT('Ctrl Pts',(15.3820829880406,-1.02190495790187,26.3395246030613));
#45337=CARTESIAN_POINT('Ctrl Pts',(15.4138395945422,-0.820960657969412,
25.8700103828963));
#45338=CARTESIAN_POINT('Ctrl Pts',(15.4455962010437,-0.419058791443737,
25.5543664017463));
#45339=CARTESIAN_POINT('Ctrl Pts',(15.4773528075454,0.083606239906823,25.4685044020221));
#45340=CARTESIAN_POINT('Ctrl Pts',(15.5091094140469,0.568315349191889,25.6353495208853));
#45341=CARTESIAN_POINT('Ctrl Pts',(15.5408660205486,0.910122788432687,26.0104771413058));
#45342=CARTESIAN_POINT('Ctrl Pts',(15.5832081625506,1.08012910476007,26.675332443826));
#45343=CARTESIAN_POINT('Ctrl Pts',(15.6255503045528,0.721324069998707,27.3228681151001));
#45344=CARTESIAN_POINT('Ctrl Pts',(15.6678924465549,0.0674690680729783,
27.5312148389458));
#45345=CARTESIAN_POINT('Ctrl Pts',(15.6996490530565,-0.431815464948015,
27.4402862284391));
#45346=CARTESIAN_POINT('Ctrl Pts',(15.7314056595581,-0.830263818456473,
27.1177662695237));
#45347=CARTESIAN_POINT('Ctrl Pts',(15.7631622660597,-1.0239653391522,26.6460416277893));
#45348=CARTESIAN_POINT('Ctrl Pts',(15.7949188725613,-0.969415499227341,
26.1379269280244));
#45349=CARTESIAN_POINT('Ctrl Pts',(15.8266754790629,-0.677857750545228,
25.7186223921606));
#45350=CARTESIAN_POINT('Ctrl Pts',(15.8584320855645,-0.221592755694851,
25.4891785666026));
#45351=CARTESIAN_POINT('Ctrl Pts',(15.8901886920661,0.289134130458304,25.5069065364043));
#45352=CARTESIAN_POINT('Ctrl Pts',(15.9219452985677,0.728789294203679,25.7652624028585));
#45353=CARTESIAN_POINT('Ctrl Pts',(15.9537019050693,0.991829552779497,26.2052510807591));
#45354=CARTESIAN_POINT('Ctrl Pts',(15.9854585115709,1.01136259502592,26.7123718921871));
#45355=CARTESIAN_POINT('Ctrl Pts',(16.027800653573,0.712796513379461,27.3302659088038));
#45356=CARTESIAN_POINT('Ctrl Pts',(16.0701427955751,0.0210926696708751,
27.5940637312762));
#45357=CARTESIAN_POINT('Ctrl Pts',(16.1124849375773,-0.613104067421575,
27.3319011490073));
#45358=CARTESIAN_POINT('Ctrl Pts',(16.1442415440789,-0.936221230599484,
26.940559410903));
#45359=CARTESIAN_POINT('Ctrl Pts',(16.1759981505805,-1.03296812494877,26.4371507769423));
#45360=CARTESIAN_POINT('Ctrl Pts',(16.207754757082,-0.877003865383148,25.9516411823127));
#45361=CARTESIAN_POINT('Ctrl Pts',(16.2395113635837,-0.507783790844506,
25.5983243702152));
#45362=CARTESIAN_POINT('Ctrl Pts',(16.2712679700852,-0.0146040258474385,
25.4656747037629));
#45363=CARTESIAN_POINT('Ctrl Pts',(16.3030245765869,0.482124254864565,25.5843474881466));
#45364=CARTESIAN_POINT('Ctrl Pts',(16.3347811830884,0.861172381629166,25.9270992215475));
#45365=CARTESIAN_POINT('Ctrl Pts',(16.3665377895901,1.03078191910565,26.4080119179241));
#45366=CARTESIAN_POINT('Ctrl Pts',(16.3982943960916,0.948286387643184,26.9139513427579));
#45367=CARTESIAN_POINT('Ctrl Pts',(16.4300510025932,0.636346828133913,27.3142596843346));
#45368=CARTESIAN_POINT('Ctrl Pts',(16.4723931445954,0.00980457101295316,
27.5942231121645));
#45369=CARTESIAN_POINT('Ctrl Pts',(16.5147352865975,-0.689071371571145,
27.3500594059764));
#45370=CARTESIAN_POINT('Ctrl Pts',(16.5570774285996,-1.00496351044611,26.7408411548729));
#45371=CARTESIAN_POINT('Ctrl Pts',(16.5888340351012,-0.999755857372427,
26.2333710203111));
#45372=CARTESIAN_POINT('Ctrl Pts',(16.6205906416028,-0.749242708650261,
25.7861312897083));
#45373=CARTESIAN_POINT('Ctrl Pts',(16.6523472481044,-0.317056998530502,
25.5154655757592));
#45374=CARTESIAN_POINT('Ctrl Pts',(16.684103854606,0.192965778634376,25.4833252595505));
#45375=CARTESIAN_POINT('Ctrl Pts',(16.7158604611076,0.655526805774623,25.6997958367279));
#45376=CARTESIAN_POINT('Ctrl Pts',(16.7476170676092,0.958806604837357,26.1107016386983));
#45377=CARTESIAN_POINT('Ctrl Pts',(16.7793736741108,1.02768036254931,26.6170736745095));
#45378=CARTESIAN_POINT('Ctrl Pts',(16.8111302806124,0.84737431619961,27.0940790690171));
#45379=CARTESIAN_POINT('Ctrl Pts',(16.842886887114,0.45819054239387,27.4277199006279));
#45380=CARTESIAN_POINT('Ctrl Pts',(16.8746434936156,-0.03832776048991,27.5327086239523));
#45381=CARTESIAN_POINT('Ctrl Pts',(16.9169856356177,-0.697804391611141,
27.3429053208116));
#45382=CARTESIAN_POINT('Ctrl Pts',(16.9593277776199,-1.07474834669968,26.705757964806));
#45383=CARTESIAN_POINT('Ctrl Pts',(17.001669919622,-0.923580740087578,26.036367887498));
#45384=CARTESIAN_POINT('Ctrl Pts',(17.0334265261236,-0.592500579978268,
25.6517395153092));
#45385=CARTESIAN_POINT('Ctrl Pts',(17.0651831326252,-0.112695250427537,
25.471276056202));
#45386=CARTESIAN_POINT('Ctrl Pts',(17.0969397391268,0.392193553644114,25.5429120263731));
#45387=CARTESIAN_POINT('Ctrl Pts',(17.1286963456284,0.802846822853741,25.8470832375036));
#45388=CARTESIAN_POINT('Ctrl Pts',(17.1604529521299,1.01696687064652,26.3107370089288));
#45389=CARTESIAN_POINT('Ctrl Pts',(17.1922095586316,0.983982253354352,26.8203782841956));
#45390=CARTESIAN_POINT('Ctrl Pts',(17.2239661651331,0.710248653396368,27.2519175639406));
#45391=CARTESIAN_POINT('Ctrl Pts',(17.2557227716348,0.264934019955137,27.5003914917165));
#45392=CARTESIAN_POINT('Ctrl Pts',(17.2874793781363,-0.247669462891774,
27.5046206380023));
#45393=CARTESIAN_POINT('Ctrl Pts',(17.319235984638,-0.694953617707919,27.2648500398476));
#45394=CARTESIAN_POINT('Ctrl Pts',(17.36157812664,-1.07681387153837,26.6946593098991));
#45395=CARTESIAN_POINT('Ctrl Pts',(17.4039202686422,-0.954321079185971,
25.9645640902068));
#45396=CARTESIAN_POINT('Ctrl Pts',(17.4462624106443,-0.407279311502855,
25.5502212472916));
#45397=CARTESIAN_POINT('Ctrl Pts',(17.4780190171459,0.093766132664254,25.469557991685));
#45398=CARTESIAN_POINT('Ctrl Pts',(17.5097756236475,0.576920900887735,25.6408519665439));
#45399=CARTESIAN_POINT('Ctrl Pts',(17.5415322301491,0.916758344639924,26.0210558161049));
#45400=CARTESIAN_POINT('Ctrl Pts',(17.5732888366507,1.03466320862596,26.5183029959961));
#45401=CARTESIAN_POINT('Ctrl Pts',(17.6050454431523,0.89951261763213,27.0108028643862));
#45402=CARTESIAN_POINT('Ctrl Pts',(17.6368020496539,0.545795229668867,27.3791875771826));
#45403=CARTESIAN_POINT('Ctrl Pts',(17.6685586561555,0.0583585912529178,
27.5326791628602));
#45404=CARTESIAN_POINT('Ctrl Pts',(17.7003152626571,-0.442267253439534,
27.4356159037157));
#45405=CARTESIAN_POINT('Ctrl Pts',(17.7320718691587,-0.836896502722454,
27.1084383526819));
#45406=CARTESIAN_POINT('Ctrl Pts',(17.7638284756603,-1.02432995541793,26.6368239035113));
#45407=CARTESIAN_POINT('Ctrl Pts',(17.8061706176624,-0.948729406006919,
25.9547380886554));
#45408=CARTESIAN_POINT('Ctrl Pts',(17.8485127596645,-0.384532327064874,
25.4755273691514));
#45409=CARTESIAN_POINT('Ctrl Pts',(17.8908549016667,0.300852282996595,25.5113082876285));
#45410=CARTESIAN_POINT('Ctrl Pts',(17.9226115081683,0.735793104159824,25.7726623671022));
#45411=CARTESIAN_POINT('Ctrl Pts',(17.9543681146699,0.99502713087998,26.2149159219124));
#45412=CARTESIAN_POINT('Ctrl Pts',(17.9861247211715,1.00930328775722,26.7249060355728));
#45413=CARTESIAN_POINT('Ctrl Pts',(18.0178813276731,0.779844466238091,27.180583963405));
#45414=CARTESIAN_POINT('Ctrl Pts',(18.0496379341747,0.35736334799373,27.4709289170012));
#45415=CARTESIAN_POINT('Ctrl Pts',(18.0813945406763,-0.147393818954905,
27.5228873156073));
#45416=CARTESIAN_POINT('Ctrl Pts',(18.1237366826784,-0.783125367432545,
27.2642800146539));
#45417=CARTESIAN_POINT('Ctrl Pts',(18.1660788246805,-1.09047816706153,26.5908592590081));
#45418=CARTESIAN_POINT('Ctrl Pts',(18.2084209666827,-0.86932372855012,25.9412076475843));
#45419=CARTESIAN_POINT('Ctrl Pts',(18.2401775731842,-0.499383898262576,
25.5937943349109));
#45420=CARTESIAN_POINT('Ctrl Pts',(18.2719341796858,-0.00317682288826529,
25.46512447582));
#45421=CARTESIAN_POINT('Ctrl Pts',(18.3036907861874,0.491295670994858,25.5898019214257));
#45422=CARTESIAN_POINT('Ctrl Pts',(18.335447392689,0.867445371041332,25.9357290040588));
#45423=CARTESIAN_POINT('Ctrl Pts',(18.3672039991906,1.03128709694628,26.4194429443397));
#45424=CARTESIAN_POINT('Ctrl Pts',(18.3989606056922,0.944543650636288,26.9227295198934));
#45425=CARTESIAN_POINT('Ctrl Pts',(18.4307172121938,0.626670994684664,27.3228711066594));
#45426=CARTESIAN_POINT('Ctrl Pts',(18.4624738186954,0.157557720092282,27.5228140760235));
#45427=CARTESIAN_POINT('Ctrl Pts',(18.494230425197,-0.352613787923266,27.4727622200216));
#45428=CARTESIAN_POINT('Ctrl Pts',(18.5259870316986,-0.772006450303902,
27.1869950198973));
#45429=CARTESIAN_POINT('Ctrl Pts',(18.5683291737007,-1.09136884806166,26.5795887753102));
#45430=CARTESIAN_POINT('Ctrl Pts',(18.6106713157029,-0.892286124579294,
25.8665603164065));
#45431=CARTESIAN_POINT('Ctrl Pts',(18.653013457705,-0.304460587344251,25.5124475381155));
#45432=CARTESIAN_POINT('Ctrl Pts',(18.6847700642066,0.202308107498574,25.4852713570665));
#45433=CARTESIAN_POINT('Ctrl Pts',(18.7165266707082,0.66461794473409,25.7067433207557));
#45434=CARTESIAN_POINT('Ctrl Pts',(18.7482832772098,0.962302924353875,26.1207820489563));
#45435=CARTESIAN_POINT('Ctrl Pts',(18.7800398837114,1.02691384051011,26.6277156375282));
#45436=CARTESIAN_POINT('Ctrl Pts',(18.811796490213,0.840392506564997,27.1031438722984));
#45437=CARTESIAN_POINT('Ctrl Pts',(18.8435530967146,0.449670903237747,27.4320189904163));
#45438=CARTESIAN_POINT('Ctrl Pts',(18.8753097032162,-0.0512760300646483,
27.5330556333141));
#45439=CARTESIAN_POINT('Ctrl Pts',(18.9070663097177,-0.53881215429493,27.38354662265));
#45440=CARTESIAN_POINT('Ctrl Pts',(18.9388229162194,-0.896600742236581,
27.0164396345976));
#45441=CARTESIAN_POINT('Ctrl Pts',(18.970579522721,-1.03305018659491,26.5276302584141));
#45442=CARTESIAN_POINT('Ctrl Pts',(19.0129216647231,-0.885703716579554,
25.8573887059411));
#45443=CARTESIAN_POINT('Ctrl Pts',(19.0552638067252,-0.27390066770943,25.4405667680158));
#45444=CARTESIAN_POINT('Ctrl Pts',(19.0976059487273,0.403769437737008,25.5487238254014));
#45445=CARTESIAN_POINT('Ctrl Pts',(19.1293625552289,0.80873508663663,25.8545928829001));
#45446=CARTESIAN_POINT('Ctrl Pts',(19.1611191617305,1.01943935782009,26.3219085411192));
#45447=CARTESIAN_POINT('Ctrl Pts',(19.1928757682321,0.980157852742228,26.8303388510914));
#45448=CARTESIAN_POINT('Ctrl Pts',(19.2246323747337,0.702803149690609,27.259559775381));
#45449=CARTESIAN_POINT('Ctrl Pts',(19.2563889812353,0.253753217819898,27.5028217191771));
#45450=CARTESIAN_POINT('Ctrl Pts',(19.2881455877369,-0.25695418374839,27.5024160149589));
#45451=CARTESIAN_POINT('Ctrl Pts',(19.3199021942385,-0.70507685881597,27.2567693149135));
#45452=CARTESIAN_POINT('Ctrl Pts',(19.3516588007401,-0.981452793478104,
26.8282127148256));
#45453=CARTESIAN_POINT('Ctrl Pts',(19.3834154072417,-1.01837402149756,26.316923132266));
#45454=CARTESIAN_POINT('Ctrl Pts',(19.4151720137433,-0.807625565040175,
25.8552542625948));
#45455=CARTESIAN_POINT('Ctrl Pts',(19.4575141557454,-0.262956383022123,
25.4377974348384));
#45456=CARTESIAN_POINT('Ctrl Pts',(19.4998562977476,0.473465944610788,25.5134654856004));
#45457=CARTESIAN_POINT('Ctrl Pts',(19.5421984397497,0.921862468895972,26.0329607001015));
#45458=CARTESIAN_POINT('Ctrl Pts',(19.5739550462513,1.03432477236453,26.5278397635314));
#45459=CARTESIAN_POINT('Ctrl Pts',(19.6057116527529,0.894201810927097,27.0209378977708));
#45460=CARTESIAN_POINT('Ctrl Pts',(19.6374682592545,0.536451672577482,27.3843374784669));
#45461=CARTESIAN_POINT('Ctrl Pts',(19.6692248657561,0.0477390316638463,
27.5337235145085));
#45462=CARTESIAN_POINT('Ctrl Pts',(19.7009814722577,-0.452379697582753,
27.4302659325279));
#45463=CARTESIAN_POINT('Ctrl Pts',(19.7327380787593,-0.842578293657814,
27.1007704542076));
#45464=CARTESIAN_POINT('Ctrl Pts',(19.7644946852609,-1.02685355954554,26.6241166390178));
#45465=CARTESIAN_POINT('Ctrl Pts',(19.7962512917624,-0.961922530439277,
26.118321840509));
#45466=CARTESIAN_POINT('Ctrl Pts',(19.8280078982641,-0.660590012392387,
25.7036184189173));
#45467=CARTESIAN_POINT('Ctrl Pts',(19.8597645047656,-0.201886130050825,
25.4864921758063));
#45468=CARTESIAN_POINT('Ctrl Pts',(19.9021066467678,0.483618392455461,25.518402526854));
#45469=CARTESIAN_POINT('Ctrl Pts',(19.9444487887699,0.997875136828353,26.0509281125392));
#45470=CARTESIAN_POINT('Ctrl Pts',(19.9867909307721,1.00584597201986,26.7371286565982));
#45471=CARTESIAN_POINT('Ctrl Pts',(20.0185475372736,0.772845883424032,27.1879767638772));
#45472=CARTESIAN_POINT('Ctrl Pts',(20.0503041437752,0.34788027460314,27.474655060286));
#45473=CARTESIAN_POINT('Ctrl Pts',(20.0820607502768,-0.159872213864887,
27.5218972786275));
#45474=CARTESIAN_POINT('Ctrl Pts',(20.1138173567784,-0.629805628964096,
27.3211018142211));
#45475=CARTESIAN_POINT('Ctrl Pts',(20.14557396328,-0.945484809342076,26.9196433858772));
#45476=CARTESIAN_POINT('Ctrl Pts',(20.1773305697816,-1.03142817993489,26.4162191595395));
#45477=CARTESIAN_POINT('Ctrl Pts',(20.2090871762832,-0.865079916123635,
25.9330168330965));
#45478=CARTESIAN_POINT('Ctrl Pts',(20.2408437827848,-0.489418261207368,
25.5881650710814));
#45479=CARTESIAN_POINT('Ctrl Pts',(20.2726003892864,0.00826905202714611,
25.465333672173));
#45480=CARTESIAN_POINT('Ctrl Pts',(20.304356995788,0.49892246719443,25.5949958613701));
#45481=CARTESIAN_POINT('Ctrl Pts',(20.3466991377902,1.00245491067529,26.061246651442));
#45482=CARTESIAN_POINT('Ctrl Pts',(20.3890412797922,1.05238006533853,26.7998608792188));
#45483=CARTESIAN_POINT('Ctrl Pts',(20.4313834217944,0.616171706309765,27.3296315733818));
#45484=CARTESIAN_POINT('Ctrl Pts',(20.463140028296,0.14743010257547,27.5241421542027));
#45485=CARTESIAN_POINT('Ctrl Pts',(20.4948966347976,-0.362259777948479,
27.4694024062689));
#45486=CARTESIAN_POINT('Ctrl Pts',(20.5266532412992,-0.780911495880461,
27.1782406714686));
#45487=CARTESIAN_POINT('Ctrl Pts',(20.5584098478008,-1.01077175041952,26.7218192691043));
#45488=CARTESIAN_POINT('Ctrl Pts',(20.5901664543024,-0.993356517859664,
26.2114087242608));
#45489=CARTESIAN_POINT('Ctrl Pts',(20.6219230608039,-0.734573511031013,
25.7711206708353));
#45490=CARTESIAN_POINT('Ctrl Pts',(20.6536796673056,-0.295935925419432,
25.5089121628844));
#45491=CARTESIAN_POINT('Ctrl Pts',(20.6854362738071,0.213555451735285,25.4873958122577));
#45492=CARTESIAN_POINT('Ctrl Pts',(20.7171928803088,0.67323417955922,25.7142783402288));
#45493=CARTESIAN_POINT('Ctrl Pts',(20.7489494868103,0.964786043823933,26.1296704051102));
#45494=CARTESIAN_POINT('Ctrl Pts',(20.7912916288125,1.04923052736995,26.8107018655283));
#45495=CARTESIAN_POINT('Ctrl Pts',(20.8336337708146,0.611314093750934,27.4075876969138));
#45496=CARTESIAN_POINT('Ctrl Pts',(20.8759759128168,-0.0636608179687255,
27.5314569401891));
#45497=CARTESIAN_POINT('Ctrl Pts',(20.9077325193183,-0.547411231874149,
27.378034014363));
#45498=CARTESIAN_POINT('Ctrl Pts',(20.9394891258199,-0.901809936088342,
27.0076534360875));
#45499=CARTESIAN_POINT('Ctrl Pts',(20.9712457323215,-1.03421574978554,26.51519722764));
#45500=CARTESIAN_POINT('Ctrl Pts',(21.0030023388231,-0.915760529993523,
26.0180809494344));
#45501=CARTESIAN_POINT('Ctrl Pts',(21.0347589453247,-0.57345180235752,25.6390731004435));
#45502=CARTESIAN_POINT('Ctrl Pts',(21.0665155518263,-0.0918045968468163,
25.4692550094277));
#45503=CARTESIAN_POINT('Ctrl Pts',(21.0982721583279,0.412565734402345,25.5515155838763));
#45504=CARTESIAN_POINT('Ctrl Pts',(21.1300287648295,0.815964861986395,25.8634667989785));
#45505=CARTESIAN_POINT('Ctrl Pts',(21.1617853713311,1.02117005185408,26.3332231660069));
#45506=CARTESIAN_POINT('Ctrl Pts',(21.1935419778327,0.976327171856112,26.838734959377));
#45507=CARTESIAN_POINT('Ctrl Pts',(21.2358841198349,0.60191837674119,27.4138460573581));
#45508=CARTESIAN_POINT('Ctrl Pts',(21.2782262618369,-0.117622662984219,
27.5879270462491));
#45509=CARTESIAN_POINT('Ctrl Pts',(21.3205684038391,-0.713515152902132,
27.2475642084716));
#45510=CARTESIAN_POINT('Ctrl Pts',(21.3523250103406,-0.984473950176901,
26.8184553792661));
#45511=CARTESIAN_POINT('Ctrl Pts',(21.3840816168423,-1.01669340159119,26.3068479895003));
#45512=CARTESIAN_POINT('Ctrl Pts',(21.4158382233439,-0.800502768285593,
25.844997335273));
#45513=CARTESIAN_POINT('Ctrl Pts',(21.4475948298455,-0.389513214291506,
25.541280658647));
#45514=CARTESIAN_POINT('Ctrl Pts',(21.4793514363471,0.116494160805104,25.472152148173));
#45515=CARTESIAN_POINT('Ctrl Pts',(21.5111080428486,0.594195549276261,25.6527721860017));
#45516=CARTESIAN_POINT('Ctrl Pts',(21.5428646493503,0.926788179821187,26.040764937558));
#45517=CARTESIAN_POINT('Ctrl Pts',(21.5746212558519,1.03413244324324,26.5392843713313));
#45518=CARTESIAN_POINT('Ctrl Pts',(21.6063778623534,0.88823197146014,27.0307040154704));
#45519=CARTESIAN_POINT('Ctrl Pts',(21.6381344688551,0.528111077870776,27.3882875709132));
#45520=CARTESIAN_POINT('Ctrl Pts',(21.6804766108571,-0.128840070118087,
27.5866556884035));
#45521=CARTESIAN_POINT('Ctrl Pts',(21.7228187528594,-0.791170334647484,
27.2559562489864));
#45522=CARTESIAN_POINT('Ctrl Pts',(21.7651608948614,-1.0273717259971,26.6116398487566));
#45523=CARTESIAN_POINT('Ctrl Pts',(21.7969175013631,-0.957943088858718,
26.1089145545175));
#45524=CARTESIAN_POINT('Ctrl Pts',(21.8286741078646,-0.65281099082484,25.6969987657186));
#45525=CARTESIAN_POINT('Ctrl Pts',(21.8604307143662,-0.1898291330484,25.4832413889823));
#45526=CARTESIAN_POINT('Ctrl Pts',(21.8921873208678,0.320157771778428,25.5159459767056));
#45527=CARTESIAN_POINT('Ctrl Pts',(21.9239439273694,0.751582456070183,25.7892497571336));
#45528=CARTESIAN_POINT('Ctrl Pts',(21.955700533871,1.00038611624865,26.2352530679894));
#45529=CARTESIAN_POINT('Ctrl Pts',(21.9874571403726,1.00458155593204,26.7462703195953));
#45530=CARTESIAN_POINT('Ctrl Pts',(22.0192137468742,0.765322018551718,27.1966027418257));
#45531=CARTESIAN_POINT('Ctrl Pts',(22.0509703533758,0.337021128126196,27.4782737583913));
#45532=CARTESIAN_POINT('Ctrl Pts',(22.0827269598774,-0.168795095708431,
27.5195412374561));
#45533=CARTESIAN_POINT('Ctrl Pts',(22.1250691018795,-0.798927100233512,
27.2477538614546));
#45534=CARTESIAN_POINT('Ctrl Pts',(22.1674112438817,-1.09215204104248,26.5680019709608));
#45535=CARTESIAN_POINT('Ctrl Pts',(22.2097533858837,-0.857433947833973,
25.9231437403386));
#45536=CARTESIAN_POINT('Ctrl Pts',(22.2415099923854,-0.480312159776085,
25.5835377714648));
#45537=CARTESIAN_POINT('Ctrl Pts',(22.2732665988869,0.0184832960993065,
25.4652867354845));
#45538=CARTESIAN_POINT('Ctrl Pts',(22.3050232053886,0.510235965813027,25.6002820263975));
#45539=CARTESIAN_POINT('Ctrl Pts',(22.3367798118902,0.879064903268412,25.9540071287703));
#45540=CARTESIAN_POINT('Ctrl Pts',(22.3685364183917,1.03274691096626,26.4410431183259));
#45541=CARTESIAN_POINT('Ctrl Pts',(22.4002930248934,0.935489987070818,26.9424045701417));
#45542=CARTESIAN_POINT('Ctrl Pts',(22.4320496313949,0.609312582905039,27.3358058082749));
#45543=CARTESIAN_POINT('Ctrl Pts',(22.4638062378966,0.136117726577721,27.525887487257));
#45544=CARTESIAN_POINT('Ctrl Pts',(22.4955628443981,-0.372894606452285,
27.4651696222111));
#45545=CARTESIAN_POINT('Ctrl Pts',(22.5273194508997,-0.7862148363273,27.170687967946));
#45546=CARTESIAN_POINT('Ctrl Pts',(22.5696615929019,-1.09279546637427,26.5567310979945));
#45547=CARTESIAN_POINT('Ctrl Pts',(22.612003734904,-0.878834030206561,25.8480252334954));
#45548=CARTESIAN_POINT('Ctrl Pts',(22.6543458769061,-0.28372634610829,25.5062920551124));
#45549=CARTESIAN_POINT('Ctrl Pts',(22.6861024834077,0.223500105487194,25.4897275169502));
#45550=CARTESIAN_POINT('Ctrl Pts',(22.7178590899093,0.681073708837323,25.7208262227656));
#45551=CARTESIAN_POINT('Ctrl Pts',(22.7496156964109,0.970028462438422,26.1410042411229));
#45552=CARTESIAN_POINT('Ctrl Pts',(22.7813723029125,1.024016088893,26.6491789840438));
#45553=CARTESIAN_POINT('Ctrl Pts',(22.8131289094141,0.827585813813665,27.1205995623439));
#45554=CARTESIAN_POINT('Ctrl Pts',(22.8448855159157,0.430067065154834,27.4412256047629));
#45555=CARTESIAN_POINT('Ctrl Pts',(22.8766421224173,-0.0728846540605334,
27.5317562696853));
#45556=CARTESIAN_POINT('Ctrl Pts',(22.9083987289189,-0.557185066024646,
27.3720768166843));
#45557=CARTESIAN_POINT('Ctrl Pts',(22.9401553354205,-0.907212454062326,
26.9975624085023));
#45558=CARTESIAN_POINT('Ctrl Pts',(22.9719119419221,-1.03340217998071,26.5060044666528));
#45559=CARTESIAN_POINT('Ctrl Pts',(23.0142540839242,-0.872061123160507,
25.8389933840877));
#45560=CARTESIAN_POINT('Ctrl Pts',(23.0565962259264,-0.251668792754912,
25.4350665900813));
#45561=CARTESIAN_POINT('Ctrl Pts',(23.0989383679284,0.423589374350715,25.5573822826056));
#45562=CARTESIAN_POINT('Ctrl Pts',(23.1306949744301,0.822065082155542,25.8716594968801));
#45563=CARTESIAN_POINT('Ctrl Pts',(23.1624515809316,1.02294319380588,26.3432824379804));
#45564=CARTESIAN_POINT('Ctrl Pts',(23.1942081874333,0.973029829999189,26.8507793077765));
#45565=CARTESIAN_POINT('Ctrl Pts',(23.2259647939348,0.68675310912089,27.2741017289122));
#45566=CARTESIAN_POINT('Ctrl Pts',(23.2577214004365,0.232710524832593,27.5079126488139));
#45567=CARTESIAN_POINT('Ctrl Pts',(23.2894780069381,-0.27787653308415,27.49681891633));
#45568=CARTESIAN_POINT('Ctrl Pts',(23.3212346134396,-0.720760152325672,
27.2418476768528));
#45569=CARTESIAN_POINT('Ctrl Pts',(23.3529912199413,-0.98810669635931,26.8076009242656));
#45570=CARTESIAN_POINT('Ctrl Pts',(23.3847478264428,-1.01431953699964,26.2956506324423));
#45571=CARTESIAN_POINT('Ctrl Pts',(23.4165044329445,-0.793955402214,25.8384934327583));
#45572=CARTESIAN_POINT('Ctrl Pts',(23.4588465749466,-0.240668948257476,
25.4325269061225));
#45573=CARTESIAN_POINT('Ctrl Pts',(23.5011887169487,0.494008505367471,25.5235902778892));
#45574=CARTESIAN_POINT('Ctrl Pts',(23.5435308589508,0.931434794646534,26.0523557857735));
#45575=CARTESIAN_POINT('Ctrl Pts',(23.5752874654524,1.03351560643094,26.5494800810842));
#45576=CARTESIAN_POINT('Ctrl Pts',(23.607044071954,0.883103744901561,27.0395377166982));
#45577=CARTESIAN_POINT('Ctrl Pts',(23.6388006784556,0.517826709887917,27.3953706893567));
#45578=CARTESIAN_POINT('Ctrl Pts',(23.6705572849572,0.026094744315042,27.5344961981135));
#45579=CARTESIAN_POINT('Ctrl Pts',(23.7023138914588,-0.471749284087486,
27.4205947582786));
#45580=CARTESIAN_POINT('Ctrl Pts',(23.7340704979604,-0.854966718043896,
27.0830053435684));
#45581=CARTESIAN_POINT('Ctrl Pts',(23.765827104462,-1.02922618322529,26.6025993986139));
#45582=CARTESIAN_POINT('Ctrl Pts',(23.7975837109636,-0.953724069196557,
26.0982742579392));
#45583=CARTESIAN_POINT('Ctrl Pts',(23.8293403174652,-0.643778608069701,
25.6899679691813));
#45584=CARTESIAN_POINT('Ctrl Pts',(23.8610969239668,-0.180631157292743,
25.4824890643223));
#45585=CARTESIAN_POINT('Ctrl Pts',(23.9034390659689,0.504055406949821,25.5287387089293));
#45586=CARTESIAN_POINT('Ctrl Pts',(23.945781207971,1.00705479143988,26.0719100610318));
#45587=CARTESIAN_POINT('Ctrl Pts',(23.9881233499732,1.0006630320742,26.7581271304004));
#45588=CARTESIAN_POINT('Ctrl Pts',(24.0198799564748,0.758278596218176,27.2040002540325));
#45589=CARTESIAN_POINT('Ctrl Pts',(24.0516365629764,0.327406439929028,27.4817220559263));
#45590=CARTESIAN_POINT('Ctrl Pts',(24.083393169478,-0.181223530827346,27.5183276509586));
#45591=CARTESIAN_POINT('Ctrl Pts',(24.1151497759796,-0.646851762725688,
27.3077413674257));
#45592=CARTESIAN_POINT('Ctrl Pts',(24.1469063824811,-0.954060056708101,
26.8997643108148));
#45593=CARTESIAN_POINT('Ctrl Pts',(24.1786629889828,-1.02944890996991,26.3946517140441));
#45594=CARTESIAN_POINT('Ctrl Pts',(24.2104195954843,-0.853024589922902,
25.9150365636903));
#45595=CARTESIAN_POINT('Ctrl Pts',(24.2421762019859,-0.47022813118385,25.5781222008084));
#45596=CARTESIAN_POINT('Ctrl Pts',(24.2739328084876,0.029920803971738,25.4657333358122));
#45597=CARTESIAN_POINT('Ctrl Pts',(24.3056894149891,0.517753179655688,25.6056355529399));
#45598=CARTESIAN_POINT('Ctrl Pts',(24.3480315569913,1.01141761520222,26.0823221858101));
#45599=CARTESIAN_POINT('Ctrl Pts',(24.3903736989933,1.04587406972389,26.8218194821433));
#45600=CARTESIAN_POINT('Ctrl Pts',(24.4327158409956,0.598674172340223,27.3423451516935));
#45601=CARTESIAN_POINT('Ctrl Pts',(24.4644724474971,0.12596450061625,27.5270032773778));
#45602=CARTESIAN_POINT('Ctrl Pts',(24.4962290539988,-0.382468152772,27.4616086959436));
#45603=CARTESIAN_POINT('Ctrl Pts',(24.5279856605003,-0.794934727931843,
27.1617491603019));
#45604=CARTESIAN_POINT('Ctrl Pts',(24.5597422670019,-1.01519262315461,26.7006171913983));
#45605=CARTESIAN_POINT('Ctrl Pts',(24.5914988735035,-0.987099300322622,
26.1906829016855));
#45606=CARTESIAN_POINT('Ctrl Pts',(24.6232554800051,-0.719158594584726,
25.7559071056468));
#45607=CARTESIAN_POINT('Ctrl Pts',(24.6550120865067,-0.275129561181238,
25.5029358609414));
#45608=CARTESIAN_POINT('Ctrl Pts',(24.6867686930083,0.234700524814755,25.492086890823));
#45609=CARTESIAN_POINT('Ctrl Pts',(24.7185252995099,0.68953036364492,25.7285399136883));
#45610=CARTESIAN_POINT('Ctrl Pts',(24.7502819060115,0.972325021744744,26.1499426171358));
#45611=CARTESIAN_POINT('Ctrl Pts',(24.7926240480136,1.04249834070029,26.8325921803725));
#45612=CARTESIAN_POINT('Ctrl Pts',(24.8349661900157,0.59218615294308,27.4201825411679));
#45613=CARTESIAN_POINT('Ctrl Pts',(24.8773083320179,-0.0852332719656635,
27.5298987370411));
#45614=CARTESIAN_POINT('Ctrl Pts',(24.9090649385194,-0.56566689204097,27.3663854537151));
#45615=CARTESIAN_POINT('Ctrl Pts',(24.9408215450211,-0.912236628899084,
26.9886691159609));
#45616=CARTESIAN_POINT('Ctrl Pts',(24.9725781515226,-1.03430728862988,26.4935497659328));
#45617=CARTESIAN_POINT('Ctrl Pts',(25.0043347580243,-0.905474331192122,
25.9990214025088));
#45618=CARTESIAN_POINT('Ctrl Pts',(25.0360913645258,-0.555308674141558,
25.627260421185));
#45619=CARTESIAN_POINT('Ctrl Pts',(25.0678479710275,-0.0702129931772203,
25.4675594665158));
#45620=CARTESIAN_POINT('Ctrl Pts',(25.099604577529,0.432325318386934,25.5603575190988));
#45621=CARTESIAN_POINT('Ctrl Pts',(25.1313611840307,0.82910756018719,25.8806827746304));
#45622=CARTESIAN_POINT('Ctrl Pts',(25.1631177905322,1.02443671559781,26.3546308048603));
#45623=CARTESIAN_POINT('Ctrl Pts',(25.1948743970339,0.969024273802758,26.8590934084466));
#45624=CARTESIAN_POINT('Ctrl Pts',(25.2372165390359,0.582661518377644,27.426242896766));
#45625=CARTESIAN_POINT('Ctrl Pts',(25.2795586810381,-0.140365108464849,
27.5852271583099));
#45626=CARTESIAN_POINT('Ctrl Pts',(25.3219008230402,-0.729003953235837,
27.2324679893181));
#45627=CARTESIAN_POINT('Ctrl Pts',(25.3536574295418,-0.990922989234294,
26.7977824987574));
#45628=CARTESIAN_POINT('Ctrl Pts',(25.3854140360434,-1.01242843194554,26.285612868414));
#45629=CARTESIAN_POINT('Ctrl Pts',(25.417170642545,-0.786619507832964,25.8283878182122));
#45630=CARTESIAN_POINT('Ctrl Pts',(25.4489272490466,-0.369363765088924,
25.5333388760098));
#45631=CARTESIAN_POINT('Ctrl Pts',(25.4806838555482,0.137979512235093,25.4748152604466));
#45632=CARTESIAN_POINT('Ctrl Pts',(25.5124404620498,0.611796248789613,25.6653931047851));
#45633=CARTESIAN_POINT('Ctrl Pts',(25.5441970685514,0.936196099210013,26.0602613995694));
#45634=CARTESIAN_POINT('Ctrl Pts',(25.575953675053,1.03308380589826,26.560918157259));
#45635=CARTESIAN_POINT('Ctrl Pts',(25.6077102815546,0.876930827085415,27.0491767582768));
#45636=CARTESIAN_POINT('Ctrl Pts',(25.6394668880562,0.509405273945525,27.3991453641787));
#45637=CARTESIAN_POINT('Ctrl Pts',(25.6818090300583,-0.151553451361267,
27.5837213202816));
#45638=CARTESIAN_POINT('Ctrl Pts',(25.7241511720605,-0.806817757172094,
27.2392330192721));
#45639=CARTESIAN_POINT('Ctrl Pts',(25.7664933140625,-1.02948312020622,26.5901144967068));
#45640=CARTESIAN_POINT('Ctrl Pts',(25.7982499205642,-0.949548624829341,
26.0889523143866));
#45641=CARTESIAN_POINT('Ctrl Pts',(25.8300065270657,-0.635862749944225,
25.6835125654851));
#45642=CARTESIAN_POINT('Ctrl Pts',(25.8617631335674,-0.168508775453428,
25.4794913193942));
#45643=CARTESIAN_POINT('Ctrl Pts',(25.8935197400689,0.340682011144958,25.5228617818911));
#45644=CARTESIAN_POINT('Ctrl Pts',(25.9252763465706,0.766292448421236,25.8051345895338));
#45645=CARTESIAN_POINT('Ctrl Pts',(25.9570329530721,1.00570770483935,26.2562471941713));
#45646=CARTESIAN_POINT('Ctrl Pts',(25.9887895595738,0.999207484337658,26.7672403335045));
#45647=CARTESIAN_POINT('Ctrl Pts',(26.0205461660753,0.750576026028524,27.2124668751901));
#45648=CARTESIAN_POINT('Ctrl Pts',(26.0523027725769,0.316473618880258,27.4851127148182));
#45649=CARTESIAN_POINT('Ctrl Pts',(26.0840593790785,-0.190094577903723,
27.5157853616777));
#45650=CARTESIAN_POINT('Ctrl Pts',(26.1264015210806,-0.814402461431545,
27.2308701517941));
#45651=CARTESIAN_POINT('Ctrl Pts',(26.1687436630828,-1.0933334814934,26.545130338164));
#45652=CARTESIAN_POINT('Ctrl Pts',(26.2110858050849,-0.845176745039968,
25.9053257852602));
#45653=CARTESIAN_POINT('Ctrl Pts',(26.2428424115865,-0.461020723843732,
25.5736862003506));
#45654=CARTESIAN_POINT('Ctrl Pts',(26.2745990180881,0.0401212288996642,
25.4659007339855));
#45655=CARTESIAN_POINT('Ctrl Pts',(26.3063556245897,0.52897749149536,25.6111562525088));
#45656=CARTESIAN_POINT('Ctrl Pts',(26.3381122310913,0.890253680816816,25.9725259631335));
#45657=CARTESIAN_POINT('Ctrl Pts',(26.3698688375929,1.03384007386217,26.4626646873927));
#45658=CARTESIAN_POINT('Ctrl Pts',(26.4016254440945,0.925865194744989,26.9619004416844));
#45659=CARTESIAN_POINT('Ctrl Pts',(26.4227965150956,0.70328308920618,27.219502667261));
#45660=CARTESIAN_POINT('Ctrl Pts',(26.4333820505961,0.567943631320456,27.313938745633));
#45661=CARTESIAN_POINT('Ctrl Pts',(9.55924492783123,0.793913214729588,26.042198285305));
#45662=CARTESIAN_POINT('Ctrl Pts',(9.56983046333176,0.870035203292496,26.1742079539272));
#45663=CARTESIAN_POINT('Ctrl Pts',(9.59100153433282,0.955123975386584,26.4768302220545));
#45664=CARTESIAN_POINT('Ctrl Pts',(9.62275814083443,0.849667148176577,26.9365296811876));
#45665=CARTESIAN_POINT('Ctrl Pts',(9.65451474733602,0.537468143587547,27.2899993389655));
#45666=CARTESIAN_POINT('Ctrl Pts',(9.68627135383762,0.0937613626242288,
27.4504710862759));
#45667=CARTESIAN_POINT('Ctrl Pts',(9.71802796033921,-0.371876568579776,
27.3802506620641));
#45668=CARTESIAN_POINT('Ctrl Pts',(9.74978456684081,-0.748580824009798,
27.0936679080815));
#45669=CARTESIAN_POINT('Ctrl Pts',(9.7815411733424,-0.939721265234505,26.665804364338));
#45670=CARTESIAN_POINT('Ctrl Pts',(9.82388331534454,-0.89634841262424,26.0336291890481));
#45671=CARTESIAN_POINT('Ctrl Pts',(9.86622545734667,-0.394314069071067,
25.569696184457));
#45672=CARTESIAN_POINT('Ctrl Pts',(9.90856759934879,0.239316832616143,25.5762629832153));
#45673=CARTESIAN_POINT('Ctrl Pts',(9.94032420585039,0.650789571874067,25.8005057228205));
#45674=CARTESIAN_POINT('Ctrl Pts',(9.97208081235198,0.906814364531588,26.1986311613203));
#45675=CARTESIAN_POINT('Ctrl Pts',(10.0038374188536,0.940122666557803,26.6683225706626));
#45676=CARTESIAN_POINT('Ctrl Pts',(10.0355940253552,0.745222154778916,27.0980682396355));
#45677=CARTESIAN_POINT('Ctrl Pts',(10.0673506318568,0.368209093249168,27.3813418354716));
#45678=CARTESIAN_POINT('Ctrl Pts',(10.0991072383584,-0.0982720703761154,
27.4504652568396));
#45679=CARTESIAN_POINT('Ctrl Pts',(10.13086384486,-0.540965920742814,27.2870953841388));
#45680=CARTESIAN_POINT('Ctrl Pts',(10.1626204513616,-0.85169374061398,26.9333047730217));
#45681=CARTESIAN_POINT('Ctrl Pts',(10.1943770578631,-0.954986831558773,
26.4713710925651));
#45682=CARTESIAN_POINT('Ctrl Pts',(10.2261336643648,-0.825332603926062,
26.0210543415525));
#45683=CARTESIAN_POINT('Ctrl Pts',(10.2684758063669,-0.384694491533629,
25.5656782949712));
#45684=CARTESIAN_POINT('Ctrl Pts',(10.310817948369,0.298172024495185,25.5345776349681));
#45685=CARTESIAN_POINT('Ctrl Pts',(10.3531600903711,0.778379589008935,25.9480144315763));
#45686=CARTESIAN_POINT('Ctrl Pts',(10.3849166968727,0.948430841333095,26.3846813151855));
#45687=CARTESIAN_POINT('Ctrl Pts',(10.4166733033743,0.887555156211573,26.8540919408332));
#45688=CARTESIAN_POINT('Ctrl Pts',(10.4484299098759,0.610273299126541,27.2346630316351));
#45689=CARTESIAN_POINT('Ctrl Pts',(10.4801865163775,0.184262527222831,27.4375974170403));
#45690=CARTESIAN_POINT('Ctrl Pts',(10.5119431228791,-0.286570765530798,
27.4111633215117));
#45691=CARTESIAN_POINT('Ctrl Pts',(10.5436997293807,-0.687772514546559,
27.1633329206604));
#45692=CARTESIAN_POINT('Ctrl Pts',(10.5754563358823,-0.92093013211283,26.7530829140763));
#45693=CARTESIAN_POINT('Ctrl Pts',(10.6072129423839,-0.930454469678779,
26.2823081585637));
#45694=CARTESIAN_POINT('Ctrl Pts',(10.6389695488855,-0.711679597010942,
25.8625585431454));
#45695=CARTESIAN_POINT('Ctrl Pts',(10.6707261553871,-0.322293315397946,
25.6018408429898));
#45696=CARTESIAN_POINT('Ctrl Pts',(10.7130682973892,0.308115995869649,25.5377051219523));
#45697=CARTESIAN_POINT('Ctrl Pts',(10.7554104393913,0.850246395681263,25.9540806232981));
#45698=CARTESIAN_POINT('Ctrl Pts',(10.7977525813935,0.950900073946533,26.5796988195625));
#45699=CARTESIAN_POINT('Ctrl Pts',(10.8295091878951,0.799451144212613,27.023160900428));
#45700=CARTESIAN_POINT('Ctrl Pts',(10.8612657943967,0.450342041291193,27.3428091740228));
#45701=CARTESIAN_POINT('Ctrl Pts',(10.8930224008983,-0.00695681293825255,
27.4550470524467));
#45702=CARTESIAN_POINT('Ctrl Pts',(10.9247790073999,-0.463467182543916,
27.3356074234353));
#45703=CARTESIAN_POINT('Ctrl Pts',(10.9565356139015,-0.806403075589457,
27.0119135491492));
#45704=CARTESIAN_POINT('Ctrl Pts',(10.9882922204031,-0.953397519599223,
26.563833886121));
#45705=CARTESIAN_POINT('Ctrl Pts',(11.0200488269047,-0.867223863248237,
26.0998924636472));
#45706=CARTESIAN_POINT('Ctrl Pts',(11.0518054334063,-0.571059652597703,
25.7338236944761));
#45707=CARTESIAN_POINT('Ctrl Pts',(11.0835620399079,-0.133238974421134,
25.5539202806239));
#45708=CARTESIAN_POINT('Ctrl Pts',(11.1153186464094,0.332515466358953,25.6055748678044));
#45709=CARTESIAN_POINT('Ctrl Pts',(11.1576607884116,0.855833159021813,25.9628812951065));
#45710=CARTESIAN_POINT('Ctrl Pts',(11.2000029304137,1.00193559695058,26.6306597060727));
#45711=CARTESIAN_POINT('Ctrl Pts',(11.2423450724158,0.675637081015731,27.1738526450402));
#45712=CARTESIAN_POINT('Ctrl Pts',(11.2741016789174,0.274006008333107,27.4152814687936));
#45713=CARTESIAN_POINT('Ctrl Pts',(11.305858285419,-0.198939335039208,27.4346434608691));
#45714=CARTESIAN_POINT('Ctrl Pts',(11.3376148919206,-0.62091092787356,27.2256947631619));
#45715=CARTESIAN_POINT('Ctrl Pts',(11.3693714984222,-0.892947937991379,
26.8401258229424));
#45716=CARTESIAN_POINT('Ctrl Pts',(11.4011281049238,-0.946496248448144,
26.3716011923876));
#45717=CARTESIAN_POINT('Ctrl Pts',(11.4328847114254,-0.770062987601644,
25.9342751635987));
#45718=CARTESIAN_POINT('Ctrl Pts',(11.464641317927,-0.40513765195304,25.6351146014624));
#45719=CARTESIAN_POINT('Ctrl Pts',(11.4963979244286,0.0572499371661582,
25.5461353855679));
#45720=CARTESIAN_POINT('Ctrl Pts',(11.5281545309302,0.507944530381333,25.6907955673779));
#45721=CARTESIAN_POINT('Ctrl Pts',(11.5599111374318,0.830741094949436,26.030498045123));
#45722=CARTESIAN_POINT('Ctrl Pts',(11.6022532794339,1.00053431786251,26.640989283306));
#45723=CARTESIAN_POINT('Ctrl Pts',(11.644595421436,0.681808444057784,27.2457104966669));
#45724=CARTESIAN_POINT('Ctrl Pts',(11.6869375634382,0.0822132948446471,
27.4506859768724));
#45725=CARTESIAN_POINT('Ctrl Pts',(11.7186941699398,-0.380469891862701,
27.3763915341362));
#45726=CARTESIAN_POINT('Ctrl Pts',(11.7504507764414,-0.754539209241824,
27.0863495882901));
#45727=CARTESIAN_POINT('Ctrl Pts',(11.782207382943,-0.942475061715997,26.6546092742268));
#45728=CARTESIAN_POINT('Ctrl Pts',(11.8139639894446,-0.901935158882476,
26.1844773152895));
#45729=CARTESIAN_POINT('Ctrl Pts',(11.8457205959462,-0.640879726462179,
25.791752459706));
#45730=CARTESIAN_POINT('Ctrl Pts',(11.8774772024478,-0.224102042897375,
25.5711190228213));
#45731=CARTESIAN_POINT('Ctrl Pts',(11.9092338089494,0.247729853529148,25.5776154872809));
#45732=CARTESIAN_POINT('Ctrl Pts',(11.9409904154509,0.658600252589484,25.8076265709458));
#45733=CARTESIAN_POINT('Ctrl Pts',(11.9727470219526,0.909934481056709,26.2087291640008));
#45734=CARTESIAN_POINT('Ctrl Pts',(12.0045036284541,0.937766694451681,26.6765119804666));
#45735=CARTESIAN_POINT('Ctrl Pts',(12.0468457704563,0.674078991690957,27.2527047310789));
#45736=CARTESIAN_POINT('Ctrl Pts',(12.0891879124584,0.0406143730004874,
27.5096025811841));
#45737=CARTESIAN_POINT('Ctrl Pts',(12.1315300544605,-0.549925132422438,
27.2798366503321));
#45738=CARTESIAN_POINT('Ctrl Pts',(12.1632866609622,-0.85578066628253,26.9248045561627));
#45739=CARTESIAN_POINT('Ctrl Pts',(12.1950432674637,-0.954822893601219,
26.4619408378153));
#45740=CARTESIAN_POINT('Ctrl Pts',(12.2267998739653,-0.820223097137686,
26.0107175247821));
#45741=CARTESIAN_POINT('Ctrl Pts',(12.2585564804669,-0.486196719112702,
25.6774099771336));
#45742=CARTESIAN_POINT('Ctrl Pts',(12.2903130869685,-0.0334698188374221,
25.5454209444212));
#45743=CARTESIAN_POINT('Ctrl Pts',(12.3220696934701,0.427389645660999,25.6453774598239));
#45744=CARTESIAN_POINT('Ctrl Pts',(12.3538262999717,0.783940164013017,25.9544717341139));
#45745=CARTESIAN_POINT('Ctrl Pts',(12.3855829064733,0.949812500284005,26.395159777397));
#45746=CARTESIAN_POINT('Ctrl Pts',(12.4173395129749,0.883431851285648,26.8638236164045));
#45747=CARTESIAN_POINT('Ctrl Pts',(12.4490961194765,0.60319338861771,27.2394055642196));
#45748=CARTESIAN_POINT('Ctrl Pts',(12.4914382614786,0.0301965841333301,
27.5099678537134));
#45749=CARTESIAN_POINT('Ctrl Pts',(12.5337804034807,-0.619705204181141,
27.2980678913091));
#45750=CARTESIAN_POINT('Ctrl Pts',(12.5761225454829,-0.923101135526423,
26.7417584456868));
#45751=CARTESIAN_POINT('Ctrl Pts',(12.6078791519845,-0.928100155477381,
26.2731750429903));
#45752=CARTESIAN_POINT('Ctrl Pts',(12.6396357584861,-0.705475825344904,
25.8554543322424));
#45753=CARTESIAN_POINT('Ctrl Pts',(12.6713923649877,-0.311724079885715,
25.5972312767641));
#45754=CARTESIAN_POINT('Ctrl Pts',(12.7031489714893,0.158494124499654,25.557704288509));
#45755=CARTESIAN_POINT('Ctrl Pts',(12.7349055779909,0.5897011895471,25.7486053572393));
#45756=CARTESIAN_POINT('Ctrl Pts',(12.7666621844925,0.877621467780753,26.1220818148255));
#45757=CARTESIAN_POINT('Ctrl Pts',(12.7984187909941,0.950989231806714,26.5882198992358));
#45758=CARTESIAN_POINT('Ctrl Pts',(12.8301753974956,0.793753413987165,27.0320627554668));
#45759=CARTESIAN_POINT('Ctrl Pts',(12.8619320039973,0.440916858551541,27.3475917552481));
#45760=CARTESIAN_POINT('Ctrl Pts',(12.8936886104988,-0.0154266227514476,
27.4541094653034));
#45761=CARTESIAN_POINT('Ctrl Pts',(12.936030752501,-0.627905542014287,27.291632193342));
#45762=CARTESIAN_POINT('Ctrl Pts',(12.9783728945031,-0.988202581431092,
26.7107191431281));
#45763=CARTESIAN_POINT('Ctrl Pts',(13.0207150365052,-0.86158431644457,26.0898350110897));
#45764=CARTESIAN_POINT('Ctrl Pts',(13.0524716430068,-0.563372759635625,
25.7283585071938));
#45765=CARTESIAN_POINT('Ctrl Pts',(13.0842282495084,-0.123916753765488,
25.5524875219252));
#45766=CARTESIAN_POINT('Ctrl Pts',(13.11598485601,0.343567325343907,25.6088632189223));
#45767=CARTESIAN_POINT('Ctrl Pts',(13.1477414625116,0.728549312681536,25.8817302414103));
#45768=CARTESIAN_POINT('Ctrl Pts',(13.1794980690132,0.935179034674501,26.305625168224));
#45769=CARTESIAN_POINT('Ctrl Pts',(13.2112546755148,0.914577064838846,26.7767496844913));
#45770=CARTESIAN_POINT('Ctrl Pts',(13.2430112820164,0.670212837001825,27.180424883989));
#45771=CARTESIAN_POINT('Ctrl Pts',(13.274767888518,0.263911977775921,27.4184147897098));
#45772=CARTESIAN_POINT('Ctrl Pts',(13.3065244950196,-0.209228031077641,
27.4322248069704));
#45773=CARTESIAN_POINT('Ctrl Pts',(13.3382811015212,-0.626782162306477,
27.2195185706328));
#45774=CARTESIAN_POINT('Ctrl Pts',(13.3806232435233,-0.990323889191508,
26.7005130761929));
#45775=CARTESIAN_POINT('Ctrl Pts',(13.4229653855255,-0.891350548436152,
26.0241417237977));
#45776=CARTESIAN_POINT('Ctrl Pts',(13.4653075275276,-0.394343245000318,
25.6310602681465));
#45777=CARTESIAN_POINT('Ctrl Pts',(13.4970641340292,0.0666496135424663,
25.5469117098955));
#45778=CARTESIAN_POINT('Ctrl Pts',(13.5288207405308,0.515995320900319,25.6957089539351));
#45779=CARTESIAN_POINT('Ctrl Pts',(13.5605773470324,0.837071203165268,26.040135813022));
#45780=CARTESIAN_POINT('Ctrl Pts',(13.592333953534,0.955527079936532,26.4969024359207));
#45781=CARTESIAN_POINT('Ctrl Pts',(13.6240905600356,0.840276516062167,26.9541770345109));
#45782=CARTESIAN_POINT('Ctrl Pts',(13.6558471665372,0.520853866128242,27.3010947793704));
#45783=CARTESIAN_POINT('Ctrl Pts',(13.6876037730388,0.0738299518903651,
27.452214475755));
#45784=CARTESIAN_POINT('Ctrl Pts',(13.7193603795403,-0.390206894582817,
27.3722808248444));
#45785=CARTESIAN_POINT('Ctrl Pts',(13.751116986042,-0.76084642148672,27.0778686551721));
#45786=CARTESIAN_POINT('Ctrl Pts',(13.7828735925435,-0.942982927868766,
26.646102875465));
#45787=CARTESIAN_POINT('Ctrl Pts',(13.8252157345457,-0.886393891964172,
26.0149713745393));
#45788=CARTESIAN_POINT('Ctrl Pts',(13.8675578765478,-0.374757199409084,
25.561648285173));
#45789=CARTESIAN_POINT('Ctrl Pts',(13.9099000185499,0.258595981805174,25.5814734785183));
#45790=CARTESIAN_POINT('Ctrl Pts',(13.9416566250515,0.665286358978002,25.8142788319751));
#45791=CARTESIAN_POINT('Ctrl Pts',(13.9734132315531,0.912922684959164,26.2176749581455));
#45792=CARTESIAN_POINT('Ctrl Pts',(14.0051698380547,0.936394173098453,26.6879606932866));
#45793=CARTESIAN_POINT('Ctrl Pts',(14.0369264445563,0.732542489799628,27.1135332884477));
#45794=CARTESIAN_POINT('Ctrl Pts',(14.0686830510579,0.349683692101816,27.3888547224382));
#45795=CARTESIAN_POINT('Ctrl Pts',(14.1004396575595,-0.118141955808618,
27.4482004396081));
#45796=CARTESIAN_POINT('Ctrl Pts',(14.1321962640611,-0.55731981727521,27.2756016315776));
#45797=CARTESIAN_POINT('Ctrl Pts',(14.1639528705627,-0.860575439144756,
26.9153855696964));
#45798=CARTESIAN_POINT('Ctrl Pts',(14.1957094770643,-0.954178525076913,
26.4513913382035));
#45799=CARTESIAN_POINT('Ctrl Pts',(14.2274660835659,-0.815128438364575,
26.0038866244089));
#45800=CARTESIAN_POINT('Ctrl Pts',(14.269808225568,-0.365056692386834,25.5578320157364));
#45801=CARTESIAN_POINT('Ctrl Pts',(14.3121503675701,0.318311140684575,25.5410292408296));
#45802=CARTESIAN_POINT('Ctrl Pts',(14.3544925095723,0.789761100866001,25.9644253030342));
#45803=CARTESIAN_POINT('Ctrl Pts',(14.3862491160739,0.950636516610815,26.4045553929986));
#45804=CARTESIAN_POINT('Ctrl Pts',(14.4180057225755,0.879950308795002,26.8725892000887));
#45805=CARTESIAN_POINT('Ctrl Pts',(14.4497623290771,0.594764564687753,27.2472739673141));
#45806=CARTESIAN_POINT('Ctrl Pts',(14.4815189355787,0.164600072175658,27.4412483262322));
#45807=CARTESIAN_POINT('Ctrl Pts',(14.5132755420803,-0.305576886172813,
27.4049663909559));
#45808=CARTESIAN_POINT('Ctrl Pts',(14.5450321485819,-0.701504155152511,
27.1487938930808));
#45809=CARTESIAN_POINT('Ctrl Pts',(14.5767887550835,-0.926024969152664,
26.7337542002603));
#45810=CARTESIAN_POINT('Ctrl Pts',(14.608545361585,-0.925694816580148,26.2628832259669));
#45811=CARTESIAN_POINT('Ctrl Pts',(14.6403019680866,-0.698183312328932,
25.8478040769025));
#45812=CARTESIAN_POINT('Ctrl Pts',(14.6720585745883,-0.303425995824808,
25.5952925790462));
#45813=CARTESIAN_POINT('Ctrl Pts',(14.7144007165904,0.328187482238224,25.5443641510859));
#45814=CARTESIAN_POINT('Ctrl Pts',(14.7567428585925,0.861485213777406,25.9719941992074));
#45815=CARTESIAN_POINT('Ctrl Pts',(14.7990850005946,0.949023869712233,26.5995818617395));
#45816=CARTESIAN_POINT('Ctrl Pts',(14.8308416070962,0.788327306949261,27.0397772844774));
#45817=CARTESIAN_POINT('Ctrl Pts',(14.8625982135978,0.432605044989158,27.3520493724081));
#45818=CARTESIAN_POINT('Ctrl Pts',(14.8943548200994,-0.0269425750032053,
27.4546922893193));
#45819=CARTESIAN_POINT('Ctrl Pts',(14.926111426601,-0.480853321388377,27.3257249413122));
#45820=CARTESIAN_POINT('Ctrl Pts',(14.9578680331026,-0.816939819939113,
26.9949249768607));
#45821=CARTESIAN_POINT('Ctrl Pts',(14.9896246396042,-0.954524630017393,
26.5438671412952));
#45822=CARTESIAN_POINT('Ctrl Pts',(15.0213812461058,-0.858660451344394,
26.0818307771601));
#45823=CARTESIAN_POINT('Ctrl Pts',(15.0531378526074,-0.554899994784753,
25.7220403263928));
#45824=CARTESIAN_POINT('Ctrl Pts',(15.084894459109,-0.113410176167132,25.5513390533698));
#45825=CARTESIAN_POINT('Ctrl Pts',(15.1166510656106,0.351161226478998,25.6127296660606));
#45826=CARTESIAN_POINT('Ctrl Pts',(15.1589932076127,0.866886572506035,25.9809098636687));
#45827=CARTESIAN_POINT('Ctrl Pts',(15.2013353496149,0.998981702436636,26.65159966169));
#45828=CARTESIAN_POINT('Ctrl Pts',(15.243677491617,0.661386674545668,27.1878448365762));
#45829=CARTESIAN_POINT('Ctrl Pts',(15.2754340981186,0.254790927614128,27.4208154228319));
#45830=CARTESIAN_POINT('Ctrl Pts',(15.3071907046202,-0.218456042209027,
27.4302753439674));
#45831=CARTESIAN_POINT('Ctrl Pts',(15.3389473111218,-0.635962324857501,
27.2125413609015));
#45832=CARTESIAN_POINT('Ctrl Pts',(15.3707039176234,-0.89987054313192,26.821363658491));
#45833=CARTESIAN_POINT('Ctrl Pts',(15.402460524125,-0.943601812261104,26.3518209798243));
#45834=CARTESIAN_POINT('Ctrl Pts',(15.4342171306266,-0.758054806041372,
25.9182831389474));
#45835=CARTESIAN_POINT('Ctrl Pts',(15.4659737371282,-0.386948543494837,
25.626825278469));
#45836=CARTESIAN_POINT('Ctrl Pts',(15.4977303436297,0.0771999380983128,
25.547542427439));
#45837=CARTESIAN_POINT('Ctrl Pts',(15.5294869501314,0.524768364500619,25.7016030916023));
#45838=CARTESIAN_POINT('Ctrl Pts',(15.5612435566329,0.840384916331581,26.0479866762213));
#45839=CARTESIAN_POINT('Ctrl Pts',(15.6035856986351,0.997364552198828,26.6618976505233));
#45840=CARTESIAN_POINT('Ctrl Pts',(15.6459278406372,0.666052840252209,27.25981610487));
#45841=CARTESIAN_POINT('Ctrl Pts',(15.6882699826393,0.0622992719753226,
27.4521983266014));
#45842=CARTESIAN_POINT('Ctrl Pts',(15.7200265891409,-0.39872774090838,27.3682370922448));
#45843=CARTESIAN_POINT('Ctrl Pts',(15.7517831956425,-0.766645114785282,
27.0704301236322));
#45844=CARTESIAN_POINT('Ctrl Pts',(15.7835398021441,-0.945504317446849,
26.6348512340428));
#45845=CARTESIAN_POINT('Ctrl Pts',(15.8152964086457,-0.895134341830607,
26.1656706631617));
#45846=CARTESIAN_POINT('Ctrl Pts',(15.8470530151473,-0.625917113840984,
25.7784952053356));
#45847=CARTESIAN_POINT('Ctrl Pts',(15.8788096216489,-0.204613280560773,
25.566632440668));
#45848=CARTESIAN_POINT('Ctrl Pts',(15.9105662281505,0.266979318749092,25.5830020103654));
#45849=CARTESIAN_POINT('Ctrl Pts',(15.9423228346521,0.672946044002942,25.821561439899));
#45850=CARTESIAN_POINT('Ctrl Pts',(15.9740794411537,0.91583092558663,26.2278361238909));
#45851=CARTESIAN_POINT('Ctrl Pts',(16.0058360476553,0.933867254621135,26.6960989628159));
#45852=CARTESIAN_POINT('Ctrl Pts',(16.0481781896574,0.658178704973912,27.2666470449604));
#45853=CARTESIAN_POINT('Ctrl Pts',(16.0905203316595,0.0194764504986447,
27.5102314423456));
#45854=CARTESIAN_POINT('Ctrl Pts',(16.1328624736617,-0.566125161298197,
27.2681569853983));
#45855=CARTESIAN_POINT('Ctrl Pts',(16.1646190801633,-0.864483573584741,
26.9068016847578));
#45856=CARTESIAN_POINT('Ctrl Pts',(16.1963756866649,-0.953817267616392,
26.4419665788703));
#45857=CARTESIAN_POINT('Ctrl Pts',(16.2281322931665,-0.809803720332871,
25.993659004061));
#45858=CARTESIAN_POINT('Ctrl Pts',(16.2598888996681,-0.468875017752602,
25.6674149814447));
#45859=CARTESIAN_POINT('Ctrl Pts',(16.2916455061697,-0.0134849969651525,
25.5449295539179));
#45860=CARTESIAN_POINT('Ctrl Pts',(16.3234021126713,0.445181635637873,25.6545090735637));
#45861=CARTESIAN_POINT('Ctrl Pts',(16.3551587191728,0.795185319036783,25.970997563312));
#45862=CARTESIAN_POINT('Ctrl Pts',(16.3869153256744,0.951798579107647,26.4150604757497));
#45863=CARTESIAN_POINT('Ctrl Pts',(16.418671932176,0.875624241768845,26.8822324514563));
#45864=CARTESIAN_POINT('Ctrl Pts',(16.4504285386776,0.587586952789248,27.2518672924014));
#45865=CARTESIAN_POINT('Ctrl Pts',(16.4927706806798,0.00905329884619842,
27.5103786107236));
#45866=CARTESIAN_POINT('Ctrl Pts',(16.5351128226819,-0.636271494686479,
27.2849238716444));
#45867=CARTESIAN_POINT('Ctrl Pts',(16.577454964684,-0.927958497882414,26.7223867772124));
#45868=CARTESIAN_POINT('Ctrl Pts',(16.6092115711856,-0.923149879585831,
26.2538013819286));
#45869=CARTESIAN_POINT('Ctrl Pts',(16.6409681776872,-0.691832222007586,
25.8408312548647));
#45870=CARTESIAN_POINT('Ctrl Pts',(16.6727247841888,-0.292762605847151,
25.5909052160247));
#45871=CARTESIAN_POINT('Ctrl Pts',(16.7044813906904,0.178179836603969,25.5612276414258));
#45872=CARTESIAN_POINT('Ctrl Pts',(16.736237997192,0.605297270682226,25.7611112287851));
#45873=CARTESIAN_POINT('Ctrl Pts',(16.7679946036936,0.885338350632903,26.140531503058));
#45874=CARTESIAN_POINT('Ctrl Pts',(16.7997512101952,0.948934678345878,26.6081029410621));
#45875=CARTESIAN_POINT('Ctrl Pts',(16.8315078166968,0.782444526026321,27.0485579474062));
#45876=CARTESIAN_POINT('Ctrl Pts',(16.8632644231984,0.423081836349496,27.3566336553455));
#45877=CARTESIAN_POINT('Ctrl Pts',(16.8950210297,-0.0353909079102747,27.4535776508021));
#45878=CARTESIAN_POINT('Ctrl Pts',(16.9373631717021,-0.644335349815601,
27.2783179660028));
#45879=CARTESIAN_POINT('Ctrl Pts',(16.9797053137042,-0.992396093030616,
26.6899918255381));
#45880=CARTESIAN_POINT('Ctrl Pts',(17.0220474557064,-0.852811656678332,
26.0718935521386));
#45881=CARTESIAN_POINT('Ctrl Pts',(17.0538040622079,-0.547100409593038,
25.7167372078641));
#45882=CARTESIAN_POINT('Ctrl Pts',(17.0855606687096,-0.104060012346944,
25.5501017044901));
#45883=CARTESIAN_POINT('Ctrl Pts',(17.1173172752111,0.36214184608273,25.6162485910021));
#45884=CARTESIAN_POINT('Ctrl Pts',(17.1490738817128,0.741328937838052,25.8971127788516));
#45885=CARTESIAN_POINT('Ctrl Pts',(17.1808304882143,0.939042104386864,26.3252392260279));
#45886=CARTESIAN_POINT('Ctrl Pts',(17.212587094716,0.908584923009143,26.7958293990439));
#45887=CARTESIAN_POINT('Ctrl Pts',(17.2443437012175,0.655826073959799,27.1943021173535));
#45888=CARTESIAN_POINT('Ctrl Pts',(17.2761003077192,0.244633534093608,27.4237368086484));
#45889=CARTESIAN_POINT('Ctrl Pts',(17.3078569142207,-0.228691868279225,
27.4276418979317));
#45890=CARTESIAN_POINT('Ctrl Pts',(17.3396135207224,-0.641703015565117,
27.206243646366));
#45891=CARTESIAN_POINT('Ctrl Pts',(17.3819556627244,-0.994303347678889,
26.6797436015688));
#45892=CARTESIAN_POINT('Ctrl Pts',(17.4242978047266,-0.88119652697226,26.0055916982066));
#45893=CARTESIAN_POINT('Ctrl Pts',(17.4666399467287,-0.376071662495523,
25.6229977451693));
#45894=CARTESIAN_POINT('Ctrl Pts',(17.4983965532303,0.0865813322721645,
25.5485152861257));
#45895=CARTESIAN_POINT('Ctrl Pts',(17.5301531597319,0.532714518507328,25.706683914095));
#45896=CARTESIAN_POINT('Ctrl Pts',(17.5619097662335,0.846512025133718,26.0577547633947));
#45897=CARTESIAN_POINT('Ctrl Pts',(17.5936663727351,0.955382466040536,26.5169005346908));
#45898=CARTESIAN_POINT('Ctrl Pts',(17.6254229792367,0.83058774652791,26.9716627557347));
#45899=CARTESIAN_POINT('Ctrl Pts',(17.6571795857383,0.503973842045383,27.3118201059033));
#45900=CARTESIAN_POINT('Ctrl Pts',(17.6889361922399,0.0538868825730616,
27.4535504471568));
#45901=CARTESIAN_POINT('Ctrl Pts',(17.7206927987415,-0.408378664397602,
27.3639246296828));
#45902=CARTESIAN_POINT('Ctrl Pts',(17.7524494052431,-0.772769571707759,
27.0618169554814));
#45903=CARTESIAN_POINT('Ctrl Pts',(17.7842060117447,-0.945840995106025,
26.6263398149854));
#45904=CARTESIAN_POINT('Ctrl Pts',(17.8265481537468,-0.876033313989953,
25.9965186109302));
#45905=CARTESIAN_POINT('Ctrl Pts',(17.868890295749,-0.355067658577955,25.5540272619233));
#45906=CARTESIAN_POINT('Ctrl Pts',(17.911232437751,0.277799571538731,25.5870664787881));
#45907=CARTESIAN_POINT('Ctrl Pts',(17.9429890442527,0.679413189226427,25.8283943842124));
#45908=CARTESIAN_POINT('Ctrl Pts',(17.9747456507543,0.918783490271958,26.2367603996339));
#45909=CARTESIAN_POINT('Ctrl Pts',(18.0065022572559,0.931965741123502,26.7076726814112));
#45910=CARTESIAN_POINT('Ctrl Pts',(18.0382588637574,0.720089129555561,27.1284344314988));
#45911=CARTESIAN_POINT('Ctrl Pts',(18.070015470259,0.329980493973673,27.396531794444));
#45912=CARTESIAN_POINT('Ctrl Pts',(18.1017720767607,-0.136099813986084,
27.4445088971166));
#45913=CARTESIAN_POINT('Ctrl Pts',(18.1441142187627,-0.723118632728979,
27.2057172991734));
#45914=CARTESIAN_POINT('Ctrl Pts',(18.1864563607649,-1.00692062085995,26.5838971968947));
#45915=CARTESIAN_POINT('Ctrl Pts',(18.228798502767,-0.802712071566496,25.984024935646));
#45916=CARTESIAN_POINT('Ctrl Pts',(18.2605551092686,-0.46111876429496,25.6632320586692));
#45917=CARTESIAN_POINT('Ctrl Pts',(18.2923117157702,-0.00293339983474069,
25.5444214870179));
#45918=CARTESIAN_POINT('Ctrl Pts',(18.3240683222718,0.453650294894908,25.6595455626102));
#45919=CARTESIAN_POINT('Ctrl Pts',(18.3558249287734,0.800977642610365,25.9789660914556));
#45920=CARTESIAN_POINT('Ctrl Pts',(18.387581535275,0.952265047855294,26.4256156033654));
#45921=CARTESIAN_POINT('Ctrl Pts',(18.4193381417766,0.87216829080666,26.8903380035327));
#45922=CARTESIAN_POINT('Ctrl Pts',(18.4510947482782,0.5786525270315,27.259818867202));
#45923=CARTESIAN_POINT('Ctrl Pts',(18.4828513547798,0.14548490939909,27.4444412694929));
#45924=CARTESIAN_POINT('Ctrl Pts',(18.5146079612814,-0.325594867448101,
27.3982246211978));
#45925=CARTESIAN_POINT('Ctrl Pts',(18.546364567783,-0.712851699124399,27.1343542428059));
#45926=CARTESIAN_POINT('Ctrl Pts',(18.5887067097851,-1.00774305370889,26.5734903104616));
#45927=CARTESIAN_POINT('Ctrl Pts',(18.6310488517872,-0.823914981229908,
25.9150974327161));
#45928=CARTESIAN_POINT('Ctrl Pts',(18.6733909937894,-0.281131390701923,
25.5881184345652));
#45929=CARTESIAN_POINT('Ctrl Pts',(18.705147600291,0.186806312460487,25.5630246198324));
#45930=CARTESIAN_POINT('Ctrl Pts',(18.7369042067926,0.613691803981374,25.7675263640368));
#45931=CARTESIAN_POINT('Ctrl Pts',(18.7686608132942,0.888566765767323,26.1498395050539));
#45932=CARTESIAN_POINT('Ctrl Pts',(18.8004174197958,0.948226890816592,26.6179294670152));
#45933=CARTESIAN_POINT('Ctrl Pts',(18.8321740262974,0.775997695356658,27.0569281629903));
#45934=CARTESIAN_POINT('Ctrl Pts',(18.863930632799,0.415215011861205,27.3606033287324));
#45935=CARTESIAN_POINT('Ctrl Pts',(18.8956872393005,-0.0473470204057584,
27.4538980706808));
#45936=CARTESIAN_POINT('Ctrl Pts',(18.9274438458022,-0.497525842623222,
27.3158451408842));
#45937=CARTESIAN_POINT('Ctrl Pts',(18.9592004523037,-0.827898992667679,
26.9768676102035));
#45938=CARTESIAN_POINT('Ctrl Pts',(18.9909570588054,-0.953893041314731,
26.5255130985628));
#45939=CARTESIAN_POINT('Ctrl Pts',(19.0332992008074,-0.817836948170601,
25.9066285940149));
#45940=CARTESIAN_POINT('Ctrl Pts',(19.0756413428097,-0.252913115286982,
25.5217455058419));
#45941=CARTESIAN_POINT('Ctrl Pts',(19.1179834848117,0.372830731701806,25.6216150627598));
#45942=CARTESIAN_POINT('Ctrl Pts',(19.1497400913134,0.746766015262565,25.904047000034));
#45943=CARTESIAN_POINT('Ctrl Pts',(19.1814966978149,0.94132513800925,26.3355547430818));
#45944=CARTESIAN_POINT('Ctrl Pts',(19.2132533043165,0.905053565889767,26.8050267406374));
#45945=CARTESIAN_POINT('Ctrl Pts',(19.2450099108181,0.648951079631192,27.2013587467485));
#45946=CARTESIAN_POINT('Ctrl Pts',(19.2767665173197,0.234309457401578,27.425980820695));
#45947=CARTESIAN_POINT('Ctrl Pts',(19.3085231238213,-0.237265150323603,
27.4256062034349));
#45948=CARTESIAN_POINT('Ctrl Pts',(19.3402797303229,-0.651050566510682,
27.1987821044357));
#45949=CARTESIAN_POINT('Ctrl Pts',(19.3720363368245,-0.906249282199466,
26.8030635188936));
#45950=CARTESIAN_POINT('Ctrl Pts',(19.4037929433261,-0.940341432747018,
26.3309513396123));
#45951=CARTESIAN_POINT('Ctrl Pts',(19.4355495498277,-0.745741510409131,
25.9046577017179));
#45952=CARTESIAN_POINT('Ctrl Pts',(19.4778916918298,-0.242807432967905,
25.5191883719474));
#45953=CARTESIAN_POINT('Ctrl Pts',(19.520233833832,0.437186765681122,25.5890583821446));
#45954=CARTESIAN_POINT('Ctrl Pts',(19.5625759758341,0.85122504747574,26.0687474394035));
#45955=CARTESIAN_POINT('Ctrl Pts',(19.5943325823357,0.955069962351073,26.5257065504164));
#45956=CARTESIAN_POINT('Ctrl Pts',(19.6260891888373,0.825683878714483,26.9810211953773));
#45957=CARTESIAN_POINT('Ctrl Pts',(19.6578457953389,0.495346232074199,27.3165753976231));
#45958=CARTESIAN_POINT('Ctrl Pts',(19.6896024018405,0.0440810433938132,
27.454514775689));
#45959=CARTESIAN_POINT('Ctrl Pts',(19.7213590083421,-0.417716245692366,
27.3589845983528));
#45960=CARTESIAN_POINT('Ctrl Pts',(19.7531156148437,-0.778015997201674,
27.0547366073134));
#45961=CARTESIAN_POINT('Ctrl Pts',(19.7848722213452,-0.948171228861939,
26.6146062406326));
#45962=CARTESIAN_POINT('Ctrl Pts',(19.8166288278469,-0.888215519416682,
26.1475678093043));
#45963=CARTESIAN_POINT('Ctrl Pts',(19.8483854343484,-0.609972510687159,
25.7646409068179));
#45964=CARTESIAN_POINT('Ctrl Pts',(19.88014204085,-0.186416668901866,25.5641518937206));
#45965=CARTESIAN_POINT('Ctrl Pts',(19.9224841828522,0.446561285406313,25.5936171241666));
#45966=CARTESIAN_POINT('Ctrl Pts',(19.9648263248543,0.921413268661259,26.0853381045205));
#45967=CARTESIAN_POINT('Ctrl Pts',(20.0071684668564,0.928773341115951,26.718958747949));
#45968=CARTESIAN_POINT('Ctrl Pts',(20.038925073358,0.713626810946046,27.1352607609624));
#45969=CARTESIAN_POINT('Ctrl Pts',(20.0706816798596,0.321224058095783,27.3999724231729));
#45970=CARTESIAN_POINT('Ctrl Pts',(20.1024382863612,-0.147622055815055,
27.4435947214087));
#45971=CARTESIAN_POINT('Ctrl Pts',(20.1341948928628,-0.5815469709462,27.2581851462398));
#45972=CARTESIAN_POINT('Ctrl Pts',(20.1659514993644,-0.873037333522926,
26.8874883435638));
#45973=CARTESIAN_POINT('Ctrl Pts',(20.197708105866,-0.952395320404333,26.4226388400605));
#45974=CARTESIAN_POINT('Ctrl Pts',(20.2294647123676,-0.798793439930978,
25.9764617397393));
#45975=CARTESIAN_POINT('Ctrl Pts',(20.2612213188692,-0.451916741041312,
25.6580341354082));
#45976=CARTESIAN_POINT('Ctrl Pts',(20.2929779253708,0.00763543851914112,
25.5446146537662));
#45977=CARTESIAN_POINT('Ctrl Pts',(20.3247345318724,0.460692690237073,25.6643415185417));
#45978=CARTESIAN_POINT('Ctrl Pts',(20.3670766738745,0.925642118779168,26.0948659886288));
#45979=CARTESIAN_POINT('Ctrl Pts',(20.4094188158766,0.97174177418587,26.7768841337632));
#45980=CARTESIAN_POINT('Ctrl Pts',(20.4517609578788,0.568957743322508,27.2660613152904));
#45981=CARTESIAN_POINT('Ctrl Pts',(20.4835175643804,0.136133317385707,27.4456675840998));
#45982=CARTESIAN_POINT('Ctrl Pts',(20.515274170882,-0.33450173652478,27.395122252116));
#45983=CARTESIAN_POINT('Ctrl Pts',(20.5470307773836,-0.721074398387512,
27.1262706935691));
#45984=CARTESIAN_POINT('Ctrl Pts',(20.5787873838852,-0.933321683296651,
26.7048224374515));
#45985=CARTESIAN_POINT('Ctrl Pts',(20.6105439903868,-0.917240887448331,
26.233521939898));
#45986=CARTESIAN_POINT('Ctrl Pts',(20.6423005968884,-0.678287047037146,
25.8269708199366));
#45987=CARTESIAN_POINT('Ctrl Pts',(20.67405720339,-0.273259928313006,25.584853956348));
#45988=CARTESIAN_POINT('Ctrl Pts',(20.7058138098915,0.197191832486415,25.5649862893134));
#45989=CARTESIAN_POINT('Ctrl Pts',(20.7375704163932,0.621647822525948,25.7744840150153));
#45990=CARTESIAN_POINT('Ctrl Pts',(20.7693270228947,0.890859616989826,26.1580467937161));
#45991=CARTESIAN_POINT('Ctrl Pts',(20.8116691648969,0.968833568572465,26.7868944329102));
#45992=CARTESIAN_POINT('Ctrl Pts',(20.854011306899,0.564472343796524,27.3380440754021));
#45993=CARTESIAN_POINT('Ctrl Pts',(20.8963534489011,-0.0587828278361782,
27.4524218769131));
#45994=CARTESIAN_POINT('Ctrl Pts',(20.9281100554027,-0.505466018590451,
27.3107549344715));
#45995=CARTESIAN_POINT('Ctrl Pts',(20.9598666619043,-0.832709033680724,
26.9687546513878));
#45996=CARTESIAN_POINT('Ctrl Pts',(20.9916232684059,-0.954969293592875,
26.5140327448572));
#45997=CARTESIAN_POINT('Ctrl Pts',(21.0233798749075,-0.845590667720455,
26.0550078449463));
#45998=CARTESIAN_POINT('Ctrl Pts',(21.0551364814091,-0.529511238559754,
25.7050413530494));
#45999=CARTESIAN_POINT('Ctrl Pts',(21.0868930879107,-0.0847700985191855,
25.5482355197884));
#46000=CARTESIAN_POINT('Ctrl Pts',(21.1186496944123,0.380953014904775,25.6241929036207));
#46001=CARTESIAN_POINT('Ctrl Pts',(21.1504063009139,0.753441811352533,25.9122409550869));
#46002=CARTESIAN_POINT('Ctrl Pts',(21.1821629074155,0.94292321815782,26.3460023884001));
#46003=CARTESIAN_POINT('Ctrl Pts',(21.2139195139171,0.901516409720417,26.8127794997692));
#46004=CARTESIAN_POINT('Ctrl Pts',(21.2562616559192,0.555796570644303,27.343822890948));
#46005=CARTESIAN_POINT('Ctrl Pts',(21.2986037979214,-0.108609863467862,
27.5045649788765));
#46006=CARTESIAN_POINT('Ctrl Pts',(21.3409459399235,-0.658842278969386,
27.1902823363766));
#46007=CARTESIAN_POINT('Ctrl Pts',(21.3727025464251,-0.909038943717463,
26.7940538360991));
#46008=CARTESIAN_POINT('Ctrl Pts',(21.4044591529267,-0.938789589811806,
26.3216482014888));
#46009=CARTESIAN_POINT('Ctrl Pts',(21.4362157594283,-0.739164495713174,
25.8951867082226));
#46010=CARTESIAN_POINT('Ctrl Pts',(21.4679723659299,-0.359666886889135,
25.6147422263144));
#46011=CARTESIAN_POINT('Ctrl Pts',(21.4997289724315,0.107567832412902,25.5509106661896));
#46012=CARTESIAN_POINT('Ctrl Pts',(21.5314855789331,0.548665502402203,25.7176907504899));
#46013=CARTESIAN_POINT('Ctrl Pts',(21.5632421854347,0.855773327352228,26.0759536796221));
#46014=CARTESIAN_POINT('Ctrl Pts',(21.5949987919363,0.954892370388148,26.5362742187471));
#46015=CARTESIAN_POINT('Ctrl Pts',(21.6267553984379,0.82017147631701,26.9900389873832));
#46016=CARTESIAN_POINT('Ctrl Pts',(21.6585120049394,0.487644732810762,27.3202228154794));
#46017=CARTESIAN_POINT('Ctrl Pts',(21.7008541469416,-0.118967740312026,
27.5033910384256));
#46018=CARTESIAN_POINT('Ctrl Pts',(21.7431962889437,-0.730547156864122,
27.1980313394293));
#46019=CARTESIAN_POINT('Ctrl Pts',(21.7855384309458,-0.948649690972304,
26.6030854804968));
#46020=CARTESIAN_POINT('Ctrl Pts',(21.8172950374474,-0.88454100129426,26.1388813536399));
#46021=CARTESIAN_POINT('Ctrl Pts',(21.849051643949,-0.602789554197912,25.7585284824614));
#46022=CARTESIAN_POINT('Ctrl Pts',(21.8808082504506,-0.175283535498467,
25.5611501974135));
#46023=CARTESIAN_POINT('Ctrl Pts',(21.9125648569522,0.295625783321212,25.5913488063999));
#46024=CARTESIAN_POINT('Ctrl Pts',(21.9443214634538,0.693992687018111,25.8437107707054));
#46025=CARTESIAN_POINT('Ctrl Pts',(21.9760780699554,0.923731845074089,26.2555392182961));
#46026=CARTESIAN_POINT('Ctrl Pts',(22.007834676457,0.927605810512738,26.7273999338973));
#46027=CARTESIAN_POINT('Ctrl Pts',(22.0395912829586,0.706679459850598,27.1432257760666));
#46028=CARTESIAN_POINT('Ctrl Pts',(22.0713478894602,0.311196990298509,27.4033138396751));
#46029=CARTESIAN_POINT('Ctrl Pts',(22.1031044959618,-0.155861224646809,
27.4414192111503));
#46030=CARTESIAN_POINT('Ctrl Pts',(22.1454466379639,-0.737709562729427,
27.1904574572595));
#46031=CARTESIAN_POINT('Ctrl Pts',(22.1877887799661,-1.00846623477415,26.5627913413472));
#46032=CARTESIAN_POINT('Ctrl Pts',(22.2301309219682,-0.791733341554092,
25.9673451696054));
#46033=CARTESIAN_POINT('Ctrl Pts',(22.2618875284698,-0.443508391765042,
25.6537614011678));
#46034=CARTESIAN_POINT('Ctrl Pts',(22.2936441349714,0.0170670193553443,
25.5445713135867));
#46035=CARTESIAN_POINT('Ctrl Pts',(22.3254007414729,0.471139295586204,25.6692226328383));
#46036=CARTESIAN_POINT('Ctrl Pts',(22.3571573479746,0.811706831839087,25.9958436606161));
#46037=CARTESIAN_POINT('Ctrl Pts',(22.3889139544761,0.953613004085633,26.4455606708209));
#46038=CARTESIAN_POINT('Ctrl Pts',(22.4206705609778,0.863808361361245,26.9085054592507));
#46039=CARTESIAN_POINT('Ctrl Pts',(22.4524271674793,0.562624198088996,27.2717624513788));
#46040=CARTESIAN_POINT('Ctrl Pts',(22.484183773981,0.125687748636954,27.4472791815583));
#46041=CARTESIAN_POINT('Ctrl Pts',(22.5159403804825,-0.34432167464298,27.3912138038039));
#46042=CARTESIAN_POINT('Ctrl Pts',(22.5476969869841,-0.725971372042429,
27.1192967135759));
#46043=CARTESIAN_POINT('Ctrl Pts',(22.5900391289863,-1.00906035784248,26.5523840954732));
#46044=CARTESIAN_POINT('Ctrl Pts',(22.6323812709884,-0.811493649352943,
25.8979825946971));
#46045=CARTESIAN_POINT('Ctrl Pts',(22.6747234129905,-0.261985904172254,
25.5824346135091));
#46046=CARTESIAN_POINT('Ctrl Pts',(22.7064800194921,0.206374480275771,25.567139327868));
#46047=CARTESIAN_POINT('Ctrl Pts',(22.7382366259937,0.628886650341483,25.7805301681145));
#46048=CARTESIAN_POINT('Ctrl Pts',(22.7699932324953,0.895700336928616,26.1685121781128));
#46049=CARTESIAN_POINT('Ctrl Pts',(22.8017498389969,0.945551178504746,26.6377481913622));
#46050=CARTESIAN_POINT('Ctrl Pts',(22.8335064454985,0.764172311405064,27.0730463162821));
#46051=CARTESIAN_POINT('Ctrl Pts',(22.8652630520001,0.397113311698903,27.3691044891535));
#46052=CARTESIAN_POINT('Ctrl Pts',(22.8970196585017,-0.0672998903916815,
27.4526982703809));
#46053=CARTESIAN_POINT('Ctrl Pts',(22.9287762650033,-0.514490935776569,
27.3052542051893));
#46054=CARTESIAN_POINT('Ctrl Pts',(22.9605328715049,-0.837697585415996,
26.9594368456141));
#46055=CARTESIAN_POINT('Ctrl Pts',(22.9922894780065,-0.954218063318174,
26.5055443762862));
#46056=CARTESIAN_POINT('Ctrl Pts',(23.0346316200086,-0.805239714176764,
25.8896428079065));
#46057=CARTESIAN_POINT('Ctrl Pts',(23.0769737620108,-0.232384750750894,
25.5166667773099));
#46058=CARTESIAN_POINT('Ctrl Pts',(23.1193159040128,0.391131971913022,25.629610068407));
#46059=CARTESIAN_POINT('Ctrl Pts',(23.1510725105145,0.759074604071942,25.9198058900914));
#46060=CARTESIAN_POINT('Ctrl Pts',(23.1828291170161,0.944560493665858,26.3552908718259));
#46061=CARTESIAN_POINT('Ctrl Pts',(23.2145857235177,0.898471725645074,26.823900953765));
#46062=CARTESIAN_POINT('Ctrl Pts',(23.2463423300193,0.634130868366591,27.2147864276691));
#46063=CARTESIAN_POINT('Ctrl Pts',(23.2780989365208,0.214879154138892,27.4306816594514));
#46064=CARTESIAN_POINT('Ctrl Pts',(23.3098555430225,-0.25658433122915,27.420437980726));
#46065=CARTESIAN_POINT('Ctrl Pts',(23.3416121495241,-0.665532132593269,
27.1850038321932));
#46066=CARTESIAN_POINT('Ctrl Pts',(23.3733687560256,-0.912393331867455,
26.7840311002954));
#46067=CARTESIAN_POINT('Ctrl Pts',(23.4051253625272,-0.936597621847152,
26.3113088383897));
#46068=CARTESIAN_POINT('Ctrl Pts',(23.4368819690288,-0.733118819505304,
25.8891811651903));
#46069=CARTESIAN_POINT('Ctrl Pts',(23.479224111031,-0.222227765874648,25.5143216958347));
#46070=CARTESIAN_POINT('Ctrl Pts',(23.5215662530331,0.456155259187886,25.5984073654122));
#46071=CARTESIAN_POINT('Ctrl Pts',(23.5639083950352,0.860063896779621,26.0866563827427));
#46072=CARTESIAN_POINT('Ctrl Pts',(23.5956650015368,0.954322798502375,26.5456886854505));
#46073=CARTESIAN_POINT('Ctrl Pts',(23.6274216080384,0.815436198503803,26.9981958090358));
#46074=CARTESIAN_POINT('Ctrl Pts',(23.65917821454,0.478148401286439,27.3267631922024));
#46075=CARTESIAN_POINT('Ctrl Pts',(23.6909348210416,0.0240952427481605,
27.455228252656));
#46076=CARTESIAN_POINT('Ctrl Pts',(23.7226914275432,-0.43560164372991,27.3500544747853));
#46077=CARTESIAN_POINT('Ctrl Pts',(23.7544480340448,-0.789455162469809,
27.0383327426834));
#46078=CARTESIAN_POINT('Ctrl Pts',(23.7862046405464,-0.950362050999274,
26.5947377519997));
#46079=CARTESIAN_POINT('Ctrl Pts',(23.817961247048,-0.880645262685305,26.1290563664367));
#46080=CARTESIAN_POINT('Ctrl Pts',(23.8497178535496,-0.594449274927437,
25.7520364184949));
#46081=CARTESIAN_POINT('Ctrl Pts',(23.8814744600511,-0.166790351739,25.5604555193937));
#46082=CARTESIAN_POINT('Ctrl Pts',(23.9238166020534,0.465432320099869,25.6031612995448));
#46083=CARTESIAN_POINT('Ctrl Pts',(23.9661587440554,0.929889535128502,26.1047123178162));
#46084=CARTESIAN_POINT('Ctrl Pts',(24.0085008860576,0.923987542311717,26.7383482203077));
#46085=CARTESIAN_POINT('Ctrl Pts',(24.0402574925592,0.700175737535662,27.1500564562298));
#46086=CARTESIAN_POINT('Ctrl Pts',(24.0720140990608,0.302319024557154,27.4064979124974));
#46087=CARTESIAN_POINT('Ctrl Pts',(24.1037707055624,-0.167337334837971,
27.440298615336));
#46088=CARTESIAN_POINT('Ctrl Pts',(24.135527312064,-0.597286950075481,27.2458484394733));
#46089=CARTESIAN_POINT('Ctrl Pts',(24.1672839185655,-0.880955505259544,
26.869132496369));
#46090=CARTESIAN_POINT('Ctrl Pts',(24.1990405250672,-0.950567711377221,
26.4027239932854));
#46091=CARTESIAN_POINT('Ctrl Pts',(24.2307971315687,-0.787661849304617,
25.9598592028151));
#46092=CARTESIAN_POINT('Ctrl Pts',(24.2625537380703,-0.434197048688617,
25.6487607969077));
#46093=CARTESIAN_POINT('Ctrl Pts',(24.294310344572,0.0276281317882825,25.5449836933049));
#46094=CARTESIAN_POINT('Ctrl Pts',(24.3260669510735,0.478080505285049,25.674165947095));
#46095=CARTESIAN_POINT('Ctrl Pts',(24.3684090930757,0.933918058893733,26.1143266168117));
#46096=CARTESIAN_POINT('Ctrl Pts',(24.4107512350778,0.965734298436713,26.7971601656526));
#46097=CARTESIAN_POINT('Ctrl Pts',(24.45309337708,0.552800952384084,27.2778007196669));
#46098=CARTESIAN_POINT('Ctrl Pts',(24.4848499835815,0.116312510417921,27.4483094746125));
#46099=CARTESIAN_POINT('Ctrl Pts',(24.5166065900832,-0.353161650990287,
27.3879257323904));
#46100=CARTESIAN_POINT('Ctrl Pts',(24.5483631965847,-0.734023104698332,
27.1110428392531));
#46101=CARTESIAN_POINT('Ctrl Pts',(24.5801198030863,-0.937403808050388,
26.685244962274));
#46102=CARTESIAN_POINT('Ctrl Pts',(24.6118764095879,-0.911463127234907,
26.2143842269519));
#46103=CARTESIAN_POINT('Ctrl Pts',(24.6436330160895,-0.664053293709996,
25.8129229893904));
#46104=CARTESIAN_POINT('Ctrl Pts',(24.6753896225911,-0.254047845183442,
25.5793355866597));
#46105=CARTESIAN_POINT('Ctrl Pts',(24.7071462290927,0.216716670998938,25.5693179154607));
#46106=CARTESIAN_POINT('Ctrl Pts',(24.7389028355943,0.636695316637121,25.7876527998988));
#46107=CARTESIAN_POINT('Ctrl Pts',(24.7706594420959,0.897820923101191,26.1767656538782));
#46108=CARTESIAN_POINT('Ctrl Pts',(24.813001584098,0.962617233586659,26.8071074092719));
#46109=CARTESIAN_POINT('Ctrl Pts',(24.8553437261002,0.546810075430422,27.3496738436809));
#46110=CARTESIAN_POINT('Ctrl Pts',(24.8976858681022,-0.0787022993379347,
27.4509830705907));
#46111=CARTESIAN_POINT('Ctrl Pts',(24.9294424746039,-0.522322844544992,
27.2999989411156));
#46112=CARTESIAN_POINT('Ctrl Pts',(24.9611990811055,-0.842336784437806,
26.9512249988135));
#46113=CARTESIAN_POINT('Ctrl Pts',(24.9929556876071,-0.955053818302088,
26.4940440130873));
#46114=CARTESIAN_POINT('Ctrl Pts',(25.0247122941086,-0.836092645663481,
26.0374087298028));
#46115=CARTESIAN_POINT('Ctrl Pts',(25.0564689006103,-0.512758321830771,
25.6941338166197));
#46116=CARTESIAN_POINT('Ctrl Pts',(25.0882255071118,-0.0648329446824077,
25.5466698973183));
#46117=CARTESIAN_POINT('Ctrl Pts',(25.1199821136134,0.399198526988075,25.6323573283407));
#46118=CARTESIAN_POINT('Ctrl Pts',(25.151738720115,0.765577454441822,25.9281377620251));
#46119=CARTESIAN_POINT('Ctrl Pts',(25.1834953266166,0.945939574820729,26.3657696736668));
#46120=CARTESIAN_POINT('Ctrl Pts',(25.2152519331182,0.894773093931002,26.831577989089));
#46121=CARTESIAN_POINT('Ctrl Pts',(25.2575940751203,0.538015262989621,27.3552698264395));
#46122=CARTESIAN_POINT('Ctrl Pts',(25.2999362171226,-0.129609676224257,
27.5020719690006));
#46123=CARTESIAN_POINT('Ctrl Pts',(25.3422783591246,-0.673144254854347,
27.1763428602625));
#46124=CARTESIAN_POINT('Ctrl Pts',(25.3740349656263,-0.914993827187637,
26.7749650085504));
#46125=CARTESIAN_POINT('Ctrl Pts',(25.4057915721278,-0.934851422122379,
26.3020402148696));
#46126=CARTESIAN_POINT('Ctrl Pts',(25.4375481786294,-0.726345035721426,
25.8798498901769));
#46127=CARTESIAN_POINT('Ctrl Pts',(25.469304785131,-0.341061382887417,25.6074089802713));
#46128=CARTESIAN_POINT('Ctrl Pts',(25.5010613916326,0.127406875554477,25.5533697183237));
#46129=CARTESIAN_POINT('Ctrl Pts',(25.5328179981342,0.564917553857126,25.7293445953454));
#46130=CARTESIAN_POINT('Ctrl Pts',(25.5645746046358,0.864460367880076,26.0939562313707));
#46131=CARTESIAN_POINT('Ctrl Pts',(25.5963312111374,0.953924084549553,26.5562503226398));
#46132=CARTESIAN_POINT('Ctrl Pts',(25.628087817639,0.809736278571705,27.0070962620883));
#46133=CARTESIAN_POINT('Ctrl Pts',(25.6598444241406,0.470372255221548,27.3302486337547));
#46134=CARTESIAN_POINT('Ctrl Pts',(25.7021865661427,-0.139940715869016,
27.5006815153371));
#46135=CARTESIAN_POINT('Ctrl Pts',(25.7445287081448,-0.744995600564553,
27.1825895219264));
#46136=CARTESIAN_POINT('Ctrl Pts',(25.786870850147,-0.950599300264946,26.5832095017703));
#46137=CARTESIAN_POINT('Ctrl Pts',(25.8186274566486,-0.876789760428042,
26.1204487138737));
#46138=CARTESIAN_POINT('Ctrl Pts',(25.8503840631502,-0.587139966938427,
25.7460756580744));
#46139=CARTESIAN_POINT('Ctrl Pts',(25.8821406696517,-0.155596843591253,
25.5576874757268));
#46140=CARTESIAN_POINT('Ctrl Pts',(25.9138972761533,0.314577359308573,25.5977346901905));
#46141=CARTESIAN_POINT('Ctrl Pts',(25.945653882655,0.707575530836875,25.8583784328245));
#46142=CARTESIAN_POINT('Ctrl Pts',(25.9774104891565,0.928645668614596,26.2749246761696));
#46143=CARTESIAN_POINT('Ctrl Pts',(26.0091670956582,0.922643525462191,26.7467631270934));
#46144=CARTESIAN_POINT('Ctrl Pts',(26.0409237021597,0.693063374361549,27.157874325207));
#46145=CARTESIAN_POINT('Ctrl Pts',(26.0726803086614,0.292223927478923,27.4096287632192));
#46146=CARTESIAN_POINT('Ctrl Pts',(26.1044369151629,-0.175528640725272,
27.4379511281708));
#46147=CARTESIAN_POINT('Ctrl Pts',(26.146779057165,-0.751999129248255,27.1748674565358));
#46148=CARTESIAN_POINT('Ctrl Pts',(26.1891211991672,-1.00955714772251,26.541672240212));
#46149=CARTESIAN_POINT('Ctrl Pts',(26.2314633411693,-0.780415343064855,
25.9508925097247));
#46150=CARTESIAN_POINT('Ctrl Pts',(26.2632199476709,-0.425695156036877,
25.6446647035882));
#46151=CARTESIAN_POINT('Ctrl Pts',(26.2949765541725,0.0370469523678254,
25.5451382646459));
#46152=CARTESIAN_POINT('Ctrl Pts',(26.3267331606741,0.488444757764112,25.6792636247976));
#46153=CARTESIAN_POINT('Ctrl Pts',(26.3584897671757,0.822038272830759,26.0129434951272));
#46154=CARTESIAN_POINT('Ctrl Pts',(26.3902463736773,0.954622403718847,26.4655254939658));
#46155=CARTESIAN_POINT('Ctrl Pts',(26.4220029801789,0.854921065716908,26.926507465775));
#46156=CARTESIAN_POINT('Ctrl Pts',(26.44317405118,0.649394243932496,27.1643710019258));
#46157=CARTESIAN_POINT('Ctrl Pts',(26.4537595866805,0.524425129394093,27.2515709455267));
#46158=CARTESIAN_POINT('Ctrl Pts',(9.57962246391563,0.728031715487703,26.0801881597144));
#46159=CARTESIAN_POINT('Ctrl Pts',(9.59020799941616,0.797836853998554,26.2012432369256));
#46160=CARTESIAN_POINT('Ctrl Pts',(9.61137907041722,0.875864683195867,26.4787529255437));
#46161=CARTESIAN_POINT('Ctrl Pts',(9.64313567691882,0.779159006304305,26.9003050292651));
#46162=CARTESIAN_POINT('Ctrl Pts',(9.67489228342041,0.492867289945966,27.224442625857));
#46163=CARTESIAN_POINT('Ctrl Pts',(9.70664888992201,0.0859807399742794,
27.3715979059481));
#46164=CARTESIAN_POINT('Ctrl Pts',(9.73840549642361,-0.341017042102029,
27.3072046007951));
#46165=CARTESIAN_POINT('Ctrl Pts',(9.7701621029252,-0.686461153906695,27.0444034153001));
#46166=CARTESIAN_POINT('Ctrl Pts',(9.8019187094268,-0.861740140000044,26.6520453792238));
#46167=CARTESIAN_POINT('Ctrl Pts',(9.84426085142894,-0.821966507686613,
26.0723301549197));
#46168=CARTESIAN_POINT('Ctrl Pts',(9.88660299343105,-0.361592605867576,
25.6468958191038));
#46169=CARTESIAN_POINT('Ctrl Pts',(9.9289451354332,0.21945754392555,25.6529176835553));
#46170=CARTESIAN_POINT('Ctrl Pts',(9.96070174193477,0.596784937752111,25.8585520317075));
#46171=CARTESIAN_POINT('Ctrl Pts',(9.99245834843639,0.83156396088418,26.2236397271795));
#46172=CARTESIAN_POINT('Ctrl Pts',(10.024214954938,0.862108231736756,26.6543546166019));
#46173=CARTESIAN_POINT('Ctrl Pts',(10.0559715614396,0.683381197966278,27.048438593038));
#46174=CARTESIAN_POINT('Ctrl Pts',(10.0877281679412,0.33765390579586,27.3082052250863));
#46175=CARTESIAN_POINT('Ctrl Pts',(10.1194847744428,-0.0901171345344043,
27.3715925602575));
#46176=CARTESIAN_POINT('Ctrl Pts',(10.1512413809444,-0.496074810183009,
27.2217796506413));
#46177=CARTESIAN_POINT('Ctrl Pts',(10.182997987446,-0.781017425513611,26.8973477344617));
#46178=CARTESIAN_POINT('Ctrl Pts',(10.2147545939475,-0.875738920008686,
26.4737468123648));
#46179=CARTESIAN_POINT('Ctrl Pts',(10.2465112004492,-0.756843821637242,
26.0607988091448));
#46180=CARTESIAN_POINT('Ctrl Pts',(10.2888533424513,-0.352771292143462,
25.6432113471481));
#46181=CARTESIAN_POINT('Ctrl Pts',(10.3311954844534,0.273428740668571,25.6146915210074));
#46182=CARTESIAN_POINT('Ctrl Pts',(10.3735376264555,0.713787120522742,25.993819988321));
#46183=CARTESIAN_POINT('Ctrl Pts',(10.4052942329571,0.869726967162744,26.3942508345048));
#46184=CARTESIAN_POINT('Ctrl Pts',(10.4370508394587,0.813902944274307,26.8247082405763));
#46185=CARTESIAN_POINT('Ctrl Pts',(10.4688074459603,0.559630837018874,27.1736983051843));
#46186=CARTESIAN_POINT('Ctrl Pts',(10.5005640524619,0.168971823752622,27.3597925356327));
#46187=CARTESIAN_POINT('Ctrl Pts',(10.5323206589635,-0.262790191883949,
27.3355520272775));
#46188=CARTESIAN_POINT('Ctrl Pts',(10.5640772654651,-0.630698915625386,
27.1082873986829));
#46189=CARTESIAN_POINT('Ctrl Pts',(10.5958338719667,-0.844508356187008,
26.7320812711984));
#46190=CARTESIAN_POINT('Ctrl Pts',(10.6275904784683,-0.853242333262068,
26.3003729351923));
#46191=CARTESIAN_POINT('Ctrl Pts',(10.6593470849699,-0.652622110674877,
25.9154555072938));
#46192=CARTESIAN_POINT('Ctrl Pts',(10.6911036914715,-0.295548368443942,
25.6763730093826));
#46193=CARTESIAN_POINT('Ctrl Pts',(10.7334458334736,0.282547528974645,25.6175594789554));
#46194=CARTESIAN_POINT('Ctrl Pts',(10.7757879754757,0.779690185968125,25.9993827877349));
#46195=CARTESIAN_POINT('Ctrl Pts',(10.8181301174779,0.871991294827471,26.5730851524473));
#46196=CARTESIAN_POINT('Ctrl Pts',(10.8498867239795,0.733110089580741,26.9797473083307));
#46197=CARTESIAN_POINT('Ctrl Pts',(10.8816433304811,0.412971194829101,27.2728701291382));
#46198=CARTESIAN_POINT('Ctrl Pts',(10.9133999369827,-0.00637951398688148,
27.3757941435716));
#46199=CARTESIAN_POINT('Ctrl Pts',(10.9451565434843,-0.425007169196209,
27.2662660032243));
#46200=CARTESIAN_POINT('Ctrl Pts',(10.9769131499859,-0.739485127094044,
26.9694332988216));
#46201=CARTESIAN_POINT('Ctrl Pts',(11.0086697564875,-0.874281494321734,
26.5585367427531));
#46202=CARTESIAN_POINT('Ctrl Pts',(11.0404263629891,-0.795258808089696,
26.133094687598));
#46203=CARTESIAN_POINT('Ctrl Pts',(11.0721829694907,-0.523671266346352,
25.7974034948309));
#46204=CARTESIAN_POINT('Ctrl Pts',(11.1039395759923,-0.122182371218882,
25.6324290510517));
#46205=CARTESIAN_POINT('Ctrl Pts',(11.1356961824939,0.304922252090156,25.6797971726802));
#46206=CARTESIAN_POINT('Ctrl Pts',(11.178038324496,0.78481334152642,26.0074531511894));
#46207=CARTESIAN_POINT('Ctrl Pts',(11.2203804664981,0.918791724237265,26.6198171389421));
#46208=CARTESIAN_POINT('Ctrl Pts',(11.2627226085002,0.619570519816269,27.1179341621384));
#46209=CARTESIAN_POINT('Ctrl Pts',(11.2944792150018,0.251268099081413,27.3393284373114));
#46210=CARTESIAN_POINT('Ctrl Pts',(11.3262358215034,-0.182430702348097,
27.3570837083467));
#46211=CARTESIAN_POINT('Ctrl Pts',(11.357992428005,-0.569385720753886,27.1654742527812));
#46212=CARTESIAN_POINT('Ctrl Pts',(11.3897490345066,-0.818848215492295,
26.8119010765462));
#46213=CARTESIAN_POINT('Ctrl Pts',(11.4215056410082,-0.867952913083958,
26.3822561428148));
#46214=CARTESIAN_POINT('Ctrl Pts',(11.4532622475098,-0.706160657734097,
25.9812208494608));
#46215=CARTESIAN_POINT('Ctrl Pts',(11.4850188540114,-0.371518012659009,
25.706885603218));
#46216=CARTESIAN_POINT('Ctrl Pts',(11.516775460513,0.0524991512842034,25.6252901718929));
#46217=CARTESIAN_POINT('Ctrl Pts',(11.5485320670146,0.46579364213261,25.7579459815859));
#46218=CARTESIAN_POINT('Ctrl Pts',(11.5802886735162,0.761803498494695,26.0694588434954));
#46219=CARTESIAN_POINT('Ctrl Pts',(11.6226308155183,0.917506727842895,26.6292895342794));
#46220=CARTESIAN_POINT('Ctrl Pts',(11.6649729575205,0.625229763092544,27.183829015657));
#46221=CARTESIAN_POINT('Ctrl Pts',(11.7073150995226,0.0753909683970407,
27.3717949642245));
#46222=CARTESIAN_POINT('Ctrl Pts',(11.7390717060242,-0.348897263485596,
27.3036657158471));
#46223=CARTESIAN_POINT('Ctrl Pts',(11.7708283125258,-0.691925092963921,
27.0376923934737));
#46224=CARTESIAN_POINT('Ctrl Pts',(11.8025849190274,-0.86426541749805,26.6417792940806));
#46225=CARTESIAN_POINT('Ctrl Pts',(11.834341525529,-0.827089647580133,26.2106604133007));
#46226=CARTESIAN_POINT('Ctrl Pts',(11.8660981320305,-0.58769744352536,25.8505251428195));
#46227=CARTESIAN_POINT('Ctrl Pts',(11.8978547385322,-0.205505326914698,
25.6482005857156));
#46228=CARTESIAN_POINT('Ctrl Pts',(11.9296113450337,0.22717242501594,25.654157952437));
#46229=CARTESIAN_POINT('Ctrl Pts',(11.9613679515354,0.603947462792471,25.8650819687084));
#46230=CARTESIAN_POINT('Ctrl Pts',(11.9931245580369,0.834425159997837,26.2328997647731));
#46231=CARTESIAN_POINT('Ctrl Pts',(12.0248811645385,0.859947765854294,26.66186444256));
#46232=CARTESIAN_POINT('Ctrl Pts',(12.0672233065407,0.61814172580837,27.1902428457621));
#46233=CARTESIAN_POINT('Ctrl Pts',(12.1095654485428,0.0372440603084071,
27.4258224771968));
#46234=CARTESIAN_POINT('Ctrl Pts',(12.1519075905449,-0.504290557354765,
27.2151232701611));
#46235=CARTESIAN_POINT('Ctrl Pts',(12.1836641970465,-0.784765204805277,
26.8895528932284));
#46236=CARTESIAN_POINT('Ctrl Pts',(12.2154208035481,-0.875588586155747,
26.465099110808));
#46237=CARTESIAN_POINT('Ctrl Pts',(12.2471774100497,-0.752158318331058,
26.0513197750307));
#46238=CARTESIAN_POINT('Ctrl Pts',(12.2789340165513,-0.445850534936249,
25.7456711711312));
#46239=CARTESIAN_POINT('Ctrl Pts',(12.3106906230529,-0.0306923844737817,
25.624635017395));
#46240=CARTESIAN_POINT('Ctrl Pts',(12.3424472295545,0.39192346359699,25.7162968162322));
#46241=CARTESIAN_POINT('Ctrl Pts',(12.3742038360561,0.718886260937855,25.9997414429039));
#46242=CARTESIAN_POINT('Ctrl Pts',(12.4059604425577,0.870993971562706,26.4038597598608));
#46243=CARTESIAN_POINT('Ctrl Pts',(12.4377170490593,0.810121804594295,26.833632350075));
#46244=CARTESIAN_POINT('Ctrl Pts',(12.4694736555609,0.553138440497928,27.1780472869989));
#46245=CARTESIAN_POINT('Ctrl Pts',(12.511815797563,0.0276907734253708,27.4261574382243));
#46246=CARTESIAN_POINT('Ctrl Pts',(12.5541579395651,-0.568280051932768,
27.2318416234996));
#46247=CARTESIAN_POINT('Ctrl Pts',(12.5965000815673,-0.846499202680308,
26.721696544007));
#46248=CARTESIAN_POINT('Ctrl Pts',(12.6282566880689,-0.851083387706002,
26.2919977152372));
#46249=CARTESIAN_POINT('Ctrl Pts',(12.6600132945705,-0.646933148147585,
25.9089408269044));
#46250=CARTESIAN_POINT('Ctrl Pts',(12.6917699010721,-0.28585620245073,25.6721459599461));
#46251=CARTESIAN_POINT('Ctrl Pts',(12.7235265075737,0.145341766849772,25.6358990496622));
#46252=CARTESIAN_POINT('Ctrl Pts',(12.7552831140753,0.540765867963709,25.8109585271689));
#46253=CARTESIAN_POINT('Ctrl Pts',(12.7870397205769,0.804793585599763,26.153442694287));
#46254=CARTESIAN_POINT('Ctrl Pts',(12.8187963270785,0.872073054078602,26.5808991252308));
#46255=CARTESIAN_POINT('Ctrl Pts',(12.85055293358,0.727885175530364,26.9879104585021));
#46256=CARTESIAN_POINT('Ctrl Pts',(12.8823095400817,0.404328144390558,27.2772558362273));
#46257=CARTESIAN_POINT('Ctrl Pts',(12.9140661465832,-0.014146471449928,
27.3749343604572));
#46258=CARTESIAN_POINT('Ctrl Pts',(12.9564082885854,-0.575799899076613,
27.2259399806695));
#46259=CARTESIAN_POINT('Ctrl Pts',(12.9987504305875,-0.906198318985923,
26.6932329836706));
#46260=CARTESIAN_POINT('Ctrl Pts',(13.0410925725896,-0.790087249211633,
26.1238718351462));
#46261=CARTESIAN_POINT('Ctrl Pts',(13.0728491790912,-0.516622256749178,
25.7923918265544));
#46262=CARTESIAN_POINT('Ctrl Pts',(13.1046057855928,-0.113633738735928,
25.6311151873271));
#46263=CARTESIAN_POINT('Ctrl Pts',(13.1363623920944,0.315056991891516,25.6828126457333));
#46264=CARTESIAN_POINT('Ctrl Pts',(13.168118998596,0.668091922502613,25.9330362757174));
#46265=CARTESIAN_POINT('Ctrl Pts',(13.1998756050976,0.857574838496823,26.3217550235969));
#46266=CARTESIAN_POINT('Ctrl Pts',(13.2316322115992,0.838682487086633,26.7537840960733));
#46267=CARTESIAN_POINT('Ctrl Pts',(13.2633888181008,0.61459639720261,27.1239610153356));
#46268=CARTESIAN_POINT('Ctrl Pts',(13.2951454246024,0.242011703991384,27.3422017450729));
#46269=CARTESIAN_POINT('Ctrl Pts',(13.326902031104,-0.191865608944966,27.3548657622106));
#46270=CARTESIAN_POINT('Ctrl Pts',(13.3586586376056,-0.574769741068602,
27.1598105807844));
#46271=CARTESIAN_POINT('Ctrl Pts',(13.4010007796077,-0.908143593732887,
26.6838738493453));
#46272=CARTESIAN_POINT('Ctrl Pts',(13.4433429216098,-0.817383382514841,
26.0636299903754));
#46273=CARTESIAN_POINT('Ctrl Pts',(13.485685063612,-0.361619360683378,25.7031677116595));
#46274=CARTESIAN_POINT('Ctrl Pts',(13.5174416701136,0.061118811960344,25.6260020743044));
#46275=CARTESIAN_POINT('Ctrl Pts',(13.5491982766152,0.473176351884539,25.7624516393552));
#46276=CARTESIAN_POINT('Ctrl Pts',(13.5809548831168,0.767608313754213,26.0782968380857));
#46277=CARTESIAN_POINT('Ctrl Pts',(13.6127114896184,0.876234336819935,26.4971594818568));
#46278=CARTESIAN_POINT('Ctrl Pts',(13.64446809612,0.770547639367812,26.9164879478454));
#46279=CARTESIAN_POINT('Ctrl Pts',(13.6762247026215,0.477631719236381,27.2346173305503));
#46280=CARTESIAN_POINT('Ctrl Pts',(13.7079813091232,0.0677033024918876,
27.3731966233013));
#46281=CARTESIAN_POINT('Ctrl Pts',(13.7397379156247,-0.357826258069027,
27.2998961265745));
#46282=CARTESIAN_POINT('Ctrl Pts',(13.7714945221263,-0.697708912234596,
27.0299152357539));
#46283=CARTESIAN_POINT('Ctrl Pts',(13.8032511286279,-0.8647311392666,26.6339787839389));
#46284=CARTESIAN_POINT('Ctrl Pts',(13.8455932706301,-0.812838045508947,
26.0552206265075));
#46285=CARTESIAN_POINT('Ctrl Pts',(13.8879354126322,-0.343658628821443,
25.6395157606628));
#46286=CARTESIAN_POINT('Ctrl Pts',(13.9302775546343,0.237136846646333,25.6576957950208));
#46287=CARTESIAN_POINT('Ctrl Pts',(13.9620341611359,0.610078734339102,25.8711822034938));
#46288=CARTESIAN_POINT('Ctrl Pts',(13.9937907676375,0.837165393027052,26.2411032078405));
#46289=CARTESIAN_POINT('Ctrl Pts',(14.0255473741391,0.858689140784456,26.6723631039751));
#46290=CARTESIAN_POINT('Ctrl Pts',(14.0573039806407,0.67175373280332,27.0626203018292));
#46291=CARTESIAN_POINT('Ctrl Pts',(14.0890605871423,0.320665802654134,27.3150946682711));
#46292=CARTESIAN_POINT('Ctrl Pts',(14.1208171936439,-0.108338152284935,
27.3695156849218));
#46293=CARTESIAN_POINT('Ctrl Pts',(14.1525738001455,-0.511071607221392,
27.2112396870291));
#46294=CARTESIAN_POINT('Ctrl Pts',(14.1843304066471,-0.789162091829571,
26.8809155248763));
#46295=CARTESIAN_POINT('Ctrl Pts',(14.2160870131487,-0.874997689426164,
26.4554250429661));
#46296=CARTESIAN_POINT('Ctrl Pts',(14.2478436196503,-0.747486430903569,
26.0450557249749));
#46297=CARTESIAN_POINT('Ctrl Pts',(14.2901857616524,-0.334763101404237,
25.6360161776692));
#46298=CARTESIAN_POINT('Ctrl Pts',(14.3325279036546,0.291896647532627,25.6206077516431));
#46299=CARTESIAN_POINT('Ctrl Pts',(14.3748700456567,0.724224157529318,26.0088690323203));
#46300=CARTESIAN_POINT('Ctrl Pts',(14.4066266521583,0.871749608336183,26.4124756967386));
#46301=CARTESIAN_POINT('Ctrl Pts',(14.4383832586599,0.806929171816575,26.8416705371319));
#46302=CARTESIAN_POINT('Ctrl Pts',(14.4701398651615,0.545409067776301,27.1852627444276));
#46303=CARTESIAN_POINT('Ctrl Pts',(14.501896471663,0.150941023139775,27.3631404805124));
#46304=CARTESIAN_POINT('Ctrl Pts',(14.5336530781647,-0.28021912285405,27.3298693381627));
#46305=CARTESIAN_POINT('Ctrl Pts',(14.5654096846662,-0.64329106005797,27.0949548668723));
#46306=CARTESIAN_POINT('Ctrl Pts',(14.5971662911679,-0.84918040708807,26.7143565168844));
#46307=CARTESIAN_POINT('Ctrl Pts',(14.6289228976694,-0.848877651649225,
26.2825599466448));
#46308=CARTESIAN_POINT('Ctrl Pts',(14.6606795041711,-0.640245791566623,
25.9019254146205));
#46309=CARTESIAN_POINT('Ctrl Pts',(14.6924361106726,-0.278246720378839,
25.6703681416667));
#46310=CARTESIAN_POINT('Ctrl Pts',(14.7347782526748,0.300953418160253,25.6236659202058));
#46311=CARTESIAN_POINT('Ctrl Pts',(14.7771203946769,0.7899963704059,26.0158098368856));
#46312=CARTESIAN_POINT('Ctrl Pts',(14.819462536679,0.8702707841193,26.5913182351529));
#46313=CARTESIAN_POINT('Ctrl Pts',(14.8512191431806,0.722909344492497,26.9949848108186));
#46314=CARTESIAN_POINT('Ctrl Pts',(14.8829757496822,0.39670607213585,27.2813435458255));
#46315=CARTESIAN_POINT('Ctrl Pts',(14.9147323561838,-0.0247067925502357,
27.3754688198417));
#46316=CARTESIAN_POINT('Ctrl Pts',(14.9464889626854,-0.440950549724207,
27.2572036015918));
#46317=CARTESIAN_POINT('Ctrl Pts',(14.978245569187,-0.749147498146967,26.9538544934843));
#46318=CARTESIAN_POINT('Ctrl Pts',(15.0100021756886,-0.875315073453636,
26.5402269033167));
#46319=CARTESIAN_POINT('Ctrl Pts',(15.0417587821902,-0.787406015941745,
26.1165318185666));
#46320=CARTESIAN_POINT('Ctrl Pts',(15.0735153886918,-0.508852589467088,
25.786597948934));
#46321=CARTESIAN_POINT('Ctrl Pts',(15.1052719951934,-0.103999031099223,
25.6300620224257));
#46322=CARTESIAN_POINT('Ctrl Pts',(15.137028601695,0.322020726425784,25.6863582425199));
#46323=CARTESIAN_POINT('Ctrl Pts',(15.1793707436971,0.794949506829644,26.0239856505288));
#46324=CARTESIAN_POINT('Ctrl Pts',(15.2217128856992,0.916082953491975,26.6390194289751));
#46325=CARTESIAN_POINT('Ctrl Pts',(15.2640550277014,0.60650265839727,27.1307652361379));
#46326=CARTESIAN_POINT('Ctrl Pts',(15.295811634203,0.233647548220779,27.3444031658551));
#46327=CARTESIAN_POINT('Ctrl Pts',(15.3275682407046,-0.20032784971622,27.3530780719845));
#46328=CARTESIAN_POINT('Ctrl Pts',(15.3593248472062,-0.583188103890229,
27.1534123625965));
#46329=CARTESIAN_POINT('Ctrl Pts',(15.3910814537078,-0.825196360355749,
26.7946958574891));
#46330=CARTESIAN_POINT('Ctrl Pts',(15.4228380602093,-0.865298666620334,
26.3641173565872));
#46331=CARTESIAN_POINT('Ctrl Pts',(15.454594666711,-0.69514895411333,25.9665558949986));
#46332=CARTESIAN_POINT('Ctrl Pts',(15.4863512732125,-0.354838295545939,
25.6992841551916));
#46333=CARTESIAN_POINT('Ctrl Pts',(15.5181078797141,0.0707936362898035,
25.6265804528559));
#46334=CARTESIAN_POINT('Ctrl Pts',(15.5498644862157,0.481221379809349,25.7678566623194));
#46335=CARTESIAN_POINT('Ctrl Pts',(15.5816210927173,0.770647044230475,26.0854962111369));
#46336=CARTESIAN_POINT('Ctrl Pts',(15.6239632347195,0.914599999637588,26.6484628572205));
#46337=CARTESIAN_POINT('Ctrl Pts',(15.6663053767216,0.610781610505709,27.1967640946398));
#46338=CARTESIAN_POINT('Ctrl Pts',(15.7086475187237,0.0571294758776682,
27.373181814257));
#46339=CARTESIAN_POINT('Ctrl Pts',(15.7404041252253,-0.365640016868747,
27.2961879560505));
#46340=CARTESIAN_POINT('Ctrl Pts',(15.7721607317269,-0.703026411114089,
27.0230939777408));
#46341=CARTESIAN_POINT('Ctrl Pts',(15.8039173382285,-0.867043295741499,
26.6236608402964));
#46342=CARTESIAN_POINT('Ctrl Pts',(15.8356739447301,-0.820853184433873,
26.193414398299));
#46343=CARTESIAN_POINT('Ctrl Pts',(15.8674305512317,-0.573976477136738,
25.8383680185107));
#46344=CARTESIAN_POINT('Ctrl Pts',(15.8991871577333,-0.187633805426696,
25.6440863147334));
#46345=CARTESIAN_POINT('Ctrl Pts',(15.9309437642349,0.244824507039883,25.6590974843267));
#46346=CARTESIAN_POINT('Ctrl Pts',(15.9627003707365,0.617102793802202,25.8778604769393));
#46347=CARTESIAN_POINT('Ctrl Pts',(15.9944569772381,0.839832298393764,26.2504211670227));
#46348=CARTESIAN_POINT('Ctrl Pts',(16.0262135837397,0.856371914216354,26.6798260334447));
#46349=CARTESIAN_POINT('Ctrl Pts',(16.0685557257418,0.603560896568364,27.2030281811171));
#46350=CARTESIAN_POINT('Ctrl Pts',(16.1108978677439,0.0178602313264146,
27.426399153415));
#46351=CARTESIAN_POINT('Ctrl Pts',(16.1532400097461,-0.519146255174819,
27.2044128217892));
#46352=CARTESIAN_POINT('Ctrl Pts',(16.1849966162477,-0.792745916569997,
26.8730439586125));
#46353=CARTESIAN_POINT('Ctrl Pts',(16.2167532227493,-0.874666410284016,
26.4467823807984));
#46354=CARTESIAN_POINT('Ctrl Pts',(16.2485098292509,-0.742603575282594,
26.0356768258092));
#46355=CARTESIAN_POINT('Ctrl Pts',(16.2802664357524,-0.429966244660699,
25.7365055926741));
#46356=CARTESIAN_POINT('Ctrl Pts',(16.3120230422541,-0.0123659680828667,
25.6241844040729));
#46357=CARTESIAN_POINT('Ctrl Pts',(16.3437796487556,0.408239016411182,25.7246706589808));
#46358=CARTESIAN_POINT('Ctrl Pts',(16.3755362552572,0.729198256444399,26.0148959050765));
#46359=CARTESIAN_POINT('Ctrl Pts',(16.4072928617588,0.872815239109643,26.4221090335752));
#46360=CARTESIAN_POINT('Ctrl Pts',(16.4390494682604,0.802962095894506,26.8505135601548));
#46361=CARTESIAN_POINT('Ctrl Pts',(16.470806074762,0.538827077444582,27.1894749004682));
#46362=CARTESIAN_POINT('Ctrl Pts',(16.5131482167641,0.00830202667944394,
27.4265341092826));
#46363=CARTESIAN_POINT('Ctrl Pts',(16.5554903587663,-0.583471617801813,
27.2197883373124));
#46364=CARTESIAN_POINT('Ctrl Pts',(16.5978325007684,-0.850953485318723,
26.7039323995519));
#46365=CARTESIAN_POINT('Ctrl Pts',(16.62958910727,-0.846543901799235,26.2742317435461));
#46366=CARTESIAN_POINT('Ctrl Pts',(16.6613457137716,-0.634421735364911,
25.8955312200211));
#46367=CARTESIAN_POINT('Ctrl Pts',(16.6931023202732,-0.268468213163799,
25.6663448562902));
#46368=CARTESIAN_POINT('Ctrl Pts',(16.7248589267748,0.163393894573562,25.639130023301));
#46369=CARTESIAN_POINT('Ctrl Pts',(16.7566155332764,0.55506773558983,25.8224266208424));
#46370=CARTESIAN_POINT('Ctrl Pts',(16.788372139778,0.811870096428448,26.1703613674176));
#46371=CARTESIAN_POINT('Ctrl Pts',(16.8201287462796,0.870188994142449,26.5991322076148));
#46372=CARTESIAN_POINT('Ctrl Pts',(16.8518853527812,0.717514735853032,27.0030368257953));
#46373=CARTESIAN_POINT('Ctrl Pts',(16.8836419592828,0.387973130305122,27.2855474100631));
#46374=CARTESIAN_POINT('Ctrl Pts',(16.9153985657844,-0.0324540553306391,
27.3744466776518));
#46375=CARTESIAN_POINT('Ctrl Pts',(16.9577407077865,-0.590866308020062,
27.213730611194));
#46376=CARTESIAN_POINT('Ctrl Pts',(17.0000828497886,-0.910043839361548,
26.6742256862701));
#46377=CARTESIAN_POINT('Ctrl Pts',(17.0424249917908,-0.782042573269087,
26.1074192167792));
#46378=CARTESIAN_POINT('Ctrl Pts',(17.0741815982923,-0.501700239207807,
25.7817349004191));
#46379=CARTESIAN_POINT('Ctrl Pts',(17.105938204794,-0.0954247742663506,
25.6289273527781));
#46380=CARTESIAN_POINT('Ctrl Pts',(17.1376948112956,0.332090138521344,25.6895851556312));
#46381=CARTESIAN_POINT('Ctrl Pts',(17.1694514177971,0.679811052822366,25.9471423201995));
#46382=CARTESIAN_POINT('Ctrl Pts',(17.2012080242988,0.861117338127211,26.3397414431271));
#46383=CARTESIAN_POINT('Ctrl Pts',(17.2329646308003,0.833187592663935,26.7712805138921));
#46384=CARTESIAN_POINT('Ctrl Pts',(17.2647212373019,0.601403494523231,27.1366866707663));
#46385=CARTESIAN_POINT('Ctrl Pts',(17.2964778438035,0.224333048232079,27.3470821255804));
#46386=CARTESIAN_POINT('Ctrl Pts',(17.3282344503051,-0.209714273666674,
27.350663157861));
#46387=CARTESIAN_POINT('Ctrl Pts',(17.3599910568068,-0.588452413422316,
27.1476372528845));
#46388=CARTESIAN_POINT('Ctrl Pts',(17.4023331988088,-0.911792823819409,
26.6648278932385));
#46389=CARTESIAN_POINT('Ctrl Pts',(17.444675340811,-0.808071974758552,26.0466193062064));
#46390=CARTESIAN_POINT('Ctrl Pts',(17.4870174828131,-0.344864013488189,
25.6957742430468));
#46391=CARTESIAN_POINT('Ctrl Pts',(17.5187740893147,0.0793965318800745,
25.6274725805664));
#46392=CARTESIAN_POINT('Ctrl Pts',(17.5505306958163,0.48850813612692,25.7725158616459));
#46393=CARTESIAN_POINT('Ctrl Pts',(17.5822873023179,0.776265705627514,26.0944537106846));
#46394=CARTESIAN_POINT('Ctrl Pts',(17.6140439088195,0.876101723455108,26.5154980733855));
#46395=CARTESIAN_POINT('Ctrl Pts',(17.6458005153211,0.761662875423693,26.9325226470832));
#46396=CARTESIAN_POINT('Ctrl Pts',(17.6775571218227,0.462152454421897,27.2444526346239));
#46397=CARTESIAN_POINT('Ctrl Pts',(17.7093137283243,0.0494151738932063,
27.3744217314534));
#46398=CARTESIAN_POINT('Ctrl Pts',(17.7410703348259,-0.37449007535567,27.29223335565));
#46399=CARTESIAN_POINT('Ctrl Pts',(17.7728269413275,-0.708642640693063,
27.015195558281));
#46400=CARTESIAN_POINT('Ctrl Pts',(17.8045835478291,-0.867352034794116,
26.6158557264595));
#46401=CARTESIAN_POINT('Ctrl Pts',(17.8469256898312,-0.803337221972986,
26.0382991332051));
#46402=CARTESIAN_POINT('Ctrl Pts',(17.8892678318333,-0.325602990091037,
25.6325271546952));
#46403=CARTESIAN_POINT('Ctrl Pts',(17.9316099738355,0.254746860080869,25.6628246699476));
#46404=CARTESIAN_POINT('Ctrl Pts',(17.9633665803371,0.623033274293027,25.8841264013226));
#46405=CARTESIAN_POINT('Ctrl Pts',(17.9951231868387,0.842539849663937,26.2586048773553));
#46406=CARTESIAN_POINT('Ctrl Pts',(18.0268797933403,0.854628194489789,26.6904393272496));
#46407=CARTESIAN_POINT('Ctrl Pts',(18.0586363998418,0.660333792873029,27.0762848995925));
#46408=CARTESIAN_POINT('Ctrl Pts',(18.0903930063434,0.302597639953616,27.3221346718869));
#46409=CARTESIAN_POINT('Ctrl Pts',(18.122149612845,-0.124805809017264,27.366130478626));
#46410=CARTESIAN_POINT('Ctrl Pts',(18.1644917548472,-0.66311189802541,27.1471545836929));
#46411=CARTESIAN_POINT('Ctrl Pts',(18.2068338968493,-0.923363074658378,
26.5769351347813));
#46412=CARTESIAN_POINT('Ctrl Pts',(18.2491760388514,-0.73610041458287,26.0268422237077));
#46413=CARTESIAN_POINT('Ctrl Pts',(18.280932645353,-0.422853630327345,25.7326697824275));
#46414=CARTESIAN_POINT('Ctrl Pts',(18.3126892518546,-0.00268997678121585,
25.6237184982157));
#46415=CARTESIAN_POINT('Ctrl Pts',(18.3444458583562,0.416004918794958,25.7292892037947));
#46416=CARTESIAN_POINT('Ctrl Pts',(18.3762024648578,0.734509914179396,26.0222031788523));
#46417=CARTESIAN_POINT('Ctrl Pts',(18.4079590713594,0.873242998764314,26.4317882623911));
#46418=CARTESIAN_POINT('Ctrl Pts',(18.439715677861,0.799792930977031,26.857946487172));
#46419=CARTESIAN_POINT('Ctrl Pts',(18.4714722843626,0.530634059378337,27.1967666277446));
#46420=CARTESIAN_POINT('Ctrl Pts',(18.5032288908642,0.133412098705898,27.3660684629623));
#46421=CARTESIAN_POINT('Ctrl Pts',(18.5349854973658,-0.298575946972933,
27.323687022374));
#46422=CARTESIAN_POINT('Ctrl Pts',(18.5667421038674,-0.653696947944898,
27.0817134657145));
#46423=CARTESIAN_POINT('Ctrl Pts',(18.6090842458695,-0.924117259356119,
26.5673918456129));
#46424=CARTESIAN_POINT('Ctrl Pts',(18.6514263878717,-0.755543837880523,
25.9636345490257));
#46425=CARTESIAN_POINT('Ctrl Pts',(18.6937685298738,-0.257802194059594,
25.663789331015));
#46426=CARTESIAN_POINT('Ctrl Pts',(18.7255251363754,0.171304517422399,25.6407778825982));
#46427=CARTESIAN_POINT('Ctrl Pts',(18.757281742877,0.562765663228658,25.828309407318));
#46428=CARTESIAN_POINT('Ctrl Pts',(18.7890383493786,0.814830607180771,26.1788969611515));
#46429=CARTESIAN_POINT('Ctrl Pts',(18.8207949558802,0.869539941123068,26.6081432965023));
#46430=CARTESIAN_POINT('Ctrl Pts',(18.8525515623818,0.711602884148318,27.0107124536822));
#46431=CARTESIAN_POINT('Ctrl Pts',(18.8843081688833,0.380759120484664,27.2891876670486));
#46432=CARTESIAN_POINT('Ctrl Pts',(18.916064775385,-0.0434180107468701,
27.3747405080475));
#46433=CARTESIAN_POINT('Ctrl Pts',(18.9478213818865,-0.456239530951512,
27.2481436591185));
#46434=CARTESIAN_POINT('Ctrl Pts',(18.9795779883882,-0.759197243098779,
26.9372955858094));
#46435=CARTESIAN_POINT('Ctrl Pts',(19.0113345948897,-0.874735896034552,
26.5233959387116));
#46436=CARTESIAN_POINT('Ctrl Pts',(19.0536767368919,-0.749970179761652,
25.9558684820887));
#46437=CARTESIAN_POINT('Ctrl Pts',(19.096018878894,-0.231925562864532,25.602924243668));
#46438=CARTESIAN_POINT('Ctrl Pts',(19.1383610208961,0.341892025666602,25.6945063001182));
#46439=CARTESIAN_POINT('Ctrl Pts',(19.1701176273977,0.684796943888501,25.953501117168));
#46440=CARTESIAN_POINT('Ctrl Pts',(19.2018742338993,0.863210918198414,26.3492009450444));
#46441=CARTESIAN_POINT('Ctrl Pts',(19.2336308404009,0.829949279037307,26.7797146301835));
#46442=CARTESIAN_POINT('Ctrl Pts',(19.2653874469025,0.595099009571776,27.143157718116));
#46443=CARTESIAN_POINT('Ctrl Pts',(19.2971440534041,0.214865696983258,27.3491399222129));
#46444=CARTESIAN_POINT('Ctrl Pts',(19.3289006599057,-0.217576116898816,
27.3487963919108));
#46445=CARTESIAN_POINT('Ctrl Pts',(19.3606572664073,-0.597024274205395,
27.1407948939579));
#46446=CARTESIAN_POINT('Ctrl Pts',(19.3924138729089,-0.831045770920826,
26.7779143229616));
#46447=CARTESIAN_POINT('Ctrl Pts',(19.4241704794105,-0.862308843996473,
26.3449795469586));
#46448=CARTESIAN_POINT('Ctrl Pts',(19.4559270859121,-0.683857455778086,
25.954061140841));
#46449=CARTESIAN_POINT('Ctrl Pts',(19.4982692279142,-0.222658482913689,
25.6005793090563));
#46450=CARTESIAN_POINT('Ctrl Pts',(19.5406113699163,0.400907586751457,25.6646512786888));
#46451=CARTESIAN_POINT('Ctrl Pts',(19.5829535119185,0.780587626055508,26.1045341787056));
#46452=CARTESIAN_POINT('Ctrl Pts',(19.6147101184201,0.875815152337618,26.5235733373014));
#46453=CARTESIAN_POINT('Ctrl Pts',(19.6464667249217,0.757165946501871,26.9411044929839));
#46454=CARTESIAN_POINT('Ctrl Pts',(19.6782233314233,0.454240791570915,27.2488133167793));
#46455=CARTESIAN_POINT('Ctrl Pts',(19.7099799379249,0.0404230551237811,
27.3753060368695));
#46456=CARTESIAN_POINT('Ctrl Pts',(19.7417365444265,-0.38305279380198,27.2877032641777));
#46457=CARTESIAN_POINT('Ctrl Pts',(19.7734931509281,-0.713453700745531,
27.0087027604192));
#46458=CARTESIAN_POINT('Ctrl Pts',(19.8052497574296,-0.86948889817834,26.6050958422474));
#46459=CARTESIAN_POINT('Ctrl Pts',(19.8370063639313,-0.814508508394085,
26.1768137780997));
#46460=CARTESIAN_POINT('Ctrl Pts',(19.8687629704328,-0.559355008981932,
25.8256633947185));
#46461=CARTESIAN_POINT('Ctrl Pts',(19.9005195769344,-0.170947207752905,
25.641811611635));
#46462=CARTESIAN_POINT('Ctrl Pts',(19.9428617189366,0.409504178357161,25.6688317214792));
#46463=CARTESIAN_POINT('Ctrl Pts',(19.9852038609387,0.844951400494168,26.1197480965017));
#46464=CARTESIAN_POINT('Ctrl Pts',(20.0275460029408,0.851700710212036,26.7007888392998));
#46465=CARTESIAN_POINT('Ctrl Pts',(20.0593026094424,0.65440773846806,27.0825447580477));
#46466=CARTESIAN_POINT('Ctrl Pts',(20.091059215944,0.294567841588426,27.3252897860598));
#46467=CARTESIAN_POINT('Ctrl Pts',(20.1228158224456,-0.135371897765222,
27.3652921641899));
#46468=CARTESIAN_POINT('Ctrl Pts',(20.1545724289472,-0.533288312928303,
27.1952684782584));
#46469=CARTESIAN_POINT('Ctrl Pts',(20.1863290354488,-0.800589857703777,
26.8553333012505));
#46470=CARTESIAN_POINT('Ctrl Pts',(20.2180856419504,-0.873362460873776,
26.4290585205815));
#46471=CARTESIAN_POINT('Ctrl Pts',(20.249842248452,-0.73250696373832,26.0199066463822));
#46472=CARTESIAN_POINT('Ctrl Pts',(20.2815988549536,-0.414415220875257,
25.7279031997349));
#46473=CARTESIAN_POINT('Ctrl Pts',(20.3133554614552,0.0070018250111366,
25.6238956353595));
#46474=CARTESIAN_POINT('Ctrl Pts',(20.3451120679568,0.422462913279715,25.7336871757133));
#46475=CARTESIAN_POINT('Ctrl Pts',(20.3874542099589,0.848829326883048,26.1284853258155));
#46476=CARTESIAN_POINT('Ctrl Pts',(20.429796351961,0.891103483033206,26.7539073883077));
#46477=CARTESIAN_POINT('Ctrl Pts',(20.4721384939632,0.52174378033525,27.202491057199));
#46478=CARTESIAN_POINT('Ctrl Pts',(20.5038951004647,0.124836532195944,27.3671930139969));
#46479=CARTESIAN_POINT('Ctrl Pts',(20.5356517069664,-0.306743695101083,
27.320842097963));
#46480=CARTESIAN_POINT('Ctrl Pts',(20.5674083134679,-0.661237300894562,
27.0743007156697));
#46481=CARTESIAN_POINT('Ctrl Pts',(20.5991649199696,-0.855871616173788,
26.6878256057987));
#46482=CARTESIAN_POINT('Ctrl Pts',(20.6309215264711,-0.841125257036995,
26.2556351555354));
#46483=CARTESIAN_POINT('Ctrl Pts',(20.6626781329728,-0.622000583043283,
25.8828209690378));
#46484=CARTESIAN_POINT('Ctrl Pts',(20.6944347394743,-0.250583931206579,
25.6607957498117));
#46485=CARTESIAN_POINT('Ctrl Pts',(20.7261913459759,0.180828213237544,25.6425767663691));
#46486=CARTESIAN_POINT('Ctrl Pts',(20.7579479524775,0.570061465492677,25.8346896898018));
#46487=CARTESIAN_POINT('Ctrl Pts',(20.7897045589791,0.816933190155719,26.186423182322));
#46488=CARTESIAN_POINT('Ctrl Pts',(20.8320467009813,0.888436609774976,26.7630870002921));
#46489=CARTESIAN_POINT('Ctrl Pts',(20.8743888429834,0.517630593842114,27.2685004538904));
#46490=CARTESIAN_POINT('Ctrl Pts',(20.9167309849855,-0.0539048377036311,
27.3733868136372));
#46491=CARTESIAN_POINT('Ctrl Pts',(20.9484875914871,-0.463520805306752,
27.24347585458));
#46492=CARTESIAN_POINT('Ctrl Pts',(20.9802441979887,-0.763608131273106,
26.9298558666882));
#46493=CARTESIAN_POINT('Ctrl Pts',(21.0120008044903,-0.875722837400207,
26.5128682620743));
#46494=CARTESIAN_POINT('Ctrl Pts',(21.0437574109919,-0.775420805447384,
26.0919347404582));
#46495=CARTESIAN_POINT('Ctrl Pts',(21.0755140174935,-0.485570674761989,
25.7710096056552));
#46496=CARTESIAN_POINT('Ctrl Pts',(21.1072706239951,-0.0777356001915541,
25.6272160301493));
#46497=CARTESIAN_POINT('Ctrl Pts',(21.1390272304967,0.349340295407205,25.6968702233649));
#46498=CARTESIAN_POINT('Ctrl Pts',(21.1707838369983,0.690918760718671,25.9610151111955));
#46499=CARTESIAN_POINT('Ctrl Pts',(21.2025404434999,0.864676384461559,26.3587816107931));
#46500=CARTESIAN_POINT('Ctrl Pts',(21.2342970500015,0.826705647584722,26.7868240401616));
#46501=CARTESIAN_POINT('Ctrl Pts',(21.2766391920036,0.509674764547415,27.2737997245377));
#46502=CARTESIAN_POINT('Ctrl Pts',(21.3189813340057,-0.0995970639515039,
27.421202911504));
#46503=CARTESIAN_POINT('Ctrl Pts',(21.3613234760079,-0.604169405036641,
27.1330004642816));
#46504=CARTESIAN_POINT('Ctrl Pts',(21.3930800825095,-0.833603937258024,
26.7696522929322));
#46505=CARTESIAN_POINT('Ctrl Pts',(21.4248366890111,-0.860885778032424,
26.3364484134772));
#46506=CARTESIAN_POINT('Ctrl Pts',(21.4565932955127,-0.677826223140756,
25.9453760811723));
#46507=CARTESIAN_POINT('Ctrl Pts',(21.4883499020142,-0.329820559486764,
25.6882037939819));
#46508=CARTESIAN_POINT('Ctrl Pts',(21.5201065085159,0.0986415040206994,
25.6296691842062));
#46509=CARTESIAN_POINT('Ctrl Pts',(21.5518631150174,0.503135455528145,25.7826093149782));
#46510=CARTESIAN_POINT('Ctrl Pts',(21.5836197215191,0.784758474883268,26.1111424216863));
#46511=CARTESIAN_POINT('Ctrl Pts',(21.6153763280206,0.875652297533056,26.533264066163));
#46512=CARTESIAN_POINT('Ctrl Pts',(21.6471329345222,0.752110981173881,26.949373959296));
#46513=CARTESIAN_POINT('Ctrl Pts',(21.6788895410238,0.447178387750749,27.2521580600457));
#46514=CARTESIAN_POINT('Ctrl Pts',(21.721231683026,-0.109095410505965,27.4201263884477));
#46515=CARTESIAN_POINT('Ctrl Pts',(21.7635738250281,-0.669923979080759,
27.1401064298722));
#46516=CARTESIAN_POINT('Ctrl Pts',(21.8059159670302,-0.869927655947503,
26.5945311122369));
#46517=CARTESIAN_POINT('Ctrl Pts',(21.8376725735318,-0.811138913729804,
26.1688481527623));
#46518=CARTESIAN_POINT('Ctrl Pts',(21.8694291800334,-0.552768117570983,
25.8200581992041));
#46519=CARTESIAN_POINT('Ctrl Pts',(21.901185786535,-0.160737937948536,25.6390590058447));
#46520=CARTESIAN_POINT('Ctrl Pts',(21.9329423930366,0.271093794863995,25.6667516360942));
#46521=CARTESIAN_POINT('Ctrl Pts',(21.9646989995382,0.63640291796604,25.8981717842771));
#46522=CARTESIAN_POINT('Ctrl Pts',(21.9964556060398,0.847077573899532,26.2758253686028));
#46523=CARTESIAN_POINT('Ctrl Pts',(22.0282122125414,0.850630065093437,26.7085295481993));
#46524=CARTESIAN_POINT('Ctrl Pts',(22.059968819043,0.648036901149478,27.0898488103076));
#46525=CARTESIAN_POINT('Ctrl Pts',(22.0917254255446,0.285372852470821,27.3283539209591));
#46526=CARTESIAN_POINT('Ctrl Pts',(22.1234820320462,-0.142927353585185,
27.3632971848444));
#46527=CARTESIAN_POINT('Ctrl Pts',(22.1658241740483,-0.676492025225343,
27.1331610530644));
#46528=CARTESIAN_POINT('Ctrl Pts',(22.2081663160505,-0.924780428505825,
26.5575807117335));
#46529=CARTESIAN_POINT('Ctrl Pts',(22.2505084580525,-0.726032735274209,
26.0115465988722));
#46530=CARTESIAN_POINT('Ctrl Pts',(22.2822650645542,-0.406704623753999,
25.7239850308707));
#46531=CARTESIAN_POINT('Ctrl Pts',(22.3140216710558,0.0156507426113821,
25.6238558916889));
#46532=CARTESIAN_POINT('Ctrl Pts',(22.3457782775574,0.43204262535938,25.7381632392791));
#46533=CARTESIAN_POINT('Ctrl Pts',(22.377534884059,0.744348760409762,26.0376801924619));
#46534=CARTESIAN_POINT('Ctrl Pts',(22.4092914905605,0.874479097205011,26.4500782233159));
#46535=CARTESIAN_POINT('Ctrl Pts',(22.4410480970622,0.792126735651671,26.8746063483597));
#46536=CARTESIAN_POINT('Ctrl Pts',(22.4728047035637,0.515935813272952,27.2077190944827));
#46537=CARTESIAN_POINT('Ctrl Pts',(22.5045613100654,0.115257770696188,27.3686708758596));
#46538=CARTESIAN_POINT('Ctrl Pts',(22.5363179165669,-0.315748742833674,
27.3172579853967));
#46539=CARTESIAN_POINT('Ctrl Pts',(22.5680745230685,-0.665727907757558,
27.0679054592059));
#46540=CARTESIAN_POINT('Ctrl Pts',(22.6104166650707,-0.925325249310694,
26.5480370929518));
#46541=CARTESIAN_POINT('Ctrl Pts',(22.6527588070727,-0.744153268499322,
25.9479399558989));
#46542=CARTESIAN_POINT('Ctrl Pts',(22.6951009490749,-0.240245462236218,
25.6585771719059));
#46543=CARTESIAN_POINT('Ctrl Pts',(22.7268575555765,0.189248855064349,25.6445511387859));
#46544=CARTESIAN_POINT('Ctrl Pts',(22.7586141620781,0.576699591845642,25.8402341134632));
#46545=CARTESIAN_POINT('Ctrl Pts',(22.7903707685797,0.821372211418811,26.1960201151029));
#46546=CARTESIAN_POINT('Ctrl Pts',(22.8221273750813,0.867086268116494,26.6263173986805));
#46547=CARTESIAN_POINT('Ctrl Pts',(22.8538839815829,0.700758808996464,27.0254930702204));
#46548=CARTESIAN_POINT('Ctrl Pts',(22.8856405880845,0.364159558242971,27.2969833735442));
#46549=CARTESIAN_POINT('Ctrl Pts',(22.9173971945861,-0.0617151267228295,
27.3736402710765));
#46550=CARTESIAN_POINT('Ctrl Pts',(22.9491538010877,-0.471796805528492,
27.2384315936942));
#46551=CARTESIAN_POINT('Ctrl Pts',(22.9809104075893,-0.768182716769667,
26.9213112827258));
#46552=CARTESIAN_POINT('Ctrl Pts',(23.0126670140909,-0.87503394665564,26.5050842859195));
#46553=CARTESIAN_POINT('Ctrl Pts',(23.055009156093,-0.738418305193021,25.9402922317253));
#46554=CARTESIAN_POINT('Ctrl Pts',(23.0973512980951,-0.213100708746876,
25.5982669645384));
#46555=CARTESIAN_POINT('Ctrl Pts',(23.1396934400973,0.358674569475328,25.7018378542084));
#46556=CARTESIAN_POINT('Ctrl Pts',(23.1714500465988,0.696084125988342,25.9679522833028));
#46557=CARTESIAN_POINT('Ctrl Pts',(23.2032066531005,0.866177793525835,26.3672993056713));
#46558=CARTESIAN_POINT('Ctrl Pts',(23.234963259602,0.823913621290959,26.7970225997534));
#46559=CARTESIAN_POINT('Ctrl Pts',(23.2667198661037,0.581508627612291,27.155471126426));
#46560=CARTESIAN_POINT('Ctrl Pts',(23.2984764726053,0.197047783445193,27.3534506700888));
#46561=CARTESIAN_POINT('Ctrl Pts',(23.3302330791068,-0.235292129374152,
27.3440570451221));
#46562=CARTESIAN_POINT('Ctrl Pts',(23.3619896856085,-0.610304112860864,
27.1281599875336));
#46563=CARTESIAN_POINT('Ctrl Pts',(23.39374629211,-0.836679967375603,26.7604612763252));
#46564=CARTESIAN_POINT('Ctrl Pts',(23.4255028986117,-0.858875706694659,
26.3269670443371));
#46565=CARTESIAN_POINT('Ctrl Pts',(23.4572595051132,-0.672282236796609,
25.9398688976223));
#46566=CARTESIAN_POINT('Ctrl Pts',(23.4996016471154,-0.203786583491818,
25.596116485547));
#46567=CARTESIAN_POINT('Ctrl Pts',(23.5419437891175,0.418302013008299,25.6732244529351));
#46568=CARTESIAN_POINT('Ctrl Pts',(23.5842859311196,0.788692998912709,26.1209569797119));
#46569=CARTESIAN_POINT('Ctrl Pts',(23.6160425376212,0.875129990573807,26.5418972898167));
#46570=CARTESIAN_POINT('Ctrl Pts',(23.6477991441228,0.747768652106043,26.9568539013734));
#46571=CARTESIAN_POINT('Ctrl Pts',(23.6795557506244,0.438470092684962,27.2581556950481));
#46572=CARTESIAN_POINT('Ctrl Pts',(23.711312357126,0.0220957411812786,27.3759603071985));
#46573=CARTESIAN_POINT('Ctrl Pts',(23.7430689636276,-0.399454003372334,
27.279514191292));
#46574=CARTESIAN_POINT('Ctrl Pts',(23.7748255701292,-0.723943606895722,
26.9936601417984));
#46575=CARTESIAN_POINT('Ctrl Pts',(23.8065821766308,-0.87149791877326,26.5868761053855));
#46576=CARTESIAN_POINT('Ctrl Pts',(23.8383387831324,-0.807566456174055,
26.1598384749342));
#46577=CARTESIAN_POINT('Ctrl Pts',(23.870095389634,-0.545119941785172,25.8141048678086));
#46578=CARTESIAN_POINT('Ctrl Pts',(23.9018519961356,-0.152949546185258,
25.638421974465));
#46579=CARTESIAN_POINT('Ctrl Pts',(23.9441941381377,0.426809233249918,25.6775838901603));
#46580=CARTESIAN_POINT('Ctrl Pts',(23.9865362801398,0.852724278817119,26.1375145746006));
#46581=CARTESIAN_POINT('Ctrl Pts',(24.028878422142,0.847312052549233,26.718569310215));
#46582=CARTESIAN_POINT('Ctrl Pts',(24.0606350286435,0.642072878853147,27.096112658427));
#46583=CARTESIAN_POINT('Ctrl Pts',(24.0923916351452,0.27723160918528,27.3312737690684));
#46584=CARTESIAN_POINT('Ctrl Pts',(24.1241482416467,-0.153451138848596,
27.3622695797134));
#46585=CARTESIAN_POINT('Ctrl Pts',(24.1559048481484,-0.547722137425273,
27.1839555115209));
#46586=CARTESIAN_POINT('Ctrl Pts',(24.1876614546499,-0.807850953810988,
26.8385006819232));
#46587=CARTESIAN_POINT('Ctrl Pts',(24.2194180611516,-0.871686512784537,
26.4107962725267));
#46588=CARTESIAN_POINT('Ctrl Pts',(24.2511746676531,-0.722299108686334,
26.0046818419399));
#46589=CARTESIAN_POINT('Ctrl Pts',(24.2829312741547,-0.398165966193382,
25.719399393007));
#46590=CARTESIAN_POINT('Ctrl Pts',(24.3146878806563,0.0253354596048242,
25.6242340507976));
#46591=CARTESIAN_POINT('Ctrl Pts',(24.3464444871579,0.438407830914415,25.7426963412501));
#46592=CARTESIAN_POINT('Ctrl Pts',(24.3887866291601,0.856418502585246,26.1463310478134));
#46593=CARTESIAN_POINT('Ctrl Pts',(24.4311287711621,0.885594527149535,26.7725008491618));
#46594=CARTESIAN_POINT('Ctrl Pts',(24.4734709131644,0.506927732427945,27.2132562876404));
#46595=CARTESIAN_POINT('Ctrl Pts',(24.5052275196659,0.106660520219594,27.3696156718471));
#46596=CARTESIAN_POINT('Ctrl Pts',(24.5369841261675,-0.323855149208574,
27.3142427688372));
#46597=CARTESIAN_POINT('Ctrl Pts',(24.5687407326691,-0.67311148146482,27.0603365182043));
#46598=CARTESIAN_POINT('Ctrl Pts',(24.6004973391707,-0.859614992946161,
26.6698727331497));
#46599=CARTESIAN_POINT('Ctrl Pts',(24.6322539456723,-0.835826954147192,
26.2380855522183));
#46600=CARTESIAN_POINT('Ctrl Pts',(24.6640105521739,-0.608947992835266,
25.8699388731341));
#46601=CARTESIAN_POINT('Ctrl Pts',(24.6957671586755,-0.232966129185645,
25.655735312378));
#46602=CARTESIAN_POINT('Ctrl Pts',(24.7275237651771,0.198732817183121,25.6465489400985));
#46603=CARTESIAN_POINT('Ctrl Pts',(24.7592803716787,0.583860269629324,25.8467656861094));
#46604=CARTESIAN_POINT('Ctrl Pts',(24.7910369781803,0.823316824457635,26.2035886906205));
#46605=CARTESIAN_POINT('Ctrl Pts',(24.8333791201824,0.882736126473029,26.7816226381713));
#46606=CARTESIAN_POINT('Ctrl Pts',(24.8757212621845,0.501433997917763,27.2791651461939));
#46607=CARTESIAN_POINT('Ctrl Pts',(24.9180634041867,-0.0721713267102057,
27.3720674041403));
#46608=CARTESIAN_POINT('Ctrl Pts',(24.9498200106883,-0.478978797049014,
27.233612428516));
#46609=CARTESIAN_POINT('Ctrl Pts',(24.9815766171899,-0.77243693997653,26.913780881666));
#46610=CARTESIAN_POINT('Ctrl Pts',(25.0133332236915,-0.875800347974294,
26.4945382602418));
#46611=CARTESIAN_POINT('Ctrl Pts',(25.045089830193,-0.766710960134842,26.0757960570967));
#46612=CARTESIAN_POINT('Ctrl Pts',(25.0768464366946,-0.470207969519981,
25.7610072120543));
#46613=CARTESIAN_POINT('Ctrl Pts',(25.1086030431962,-0.0594528961875975,
25.6257803281209));
#46614=CARTESIAN_POINT('Ctrl Pts',(25.1403596496979,0.366071735589218,25.7043571375826));
#46615=CARTESIAN_POINT('Ctrl Pts',(25.1721162561994,0.70204734869645,25.9755927494199));
#46616=CARTESIAN_POINT('Ctrl Pts',(25.2038728627011,0.867442434043655,26.3769085424732));
#46617=CARTESIAN_POINT('Ctrl Pts',(25.2356294692026,0.820521914059242,26.8040625697314));
#46618=CARTESIAN_POINT('Ctrl Pts',(25.2779716112048,0.493369007601602,27.2842967561129));
#46619=CARTESIAN_POINT('Ctrl Pts',(25.3203137532069,-0.118854243983667,
27.4189167796913));
#46620=CARTESIAN_POINT('Ctrl Pts',(25.362655895209,-0.617284556472856,27.120217731207));
#46621=CARTESIAN_POINT('Ctrl Pts',(25.3944125017106,-0.839064665140981,
26.7521475183433));
#46622=CARTESIAN_POINT('Ctrl Pts',(25.4261691082122,-0.857274412299222,
26.3184675613251));
#46623=CARTESIAN_POINT('Ctrl Pts',(25.4579257147138,-0.666070563609887,
25.9313119621416));
#46624=CARTESIAN_POINT('Ctrl Pts',(25.4896823212154,-0.312759000685908,
25.6814790845327));
#46625=CARTESIAN_POINT('Ctrl Pts',(25.521438927717,0.116834238873859,25.6319241762008));
#46626=CARTESIAN_POINT('Ctrl Pts',(25.5531955342186,0.51803885892464,25.7932960859057));
#46627=CARTESIAN_POINT('Ctrl Pts',(25.5849521407202,0.792724636550138,26.1276510631719));
#46628=CARTESIAN_POINT('Ctrl Pts',(25.6167087472218,0.874764363200845,26.5515824880205));
#46629=CARTESIAN_POINT('Ctrl Pts',(25.6484653537234,0.742541730057994,26.9650157659));
#46630=CARTESIAN_POINT('Ctrl Pts',(25.680221960225,0.431339236497572,27.2613519033306));
#46631=CARTESIAN_POINT('Ctrl Pts',(25.7225641022271,-0.128327980376764,
27.4176417103926));
#46632=CARTESIAN_POINT('Ctrl Pts',(25.7649062442292,-0.683173443957012,
27.1259460245806));
#46633=CARTESIAN_POINT('Ctrl Pts',(25.8072483862314,-0.871715480323669,
26.5763045068337));
#46634=CARTESIAN_POINT('Ctrl Pts',(25.8390049927329,-0.804030896026743,
26.1519451133608));
#46635=CARTESIAN_POINT('Ctrl Pts',(25.8707615992346,-0.538417183932629,
25.8086387506637));
#46636=CARTESIAN_POINT('Ctrl Pts',(25.9025182057361,-0.142684911729077,
25.6358836320594));
#46637=CARTESIAN_POINT('Ctrl Pts',(25.9342748122378,0.288472707472188,25.67260759849));
#46638=CARTESIAN_POINT('Ctrl Pts',(25.9660314187393,0.648858613252514,25.9116222761151));
#46639=CARTESIAN_POINT('Ctrl Pts',(25.997788025241,0.85158363238984,26.2936021581678));
#46640=CARTESIAN_POINT('Ctrl Pts',(26.0295446317425,0.846079566586723,26.7262859206823));
#46641=CARTESIAN_POINT('Ctrl Pts',(26.0613012382441,0.635550722694575,27.1032817752238));
#46642=CARTESIAN_POINT('Ctrl Pts',(26.0930578447457,0.267974236077588,27.3341448116203));
#46643=CARTESIAN_POINT('Ctrl Pts',(26.1248144512473,-0.16096270354682,27.3601168946639));
#46644=CARTESIAN_POINT('Ctrl Pts',(26.1671565932494,-0.689595797064967,
27.1188647612773));
#46645=CARTESIAN_POINT('Ctrl Pts',(26.2094987352516,-0.925780813951623,
26.53821414226));
#46646=CARTESIAN_POINT('Ctrl Pts',(26.2518408772537,-0.715653941089743,
25.9964592341892));
#46647=CARTESIAN_POINT('Ctrl Pts',(26.2835974837553,-0.390369588230022,
25.7156432068259));
#46648=CARTESIAN_POINT('Ctrl Pts',(26.3153540902569,0.0339726758359866,
25.6243757953063));
#46649=CARTESIAN_POINT('Ctrl Pts',(26.3471106967585,0.447912024032863,25.7473709970866));
#46650=CARTESIAN_POINT('Ctrl Pts',(26.3788673032601,0.753822864844703,26.0533610271208));
#46651=CARTESIAN_POINT('Ctrl Pts',(26.4106239097617,0.87540473357552,26.4683863005388));
#46652=CARTESIAN_POINT('Ctrl Pts',(26.4423805162633,0.783976936688825,26.8911144898655));
#46653=CARTESIAN_POINT('Ctrl Pts',(26.4635515872644,0.595505398658813,27.1092393365905));
#46654=CARTESIAN_POINT('Ctrl Pts',(26.4741371227649,0.480906627467731,27.1892031454205));
#46655=CARTESIAN_POINT('Ctrl Pts',(9.60000000000002,0.662150216245817,26.1181780341239));
#46656=CARTESIAN_POINT('Ctrl Pts',(9.61058553550055,0.725638504704611,26.2282785199239));
#46657=CARTESIAN_POINT('Ctrl Pts',(9.63175660650163,0.796605391005151,26.480675629033));
#46658=CARTESIAN_POINT('Ctrl Pts',(9.6635132130032,0.708650864432033,26.8640803773426));
#46659=CARTESIAN_POINT('Ctrl Pts',(9.69526981950482,0.448266436304386,27.1588859127484));
#46660=CARTESIAN_POINT('Ctrl Pts',(9.7270264260064,0.0782001173243299,27.2927247256205));
#46661=CARTESIAN_POINT('Ctrl Pts',(9.75878303250801,-0.310157515624281,
27.2341585395261));
#46662=CARTESIAN_POINT('Ctrl Pts',(9.7905396390096,-0.624341483803593,26.9951389225185));
#46663=CARTESIAN_POINT('Ctrl Pts',(9.82229624551119,-0.783759014765585,
26.6382863941097));
#46664=CARTESIAN_POINT('Ctrl Pts',(9.86463838751332,-0.747584602748986,
26.1110311207911));
#46665=CARTESIAN_POINT('Ctrl Pts',(9.90698052951547,-0.328871142664085,
25.7240954537507));
#46666=CARTESIAN_POINT('Ctrl Pts',(9.94932267151757,0.199598255234956,25.7295723838951));
#46667=CARTESIAN_POINT('Ctrl Pts',(9.98107927801918,0.542780303630156,25.9165983405945));
#46668=CARTESIAN_POINT('Ctrl Pts',(10.0128358845208,0.756313557236772,26.2486482930385));
#46669=CARTESIAN_POINT('Ctrl Pts',(10.0445924910224,0.784093796915711,26.6403866625412));
#46670=CARTESIAN_POINT('Ctrl Pts',(10.076349097524,0.621540241153639,26.9988089464404));
#46671=CARTESIAN_POINT('Ctrl Pts',(10.1081057040256,0.307098718342552,27.235068614701));
#46672=CARTESIAN_POINT('Ctrl Pts',(10.1398623105272,-0.0819621986926931,
27.2927198636753));
#46673=CARTESIAN_POINT('Ctrl Pts',(10.1716189170288,-0.451183699623203,
27.1564639171439));
#46674=CARTESIAN_POINT('Ctrl Pts',(10.2033755235304,-0.710341110413239,
26.8613906959017));
#46675=CARTESIAN_POINT('Ctrl Pts',(10.235132130032,-0.796491008458601,26.4761225321646));
#46676=CARTESIAN_POINT('Ctrl Pts',(10.2668887365335,-0.688355039348421,
26.1005432767371));
#46677=CARTESIAN_POINT('Ctrl Pts',(10.3092308785357,-0.320848092753299,
25.720744399325));
#46678=CARTESIAN_POINT('Ctrl Pts',(10.3515730205378,0.24868545684196,25.6948054070466));
#46679=CARTESIAN_POINT('Ctrl Pts',(10.3939151625399,0.649194652036547,26.0396255450656));
#46680=CARTESIAN_POINT('Ctrl Pts',(10.4256717690415,0.791023092992396,26.403820353824));
#46681=CARTESIAN_POINT('Ctrl Pts',(10.4574283755431,0.740250732337037,26.7953245403195));
#46682=CARTESIAN_POINT('Ctrl Pts',(10.4891849820447,0.508988374911209,27.1127335787333));
#46683=CARTESIAN_POINT('Ctrl Pts',(10.5209415885463,0.153681120282412,27.2819876542253));
#46684=CARTESIAN_POINT('Ctrl Pts',(10.5526981950479,-0.239009618237098,
27.2599407330431));
#46685=CARTESIAN_POINT('Ctrl Pts',(10.5844548015495,-0.573625316704213,
27.0532418767055));
#46686=CARTESIAN_POINT('Ctrl Pts',(10.6162114080511,-0.768086580261186,
26.7110796283205));
#46687=CARTESIAN_POINT('Ctrl Pts',(10.6479680145527,-0.776030196845357,
26.3184377118209));
#46688=CARTESIAN_POINT('Ctrl Pts',(10.6797246210543,-0.593564624338813,
25.9683524714423));
#46689=CARTESIAN_POINT('Ctrl Pts',(10.7114812275559,-0.268803421489938,
25.7509051757754));
#46690=CARTESIAN_POINT('Ctrl Pts',(10.753823369558,0.25697906207964,25.6974138359586));
#46691=CARTESIAN_POINT('Ctrl Pts',(10.7961655115601,0.709133976254987,26.0446849521718));
#46692=CARTESIAN_POINT('Ctrl Pts',(10.8385076535623,0.793082515708411,26.5664714853321));
#46693=CARTESIAN_POINT('Ctrl Pts',(10.8702642600639,0.666769034948869,26.9363337162334));
#46694=CARTESIAN_POINT('Ctrl Pts',(10.9020208665655,0.375600348367009,27.2029310842536));
#46695=CARTESIAN_POINT('Ctrl Pts',(10.9337774730671,-0.00580221503551052,
27.2965412346965));
#46696=CARTESIAN_POINT('Ctrl Pts',(10.9655340795687,-0.386547155848502,
27.1969245830134));
#46697=CARTESIAN_POINT('Ctrl Pts',(10.9972906860703,-0.672567178598631,
26.9269530484939));
#46698=CARTESIAN_POINT('Ctrl Pts',(11.0290472925719,-0.795165469044244,
26.5532395993853));
#46699=CARTESIAN_POINT('Ctrl Pts',(11.0608038990735,-0.723293752931155,
26.1662969115487));
#46700=CARTESIAN_POINT('Ctrl Pts',(11.092560505575,-0.476282880095,25.8609832951857));
#46701=CARTESIAN_POINT('Ctrl Pts',(11.1243171120767,-0.111125768016633,
25.7109378214796));
#46702=CARTESIAN_POINT('Ctrl Pts',(11.1560737185782,0.277329037821362,25.7540194775561));
#46703=CARTESIAN_POINT('Ctrl Pts',(11.1984158605804,0.713793524031026,26.0520250072723));
#46704=CARTESIAN_POINT('Ctrl Pts',(11.2407580025825,0.835647851523945,26.6089745718114));
#46705=CARTESIAN_POINT('Ctrl Pts',(11.2831001445846,0.563503958616806,27.0620156792366));
#46706=CARTESIAN_POINT('Ctrl Pts',(11.3148567510862,0.228530189829721,27.2633754058293));
#46707=CARTESIAN_POINT('Ctrl Pts',(11.3466133575878,-0.165922069656989,
27.2795239558244));
#46708=CARTESIAN_POINT('Ctrl Pts',(11.3783699640894,-0.517860513634208,
27.1052537424003));
#46709=CARTESIAN_POINT('Ctrl Pts',(11.410126570591,-0.744748492993213,26.7836763301501));
#46710=CARTESIAN_POINT('Ctrl Pts',(11.4418831770926,-0.789409577719771,
26.3929110932419));
#46711=CARTESIAN_POINT('Ctrl Pts',(11.4736397835942,-0.64225832786655,26.028166535323));
#46712=CARTESIAN_POINT('Ctrl Pts',(11.5053963900958,-0.337898373364977,
25.7786566049734));
#46713=CARTESIAN_POINT('Ctrl Pts',(11.5371529965974,0.0477483654022483,
25.704444958218));
#46714=CARTESIAN_POINT('Ctrl Pts',(11.568909603099,0.423642753883886,25.8250963957939));
#46715=CARTESIAN_POINT('Ctrl Pts',(11.6006662096006,0.692865902039955,26.1084196418678));
#46716=CARTESIAN_POINT('Ctrl Pts',(11.6430083516027,0.834479137823284,26.6175897852527));
#46717=CARTESIAN_POINT('Ctrl Pts',(11.6853504936048,0.568651082127304,27.1219475346471));
#46718=CARTESIAN_POINT('Ctrl Pts',(11.727692635607,0.0685686419494346,27.2929039515766));
#46719=CARTESIAN_POINT('Ctrl Pts',(11.7594492421086,-0.31732463510849,27.2309398975579));
#46720=CARTESIAN_POINT('Ctrl Pts',(11.7912058486102,-0.629310976686018,
26.9890351986573));
#46721=CARTESIAN_POINT('Ctrl Pts',(11.8229624551117,-0.786055773280103,
26.6289493139345));
#46722=CARTESIAN_POINT('Ctrl Pts',(11.8547190616134,-0.752244136277789,
26.2368435113117));
#46723=CARTESIAN_POINT('Ctrl Pts',(11.8864756681149,-0.534515160588541,
25.9092978259331));
#46724=CARTESIAN_POINT('Ctrl Pts',(11.9182322746166,-0.186908610932021,
25.7252821486098));
#46725=CARTESIAN_POINT('Ctrl Pts',(11.9499888811181,0.206614996502733,25.7307004175932));
#46726=CARTESIAN_POINT('Ctrl Pts',(11.9817454876198,0.549294672995457,25.9225373664711));
#46727=CARTESIAN_POINT('Ctrl Pts',(12.0135020941213,0.758915838938966,26.2570703655453));
#46728=CARTESIAN_POINT('Ctrl Pts',(12.0452587006229,0.782128837256907,26.6472169046534));
#46729=CARTESIAN_POINT('Ctrl Pts',(12.0876008426251,0.562204459925782,27.1277809604453));
#46730=CARTESIAN_POINT('Ctrl Pts',(12.1299429846272,0.0338737476163272,
27.3420423732096));
#46731=CARTESIAN_POINT('Ctrl Pts',(12.1722851266293,-0.458655982287092,
27.15040988999));
#46732=CARTESIAN_POINT('Ctrl Pts',(12.2040417331309,-0.713749743328025,
26.8543012302941));
#46733=CARTESIAN_POINT('Ctrl Pts',(12.2357983396325,-0.796354278710274,
26.4682573838007));
#46734=CARTESIAN_POINT('Ctrl Pts',(12.2675549461341,-0.684093539524432,
26.0919220252794));
#46735=CARTESIAN_POINT('Ctrl Pts',(12.2993115526357,-0.405504350759794,
25.8139323651287));
#46736=CARTESIAN_POINT('Ctrl Pts',(12.3310681591373,-0.0279149501101425,
25.7038490903687));
#46737=CARTESIAN_POINT('Ctrl Pts',(12.3628247656389,0.356457281532983,25.7872161726406));
#46738=CARTESIAN_POINT('Ctrl Pts',(12.3945813721405,0.653832357862692,26.0450111516939));
#46739=CARTESIAN_POINT('Ctrl Pts',(12.4263379786421,0.792175442841407,26.4125597423245));
#46740=CARTESIAN_POINT('Ctrl Pts',(12.4580945851437,0.736811757902941,26.8034410837456));
#46741=CARTESIAN_POINT('Ctrl Pts',(12.4898511916453,0.503083492378146,27.1166890097782));
#46742=CARTESIAN_POINT('Ctrl Pts',(12.5321933336474,0.0251849627174119,
27.3423470227353));
#46743=CARTESIAN_POINT('Ctrl Pts',(12.5745354756495,-0.516854899684397,
27.16561535569));
#46744=CARTESIAN_POINT('Ctrl Pts',(12.6168776176517,-0.769897269834191,
26.7016346423272));
#46745=CARTESIAN_POINT('Ctrl Pts',(12.6486342241533,-0.774066619934626,
26.310820387484));
#46746=CARTESIAN_POINT('Ctrl Pts',(12.6803908306549,-0.588390470950266,
25.9624273215664));
#46747=CARTESIAN_POINT('Ctrl Pts',(12.7121474371564,-0.259988325015747,
25.7470606431281));
#46748=CARTESIAN_POINT('Ctrl Pts',(12.7439040436581,0.132189409199892,25.7140938108156));
#46749=CARTESIAN_POINT('Ctrl Pts',(12.7756606501597,0.491830546380316,25.8733116970985));
#46750=CARTESIAN_POINT('Ctrl Pts',(12.8074172566613,0.731965703418775,26.1848035737485));
#46751=CARTESIAN_POINT('Ctrl Pts',(12.8391738631629,0.793156876350488,26.5735783512257));
#46752=CARTESIAN_POINT('Ctrl Pts',(12.8709304696645,0.662016937073565,26.9437581615374));
#46753=CARTESIAN_POINT('Ctrl Pts',(12.902687076166,0.367739430229575,27.2069199172065));
#46754=CARTESIAN_POINT('Ctrl Pts',(12.9344436826677,-0.0128663201484088,
27.2957592556109));
#46755=CARTESIAN_POINT('Ctrl Pts',(12.9767858246698,-0.523694256138937,
27.1602477679971));
#46756=CARTESIAN_POINT('Ctrl Pts',(13.0191279666719,-0.824194056540756,
26.675746824213));
#46757=CARTESIAN_POINT('Ctrl Pts',(13.061470108674,-0.718590181978695,26.1579086592029));
#46758=CARTESIAN_POINT('Ctrl Pts',(13.0932267151756,-0.469871753862732,
25.8564251459149));
#46759=CARTESIAN_POINT('Ctrl Pts',(13.1249833216772,-0.103350723706369,
25.7097428527291));
#46760=CARTESIAN_POINT('Ctrl Pts',(13.1567399281788,0.286546658439126,25.7567620725444));
#46761=CARTESIAN_POINT('Ctrl Pts',(13.1884965346804,0.607634532323689,25.9843423100245));
#46762=CARTESIAN_POINT('Ctrl Pts',(13.220253141182,0.779970642319146,26.3378848789699));
#46763=CARTESIAN_POINT('Ctrl Pts',(13.2520097476836,0.762787909334418,26.7308185076554));
#46764=CARTESIAN_POINT('Ctrl Pts',(13.2837663541852,0.558979957403396,27.0674971466822));
#46765=CARTESIAN_POINT('Ctrl Pts',(13.3155229606868,0.220111430206846,27.265988700436));
#46766=CARTESIAN_POINT('Ctrl Pts',(13.3472795671884,-0.17450318681229,27.2775067174508));
#46767=CARTESIAN_POINT('Ctrl Pts',(13.37903617369,-0.522757319830727,27.1001025909359));
#46768=CARTESIAN_POINT('Ctrl Pts',(13.4213783156921,-0.825963298274264,
26.6672346224978));
#46769=CARTESIAN_POINT('Ctrl Pts',(13.4637204576942,-0.743416216593533,
26.1031182569532));
#46770=CARTESIAN_POINT('Ctrl Pts',(13.5060625996964,-0.328895476366436,
25.7752751551725));
#46771=CARTESIAN_POINT('Ctrl Pts',(13.537819206198,0.0555880103782207,25.7050924387132));
#46772=CARTESIAN_POINT('Ctrl Pts',(13.5695758126996,0.430357382868759,25.8291943247753));
#46773=CARTESIAN_POINT('Ctrl Pts',(13.6013324192012,0.698145424343159,26.1164578631495));
#46774=CARTESIAN_POINT('Ctrl Pts',(13.6330890257028,0.796941593703338,26.497416527793));
#46775=CARTESIAN_POINT('Ctrl Pts',(13.6648456322043,0.700818762673457,26.8787988611799));
#46776=CARTESIAN_POINT('Ctrl Pts',(13.696602238706,0.434409572344521,27.1681398817303));
#46777=CARTESIAN_POINT('Ctrl Pts',(13.7283588452075,0.0615766530934091,
27.2941787708476));
#46778=CARTESIAN_POINT('Ctrl Pts',(13.7601154517091,-0.325445621555236,
27.2275114283046));
#46779=CARTESIAN_POINT('Ctrl Pts',(13.7918720582108,-0.634571402982474,
26.9819618163357));
#46780=CARTESIAN_POINT('Ctrl Pts',(13.8236286647123,-0.786479350664432,
26.6218546924128));
#46781=CARTESIAN_POINT('Ctrl Pts',(13.8659708067145,-0.739282199053725,
26.0954698784758));
#46782=CARTESIAN_POINT('Ctrl Pts',(13.9083129487166,-0.3125600582338,25.7173832361526));
#46783=CARTESIAN_POINT('Ctrl Pts',(13.9506550907188,0.21567771148749,25.7339181115233));
#46784=CARTESIAN_POINT('Ctrl Pts',(13.9824116972203,0.554871109700202,25.9280855750125));
#46785=CARTESIAN_POINT('Ctrl Pts',(14.0141683037219,0.761408101094941,26.2645314575356));
#46786=CARTESIAN_POINT('Ctrl Pts',(14.0459249102235,0.780984108470458,26.6567655146636));
#46787=CARTESIAN_POINT('Ctrl Pts',(14.0776815167251,0.610964975807012,27.0117073152108));
#46788=CARTESIAN_POINT('Ctrl Pts',(14.1094381232267,0.291647913206453,27.241334614104));
#46789=CARTESIAN_POINT('Ctrl Pts',(14.1411947297283,-0.0985343487612529,
27.2908309302356));
#46790=CARTESIAN_POINT('Ctrl Pts',(14.1729513362299,-0.464823397167573,
27.1468777424806));
#46791=CARTESIAN_POINT('Ctrl Pts',(14.2047079427315,-0.717748744514388,
26.8464454800562));
#46792=CARTESIAN_POINT('Ctrl Pts',(14.2364645492331,-0.795816853775414,
26.4594587477287));
#46793=CARTESIAN_POINT('Ctrl Pts',(14.2682211557347,-0.679844423442565,
26.0862248255409));
#46794=CARTESIAN_POINT('Ctrl Pts',(14.3105632977368,-0.304469510421639,
25.714200339602));
#46795=CARTESIAN_POINT('Ctrl Pts',(14.352905439739,0.26548215438068,25.7001862624564));
#46796=CARTESIAN_POINT('Ctrl Pts',(14.3952475817411,0.658687214192637,26.0533127616064));
#46797=CARTESIAN_POINT('Ctrl Pts',(14.4270041882427,0.79286270006155,26.4203960004784));
#46798=CARTESIAN_POINT('Ctrl Pts',(14.4587607947443,0.73390803483815,26.8107518741751));
#46799=CARTESIAN_POINT('Ctrl Pts',(14.4905174012459,0.496053570864849,27.1232515215411));
#46800=CARTESIAN_POINT('Ctrl Pts',(14.5222740077474,0.137281974103891,27.2850326347925));
#46801=CARTESIAN_POINT('Ctrl Pts',(14.5540306142491,-0.254861359535286,
27.2547722853697));
#46802=CARTESIAN_POINT('Ctrl Pts',(14.5857872207506,-0.58507796496343,27.0411158406638));
#46803=CARTESIAN_POINT('Ctrl Pts',(14.6175438272522,-0.772335845023473,
26.6949588335086));
#46804=CARTESIAN_POINT('Ctrl Pts',(14.6493004337538,-0.772060486718305,
26.3022366673227));
#46805=CARTESIAN_POINT('Ctrl Pts',(14.6810570402554,-0.582308270804313,
25.9560467523384));
#46806=CARTESIAN_POINT('Ctrl Pts',(14.712813646757,-0.25306744493287,25.7454437042873));
#46807=CARTESIAN_POINT('Ctrl Pts',(14.7551557887592,0.273719354082281,25.7029676893257));
#46808=CARTESIAN_POINT('Ctrl Pts',(14.7974979307613,0.718507527034393,26.059625474564));
#46809=CARTESIAN_POINT('Ctrl Pts',(14.8398400727634,0.791517698526367,26.5830546085662));
#46810=CARTESIAN_POINT('Ctrl Pts',(14.871596679265,0.657491382035733,26.9501923371599));
#46811=CARTESIAN_POINT('Ctrl Pts',(14.9033532857666,0.360807099282544,27.2106377192428));
#46812=CARTESIAN_POINT('Ctrl Pts',(14.9351098922682,-0.0224710100972664,
27.2962453503641));
#46813=CARTESIAN_POINT('Ctrl Pts',(14.9668664987698,-0.401047778060038,
27.1886822618713));
#46814=CARTESIAN_POINT('Ctrl Pts',(14.9986231052714,-0.681355176354821,
26.912784010108));
#46815=CARTESIAN_POINT('Ctrl Pts',(15.030379711773,-0.796105516889878,26.5365866653381));
#46816=CARTESIAN_POINT('Ctrl Pts',(15.0621363182746,-0.716151580539097,
26.1512328599732));
#46817=CARTESIAN_POINT('Ctrl Pts',(15.0938929247762,-0.462805184149422,
25.8511555714751));
#46818=CARTESIAN_POINT('Ctrl Pts',(15.1256495312778,-0.0945878860313145,
25.7087849914816));
#46819=CARTESIAN_POINT('Ctrl Pts',(15.1574061377794,0.292880226372572,25.7599868189792));
#46820=CARTESIAN_POINT('Ctrl Pts',(15.1997482797815,0.723012441153252,26.067061437389));
#46821=CARTESIAN_POINT('Ctrl Pts',(15.2420904217837,0.833184204547314,26.6264391962602));
#46822=CARTESIAN_POINT('Ctrl Pts',(15.2844325637858,0.551618642248873,27.0736856356996));
#46823=CARTESIAN_POINT('Ctrl Pts',(15.3161891702874,0.21250416882743,27.2679909088782));
#46824=CARTESIAN_POINT('Ctrl Pts',(15.347945776789,-0.182199657223414,27.2758808000015));
#46825=CARTESIAN_POINT('Ctrl Pts',(15.3797023832906,-0.530413882922957,
27.0942833642916));
#46826=CARTESIAN_POINT('Ctrl Pts',(15.4114589897921,-0.750522177579577,
26.7680280564871));
#46827=CARTESIAN_POINT('Ctrl Pts',(15.4432155962938,-0.786995520979564,
26.3764137333501));
#46828=CARTESIAN_POINT('Ctrl Pts',(15.4749722027953,-0.632243102185288,
26.0148286510498));
#46829=CARTESIAN_POINT('Ctrl Pts',(15.5067288092969,-0.32272804759704,25.7717430319143));
#46830=CARTESIAN_POINT('Ctrl Pts',(15.5384854157985,0.0643873344812935,
25.7056184782728));
#46831=CARTESIAN_POINT('Ctrl Pts',(15.5702420223001,0.43767439511808,25.8341102330364));
#46832=CARTESIAN_POINT('Ctrl Pts',(15.6019986288018,0.700909172129369,26.1230057460524));
#46833=CARTESIAN_POINT('Ctrl Pts',(15.6443407708038,0.831835447076346,26.6350280639177));
#46834=CARTESIAN_POINT('Ctrl Pts',(15.686682912806,0.555510380759211,27.1337120844097));
#46835=CARTESIAN_POINT('Ctrl Pts',(15.7290250548081,0.0519596797800127,
27.2941653019125));
#46836=CARTESIAN_POINT('Ctrl Pts',(15.7607816613097,-0.332552292829113,
27.2241388198563));
#46837=CARTESIAN_POINT('Ctrl Pts',(15.7925382678113,-0.639407707442898,
26.9757578318493));
#46838=CARTESIAN_POINT('Ctrl Pts',(15.8242948743129,-0.788582274036148,
26.6124704465499));
#46839=CARTESIAN_POINT('Ctrl Pts',(15.8560514808145,-0.746572027037139,
26.2211581334363));
#46840=CARTESIAN_POINT('Ctrl Pts',(15.8878080873161,-0.522035840432493,
25.8982408316857));
#46841=CARTESIAN_POINT('Ctrl Pts',(15.9195646938177,-0.17065433029262,25.7215401887988));
#46842=CARTESIAN_POINT('Ctrl Pts',(15.9513213003193,0.222669695330672,25.7351929582878));
#46843=CARTESIAN_POINT('Ctrl Pts',(15.9830779068209,0.561259543601463,25.9341595139798));
#46844=CARTESIAN_POINT('Ctrl Pts',(16.0148345133225,0.763833671200898,26.2730062101543));
#46845=CARTESIAN_POINT('Ctrl Pts',(16.0465911198241,0.778876573811572,26.6635531040737));
#46846=CARTESIAN_POINT('Ctrl Pts',(16.0889332618262,0.548943088162816,27.1394093172736));
#46847=CARTESIAN_POINT('Ctrl Pts',(16.1312754038283,0.016244012154183,27.3425668644846));
#46848=CARTESIAN_POINT('Ctrl Pts',(16.1736175458305,-0.47216734905144,27.1406686581801));
#46849=CARTESIAN_POINT('Ctrl Pts',(16.2053741523321,-0.721008259555255,
26.8392862324673));
#46850=CARTESIAN_POINT('Ctrl Pts',(16.2371307588337,-0.795515552951639,
26.4515981827264));
#46851=CARTESIAN_POINT('Ctrl Pts',(16.2688873653352,-0.675403430232317,
26.0776946475575));
#46852=CARTESIAN_POINT('Ctrl Pts',(16.3006439718369,-0.391057471568795,
25.8055962039035));
#46853=CARTESIAN_POINT('Ctrl Pts',(16.3324005783384,-0.0112469392005812,
25.7034392542279));
#46854=CARTESIAN_POINT('Ctrl Pts',(16.3641571848401,0.371296397184491,25.7948322443979));
#46855=CARTESIAN_POINT('Ctrl Pts',(16.3959137913416,0.663211193852015,26.0587942468411));
#46856=CARTESIAN_POINT('Ctrl Pts',(16.4276703978433,0.79383189911164,26.4291575914007));
#46857=CARTESIAN_POINT('Ctrl Pts',(16.4594270043448,0.730299950020167,26.8187946688532));
#46858=CARTESIAN_POINT('Ctrl Pts',(16.4911836108465,0.490067202099917,27.127082508535));
#46859=CARTESIAN_POINT('Ctrl Pts',(16.5335257528485,0.00755075451268908,
27.3426896078416));
#46860=CARTESIAN_POINT('Ctrl Pts',(16.5758678948507,-0.530671740917147,
27.1546528029804));
#46861=CARTESIAN_POINT('Ctrl Pts',(16.6182100368528,-0.773948472755031,
26.6854780218913));
#46862=CARTESIAN_POINT('Ctrl Pts',(16.6499666433544,-0.76993792401264,26.2946621051637));
#46863=CARTESIAN_POINT('Ctrl Pts',(16.681723249856,-0.577011248722235,25.9502311851775));
#46864=CARTESIAN_POINT('Ctrl Pts',(16.7134798563576,-0.244173820480448,
25.7417844965558));
#46865=CARTESIAN_POINT('Ctrl Pts',(16.7452364628592,0.148607952543154,25.7170324051763));
#46866=CARTESIAN_POINT('Ctrl Pts',(16.7769930693608,0.504838200497434,25.8837420128997));
#46867=CARTESIAN_POINT('Ctrl Pts',(16.8087496758624,0.738401842223993,26.2001912317773));
#46868=CARTESIAN_POINT('Ctrl Pts',(16.840506282364,0.791443309939019,26.5901614741675));
#46869=CARTESIAN_POINT('Ctrl Pts',(16.8722628888656,0.652584945679744,26.9575157041844));
#46870=CARTESIAN_POINT('Ctrl Pts',(16.9040194953672,0.352864424260747,27.2144611647807));
#46871=CARTESIAN_POINT('Ctrl Pts',(16.9357761018688,-0.0295172027510032,
27.2953157045016));
#46872=CARTESIAN_POINT('Ctrl Pts',(16.9781182438709,-0.537397266224523,
27.1491432563852));
#46873=CARTESIAN_POINT('Ctrl Pts',(17.0204603858731,-0.82769158569248,26.658459547002));
#46874=CARTESIAN_POINT('Ctrl Pts',(17.0628025278752,-0.711273489859842,
26.1429448814199));
#46875=CARTESIAN_POINT('Ctrl Pts',(17.0945591343768,-0.456300068822577,
25.846732592974));
#46876=CARTESIAN_POINT('Ctrl Pts',(17.1263157408784,-0.0867895361857581,
25.7077530010661));
#46877=CARTESIAN_POINT('Ctrl Pts',(17.1580723473799,0.30203843095996,25.7629217202603));
#46878=CARTESIAN_POINT('Ctrl Pts',(17.1898289538815,0.618293167806677,25.9971718615475));
#46879=CARTESIAN_POINT('Ctrl Pts',(17.2215855603831,0.78319257186756,26.3542436602263));
#46880=CARTESIAN_POINT('Ctrl Pts',(17.2533421668847,0.757790262318726,26.7467316287404));
#46881=CARTESIAN_POINT('Ctrl Pts',(17.2850987733863,0.546980915086662,27.0790712241793));
#46882=CARTESIAN_POINT('Ctrl Pts',(17.316855379888,0.20403256237055,27.2704274425122));
#46883=CARTESIAN_POINT('Ctrl Pts',(17.3486119863895,-0.190736679054125,
27.2736844177905));
#46884=CARTESIAN_POINT('Ctrl Pts',(17.3803685928912,-0.535201811279513,
27.0890308594029));
#46885=CARTESIAN_POINT('Ctrl Pts',(17.4227107348932,-0.829282299959934,
26.6499121849083));
#46886=CARTESIAN_POINT('Ctrl Pts',(17.4650528768954,-0.73494742254484,26.0876469142062));
#46887=CARTESIAN_POINT('Ctrl Pts',(17.5073950188975,-0.313656364480858,
25.7685507409244));
#46888=CARTESIAN_POINT('Ctrl Pts',(17.5391516253991,0.072211731487986,25.7064298750071));
#46889=CARTESIAN_POINT('Ctrl Pts',(17.5709082319007,0.444301753746512,25.8383478091969));
#46890=CARTESIAN_POINT('Ctrl Pts',(17.6026648384023,0.70601938612131,26.1311526579745));
#46891=CARTESIAN_POINT('Ctrl Pts',(17.6344214449039,0.796820980869681,26.5140956120801));
#46892=CARTESIAN_POINT('Ctrl Pts',(17.6661780514055,0.692738004319475,26.8933825384317));
#46893=CARTESIAN_POINT('Ctrl Pts',(17.6979346579071,0.420331066798412,27.1770851633445));
#46894=CARTESIAN_POINT('Ctrl Pts',(17.7296912644087,0.0449434652133512,
27.2952930157502));
#46895=CARTESIAN_POINT('Ctrl Pts',(17.7614478709103,-0.34060148631374,27.2205420816171));
#46896=CARTESIAN_POINT('Ctrl Pts',(17.7932044774119,-0.644515709678365,
26.9685741610806));
#46897=CARTESIAN_POINT('Ctrl Pts',(17.8249610839135,-0.788863074482209,
26.6053716379335));
#46898=CARTESIAN_POINT('Ctrl Pts',(17.8673032259156,-0.730641129956017,
26.08007965548));
#46899=CARTESIAN_POINT('Ctrl Pts',(17.9096453679177,-0.29613832160412,25.711027047467));
#46900=CARTESIAN_POINT('Ctrl Pts',(17.9519875099199,0.231694148623007,25.7385828611072));
#46901=CARTESIAN_POINT('Ctrl Pts',(17.9837441164214,0.566653359359628,25.9398584184328));
#46902=CARTESIAN_POINT('Ctrl Pts',(18.0155007229231,0.766296209055916,26.2804493550768));
#46903=CARTESIAN_POINT('Ctrl Pts',(18.0472573294246,0.777290647856074,26.673205973088));
#46904=CARTESIAN_POINT('Ctrl Pts',(18.0790139359263,0.6005784561905,27.0241353676862));
#46905=CARTESIAN_POINT('Ctrl Pts',(18.1107705424278,0.275214785933559,27.2477375493297));
#46906=CARTESIAN_POINT('Ctrl Pts',(18.1425271489295,-0.113511804048443,
27.2877520601354));
#46907=CARTESIAN_POINT('Ctrl Pts',(18.1848692909315,-0.603105163321842,
27.0885918682123));
#46908=CARTESIAN_POINT('Ctrl Pts',(18.2272114329337,-0.839805528456801,
26.569973072668));
#46909=CARTESIAN_POINT('Ctrl Pts',(18.2695535749358,-0.669488757599245,
26.0696595117695));
#46910=CARTESIAN_POINT('Ctrl Pts',(18.3013101814374,-0.38458849635973,25.8021075061857));
#46911=CARTESIAN_POINT('Ctrl Pts',(18.333066787939,-0.00244655372769168,
25.7030155094137));
#46912=CARTESIAN_POINT('Ctrl Pts',(18.3648233944406,0.378359542695009,25.7990328449791));
#46913=CARTESIAN_POINT('Ctrl Pts',(18.3965800009422,0.668042185748427,26.0654402662492));
#46914=CARTESIAN_POINT('Ctrl Pts',(18.4283366074438,0.794220949673334,26.4379609214166));
#46915=CARTESIAN_POINT('Ctrl Pts',(18.4600932139454,0.7274175711474,26.8255549708114));
#46916=CARTESIAN_POINT('Ctrl Pts',(18.491849820447,0.482615591725175,27.1337143882872));
#46917=CARTESIAN_POINT('Ctrl Pts',(18.5236064269486,0.121339288012704,27.2876956564317));
#46918=CARTESIAN_POINT('Ctrl Pts',(18.5553630334502,-0.271557026497766,
27.2491494235501));
#46919=CARTESIAN_POINT('Ctrl Pts',(18.5871196399518,-0.594542196765398,
27.0290726886231));
#46920=CARTESIAN_POINT('Ctrl Pts',(18.6294617819539,-0.840491465003347,
26.5612933807642));
#46921=CARTESIAN_POINT('Ctrl Pts',(18.671803923956,-0.687172694531139,26.0121716653354));
#46922=CARTESIAN_POINT('Ctrl Pts',(18.7141460659582,-0.234472997417264,
25.7394602274647));
#46923=CARTESIAN_POINT('Ctrl Pts',(18.7459026724598,0.155802722384311,25.7185311453641));
#46924=CARTESIAN_POINT('Ctrl Pts',(18.7776592789614,0.511839522475942,25.8890924505991));
#46925=CARTESIAN_POINT('Ctrl Pts',(18.8094158854629,0.741094448594219,26.2079544172491));
#46926=CARTESIAN_POINT('Ctrl Pts',(18.8411724919646,0.790852991429545,26.5983571259894));
#46927=CARTESIAN_POINT('Ctrl Pts',(18.8729290984662,0.647208072939979,26.964496744374));
#46928=CARTESIAN_POINT('Ctrl Pts',(18.9046857049677,0.346303229108121,27.2177720053648));
#46929=CARTESIAN_POINT('Ctrl Pts',(18.9364423114694,-0.0394890010879801,
27.2955829454142));
#46930=CARTESIAN_POINT('Ctrl Pts',(18.9681989179709,-0.414953219279804,
27.1804421773526));
#46931=CARTESIAN_POINT('Ctrl Pts',(18.9999555244725,-0.690495493529877,
26.8977235614153));
#46932=CARTESIAN_POINT('Ctrl Pts',(19.0317121309741,-0.795578750754377,
26.5212787788603));
#46933=CARTESIAN_POINT('Ctrl Pts',(19.0740542729763,-0.682103411352699,
26.0051083701625));
#46934=CARTESIAN_POINT('Ctrl Pts',(19.1163964149784,-0.210938010442085,
25.6841029814942));
#46935=CARTESIAN_POINT('Ctrl Pts',(19.1587385569805,0.310953319631399,25.7673975374766));
#46936=CARTESIAN_POINT('Ctrl Pts',(19.1904951634821,0.622827872514436,26.002955234302));
#46937=CARTESIAN_POINT('Ctrl Pts',(19.2222517699837,0.78509669838758,26.3628471470069));
#46938=CARTESIAN_POINT('Ctrl Pts',(19.2540083764853,0.754844992184846,26.7544025197296));
#46939=CARTESIAN_POINT('Ctrl Pts',(19.2857649829869,0.54124693951236,27.0849566894835));
#46940=CARTESIAN_POINT('Ctrl Pts',(19.3175215894885,0.195421936564938,27.2722990237309));
#46941=CARTESIAN_POINT('Ctrl Pts',(19.3492781959901,-0.197887083474027,
27.2719865803867));
#46942=CARTESIAN_POINT('Ctrl Pts',(19.3810348024917,-0.542997981900108,
27.0828076834802));
#46943=CARTESIAN_POINT('Ctrl Pts',(19.4127914089933,-0.755842259642186,
26.7527651270297));
#46944=CARTESIAN_POINT('Ctrl Pts',(19.4445480154949,-0.784276255245929,
26.3590077543049));
#46945=CARTESIAN_POINT('Ctrl Pts',(19.4763046219965,-0.621973401147041,
26.0034645799642));
#46946=CARTESIAN_POINT('Ctrl Pts',(19.5186467639986,-0.202509532859472,
25.6819702461652));
#46947=CARTESIAN_POINT('Ctrl Pts',(19.5609889060007,0.364628407821791,25.7402441752329));
#46948=CARTESIAN_POINT('Ctrl Pts',(19.6033310480029,0.709950204635276,26.1403209180076));
#46949=CARTESIAN_POINT('Ctrl Pts',(19.6350876545045,0.796560342324164,26.5214401241865));
#46950=CARTESIAN_POINT('Ctrl Pts',(19.6668442610061,0.688648014289257,26.9011877905904));
#46951=CARTESIAN_POINT('Ctrl Pts',(19.6986008675076,0.413135351067633,27.1810512359355));
#46952=CARTESIAN_POINT('Ctrl Pts',(19.7303574740093,0.0367650668537481,
27.2960972980499));
#46953=CARTESIAN_POINT('Ctrl Pts',(19.7621140805108,-0.348389341911593,
27.2164219300026));
#46954=CARTESIAN_POINT('Ctrl Pts',(19.7938706870124,-0.64889140428939,26.962668913525));
#46955=CARTESIAN_POINT('Ctrl Pts',(19.8256272935141,-0.790806567494741,
26.5955854438622));
#46956=CARTESIAN_POINT('Ctrl Pts',(19.8573839000156,-0.74080149737149,26.2060597468949));
#46957=CARTESIAN_POINT('Ctrl Pts',(19.8891405065173,-0.508737507276705,
25.8866858826192));
#46958=CARTESIAN_POINT('Ctrl Pts',(19.9208971130188,-0.155477746603945,
25.7194713295494));
#46959=CARTESIAN_POINT('Ctrl Pts',(19.963239255021,0.372447071308012,25.7440463187918));
#46960=CARTESIAN_POINT('Ctrl Pts',(20.0055813970231,0.768489532327075,26.154158088483));
#46961=CARTESIAN_POINT('Ctrl Pts',(20.0479235390252,0.774628079308121,26.6826189306506));
#46962=CARTESIAN_POINT('Ctrl Pts',(20.0796801455268,0.595188665990073,27.0298287551329));
#46963=CARTESIAN_POINT('Ctrl Pts',(20.1114367520284,0.267911625081069,27.2506071489466));
#46964=CARTESIAN_POINT('Ctrl Pts',(20.14319335853,-0.12312173971539,27.2869896069711));
#46965=CARTESIAN_POINT('Ctrl Pts',(20.1749499650316,-0.485029654910406,
27.132351810277));
#46966=CARTESIAN_POINT('Ctrl Pts',(20.2067065715332,-0.728142381884628,
26.8231782589373));
#46967=CARTESIAN_POINT('Ctrl Pts',(20.2384631780348,-0.794329601343219,
26.4354782011024));
#46968=CARTESIAN_POINT('Ctrl Pts',(20.2702197845364,-0.666220487545662,
26.0633515530251));
#46969=CARTESIAN_POINT('Ctrl Pts',(20.301976391038,-0.376913700709203,25.7977722640617));
#46970=CARTESIAN_POINT('Ctrl Pts',(20.3337329975396,0.00636821150313297,
25.7031766169527));
#46971=CARTESIAN_POINT('Ctrl Pts',(20.3654896040411,0.384233136322356,25.8030328328849));
#46972=CARTESIAN_POINT('Ctrl Pts',(20.4078317460434,0.77201653498693,26.1621046630022));
#46973=CARTESIAN_POINT('Ctrl Pts',(20.4501738880454,0.81046519188054,26.7309306428521));
#46974=CARTESIAN_POINT('Ctrl Pts',(20.4925160300476,0.474529817347993,27.1389207991076));
#46975=CARTESIAN_POINT('Ctrl Pts',(20.5242726365491,0.113539747006181,27.2887184438939));
#46976=CARTESIAN_POINT('Ctrl Pts',(20.5560292430508,-0.278985653677384,
27.2465619438101));
#46977=CARTESIAN_POINT('Ctrl Pts',(20.5877858495523,-0.601400203401613,
27.0223307377703));
#46978=CARTESIAN_POINT('Ctrl Pts',(20.619542456054,-0.778421549050925,26.670828774146));
#46979=CARTESIAN_POINT('Ctrl Pts',(20.6512990625556,-0.76500962662566,26.2777483711726));
#46980=CARTESIAN_POINT('Ctrl Pts',(20.6830556690571,-0.565714119049419,
25.9386711181391));
#46981=CARTESIAN_POINT('Ctrl Pts',(20.7148122755588,-0.227907934100152,
25.7367375432753));
#46982=CARTESIAN_POINT('Ctrl Pts',(20.7465688820603,0.164464593988673,25.7201672434249));
#46983=CARTESIAN_POINT('Ctrl Pts',(20.778325488562,0.518475108459405,25.8948953645883));
#46984=CARTESIAN_POINT('Ctrl Pts',(20.8100820950635,0.743006763321614,26.2147995709279));
#46985=CARTESIAN_POINT('Ctrl Pts',(20.8524242370657,0.808039650977486,26.739279567674));
#46986=CARTESIAN_POINT('Ctrl Pts',(20.8947663790678,0.470788843887705,27.1989568323787));
#46987=CARTESIAN_POINT('Ctrl Pts',(20.9371085210699,-0.0490268475710841,
27.2943517503612));
#46988=CARTESIAN_POINT('Ctrl Pts',(20.9688651275715,-0.421575592023053,
27.1761967746885));
#46989=CARTESIAN_POINT('Ctrl Pts',(21.0006217340731,-0.694507228865489,
26.8909570819885));
#46990=CARTESIAN_POINT('Ctrl Pts',(21.0323783405747,-0.796476381207539,
26.5117037792914));
#46991=CARTESIAN_POINT('Ctrl Pts',(21.0641349470763,-0.705250943174314,
26.1288616359701));
#46992=CARTESIAN_POINT('Ctrl Pts',(21.0958915535779,-0.441630110964222,
25.8369778582611));
#46993=CARTESIAN_POINT('Ctrl Pts',(21.1276481600795,-0.0707011018639236,
25.70619654051));
#46994=CARTESIAN_POINT('Ctrl Pts',(21.1594047665811,0.317727575909635,25.7695475431092));
#46995=CARTESIAN_POINT('Ctrl Pts',(21.1911613730827,0.628395710084807,26.009789267304));
#46996=CARTESIAN_POINT('Ctrl Pts',(21.2229179795843,0.786429550765298,26.3715608331863));
#46997=CARTESIAN_POINT('Ctrl Pts',(21.2546745860859,0.751894885449026,26.7608685805538));
#46998=CARTESIAN_POINT('Ctrl Pts',(21.297016728088,0.463552958450529,27.2037765581276));
#46999=CARTESIAN_POINT('Ctrl Pts',(21.3393588700901,-0.0905842644351466,
27.3378408441313));
#47000=CARTESIAN_POINT('Ctrl Pts',(21.3817010120923,-0.549496531103895,
27.0757185921867));
#47001=CARTESIAN_POINT('Ctrl Pts',(21.4134576185938,-0.758168930798584,
26.7452507497653));
#47002=CARTESIAN_POINT('Ctrl Pts',(21.4452142250955,-0.782981966253044,
26.3512486254657));
#47003=CARTESIAN_POINT('Ctrl Pts',(21.476970831597,-0.616487950568337,25.9955654541219));
#47004=CARTESIAN_POINT('Ctrl Pts',(21.5087274380987,-0.299974232084392,
25.7616653616493));
#47005=CARTESIAN_POINT('Ctrl Pts',(21.5404840446002,0.0897151756284967,
25.7084277022228));
#47006=CARTESIAN_POINT('Ctrl Pts',(21.5722406511019,0.457605408654088,25.8475278794664));
#47007=CARTESIAN_POINT('Ctrl Pts',(21.6039972576034,0.713743622414307,26.1463311637505));
#47008=CARTESIAN_POINT('Ctrl Pts',(21.6357538641051,0.796412224677964,26.5302539135788));
#47009=CARTESIAN_POINT('Ctrl Pts',(21.6675104706066,0.684050486030751,26.9087089312087));
#47010=CARTESIAN_POINT('Ctrl Pts',(21.6992670771083,0.406712042690736,27.184093304612));
#47011=CARTESIAN_POINT('Ctrl Pts',(21.7416092191103,-0.0992230806999048,
27.3368617384697));
#47012=CARTESIAN_POINT('Ctrl Pts',(21.7839513611125,-0.609300801297396,
27.0821815203151));
#47013=CARTESIAN_POINT('Ctrl Pts',(21.8262935031146,-0.791205620922703,
26.5859767439771));
#47014=CARTESIAN_POINT('Ctrl Pts',(21.8580501096162,-0.737736826165347,
26.1988149518847));
#47015=CARTESIAN_POINT('Ctrl Pts',(21.8898067161178,-0.502746680944055,
25.8815879159468));
#47016=CARTESIAN_POINT('Ctrl Pts',(21.9215633226194,-0.146192340398604,
25.7169678142758));
#47017=CARTESIAN_POINT('Ctrl Pts',(21.953319929121,0.246561806406779,25.7421544657884));
#47018=CARTESIAN_POINT('Ctrl Pts',(21.9850765356226,0.578813148913968,25.9526327978489));
#47019=CARTESIAN_POINT('Ctrl Pts',(22.0168331421242,0.770423302724975,26.2961115189095));
#47020=CARTESIAN_POINT('Ctrl Pts',(22.0485897486258,0.773654319674137,26.6896591625013));
#47021=CARTESIAN_POINT('Ctrl Pts',(22.0803463551274,0.589394342448357,27.0364718445485));
#47022=CARTESIAN_POINT('Ctrl Pts',(22.112102961629,0.259548714643134,27.253394002243));
#47023=CARTESIAN_POINT('Ctrl Pts',(22.1438595681306,-0.129993482523563,
27.2851751585385));
#47024=CARTESIAN_POINT('Ctrl Pts',(22.1862017101327,-0.615274487721257,
27.0758646488693));
#47025=CARTESIAN_POINT('Ctrl Pts',(22.2285438521349,-0.841094622237496,
26.5523700821198));
#47026=CARTESIAN_POINT('Ctrl Pts',(22.2708859941369,-0.660332128994326,
26.055748028139));
#47027=CARTESIAN_POINT('Ctrl Pts',(22.3026426006386,-0.369900855742956,
25.7942086605736));
#47028=CARTESIAN_POINT('Ctrl Pts',(22.3343992071401,0.01423446586742,25.7031404697911));
#47029=CARTESIAN_POINT('Ctrl Pts',(22.3661558136418,0.392945955132557,25.8071038457199));
#47030=CARTESIAN_POINT('Ctrl Pts',(22.3979124201434,0.676990688980436,26.0795167243078));
#47031=CARTESIAN_POINT('Ctrl Pts',(22.4296690266449,0.79534519032439,26.4545957758109));
#47032=CARTESIAN_POINT('Ctrl Pts',(22.4614256331466,0.720445109942096,26.8407072374687));
#47033=CARTESIAN_POINT('Ctrl Pts',(22.4931822396481,0.469247428456909,27.1436757375867));
#47034=CARTESIAN_POINT('Ctrl Pts',(22.5249388461498,0.104827792755421,27.290062570161));
#47035=CARTESIAN_POINT('Ctrl Pts',(22.5566954526513,-0.287175811024369,
27.2433021669895));
#47036=CARTESIAN_POINT('Ctrl Pts',(22.5884520591529,-0.605484443472687,
27.0165142048358));
#47037=CARTESIAN_POINT('Ctrl Pts',(22.630794201155,-0.841590140778907,26.5436900904305));
#47038=CARTESIAN_POINT('Ctrl Pts',(22.6731363431572,-0.676812887645703,
25.9978973171006));
#47039=CARTESIAN_POINT('Ctrl Pts',(22.7154784851593,-0.218505020300182,
25.7347197303026));
#47040=CARTESIAN_POINT('Ctrl Pts',(22.7472350916609,0.172123229852927,25.7219629497037));
#47041=CARTESIAN_POINT('Ctrl Pts',(22.7789916981625,0.524512533349801,25.899938058812));
#47042=CARTESIAN_POINT('Ctrl Pts',(22.8107483046641,0.747044085909005,26.2235280520929));
#47043=CARTESIAN_POINT('Ctrl Pts',(22.8425049111657,0.788621357728243,26.6148866059988));
#47044=CARTESIAN_POINT('Ctrl Pts',(22.8742615176673,0.637345306587861,26.9779398241586));
#47045=CARTESIAN_POINT('Ctrl Pts',(22.9060181241689,0.331205804787041,27.2248622579349));
#47046=CARTESIAN_POINT('Ctrl Pts',(22.9377747306705,-0.0561303630539786,
27.2945822717721));
#47047=CARTESIAN_POINT('Ctrl Pts',(22.9695313371721,-0.429102675280415,
27.1716089821991));
#47048=CARTESIAN_POINT('Ctrl Pts',(23.0012879436737,-0.698667848123337,
26.8831857198376));
#47049=CARTESIAN_POINT('Ctrl Pts',(23.0330445501753,-0.795849829993106,
26.5046241955528));
#47050=CARTESIAN_POINT('Ctrl Pts',(23.0753866921774,-0.671596896209279,
25.9909416555441));
#47051=CARTESIAN_POINT('Ctrl Pts',(23.1177288341795,-0.193816666742857,
25.679867151767));
#47052=CARTESIAN_POINT('Ctrl Pts',(23.1600709761817,0.326217167037633,25.7740656400097));
#47053=CARTESIAN_POINT('Ctrl Pts',(23.1918275826833,0.633093647904743,26.0160986765141));
#47054=CARTESIAN_POINT('Ctrl Pts',(23.2235841891849,0.787795093385811,26.3793077395167));
#47055=CARTESIAN_POINT('Ctrl Pts',(23.2553407956864,0.749355516936845,26.7701442457419));
#47056=CARTESIAN_POINT('Ctrl Pts',(23.2870974021881,0.528886386857991,27.0961558251828));
#47057=CARTESIAN_POINT('Ctrl Pts',(23.3188540086896,0.179216412751493,27.2762196807263));
#47058=CARTESIAN_POINT('Ctrl Pts',(23.3506106151912,-0.213999927519153,
27.2676761095181));
#47059=CARTESIAN_POINT('Ctrl Pts',(23.3823672216928,-0.55507609312846,27.071316142874));
#47060=CARTESIAN_POINT('Ctrl Pts',(23.4141238281944,-0.760966602883749,
26.7368914523551));
#47061=CARTESIAN_POINT('Ctrl Pts',(23.445880434696,-0.781153791542167,26.3426252502845));
#47062=CARTESIAN_POINT('Ctrl Pts',(23.4776370411976,-0.611445654087914,
25.9905566300544));
#47063=CARTESIAN_POINT('Ctrl Pts',(23.5199791831997,-0.185345401108989,
25.6779112752593));
#47064=CARTESIAN_POINT('Ctrl Pts',(23.5623213252019,0.380448766828713,25.7480415404581));
#47065=CARTESIAN_POINT('Ctrl Pts',(23.604663467204,0.717322101045798,26.1552575766811));
#47066=CARTESIAN_POINT('Ctrl Pts',(23.6364200737056,0.795937182645239,26.538105894183));
#47067=CARTESIAN_POINT('Ctrl Pts',(23.6681766802072,0.680101105708285,26.915511993711));
#47068=CARTESIAN_POINT('Ctrl Pts',(23.6999332867088,0.398791784083484,27.1895481978939));
#47069=CARTESIAN_POINT('Ctrl Pts',(23.7316898932104,0.0200962396143968,
27.296692361741));
#47070=CARTESIAN_POINT('Ctrl Pts',(23.763446499712,-0.363306363014758,27.2089739077987));
#47071=CARTESIAN_POINT('Ctrl Pts',(23.7952031062136,-0.658432051321634,
26.9489875409133));
#47072=CARTESIAN_POINT('Ctrl Pts',(23.8269597127152,-0.792633786547248,
26.5790144587714));
#47073=CARTESIAN_POINT('Ctrl Pts',(23.8587163192167,-0.734487649662804,
26.1906205834317));
#47074=CARTESIAN_POINT('Ctrl Pts',(23.8904729257184,-0.495790608642908,
25.8761733171223));
#47075=CARTESIAN_POINT('Ctrl Pts',(23.9222295322199,-0.139108740631515,
25.7163884295363));
#47076=CARTESIAN_POINT('Ctrl Pts',(23.9645716742221,0.388186146399965,25.752006480776));
#47077=CARTESIAN_POINT('Ctrl Pts',(24.0069138162242,0.775559022505738,26.170316831385));
#47078=CARTESIAN_POINT('Ctrl Pts',(24.0492559582264,0.770636562786746,26.6987904001223));
#47079=CARTESIAN_POINT('Ctrl Pts',(24.0810125647279,0.583970020170633,27.0421688606243));
#47080=CARTESIAN_POINT('Ctrl Pts',(24.1127691712296,0.252144193813407,27.2560496256394));
#47081=CARTESIAN_POINT('Ctrl Pts',(24.1445257777311,-0.139564942859222,
27.2842405440908));
#47082=CARTESIAN_POINT('Ctrl Pts',(24.1762823842328,-0.498157324775064,
27.1220625835686));
#47083=CARTESIAN_POINT('Ctrl Pts',(24.2080389907343,-0.734746402362433,
26.8078688674774));
#47084=CARTESIAN_POINT('Ctrl Pts',(24.2397955972359,-0.79280531419185,26.418868551768));
#47085=CARTESIAN_POINT('Ctrl Pts',(24.2715522037375,-0.656936368068052,
26.0495044810648));
#47086=CARTESIAN_POINT('Ctrl Pts',(24.3033088102391,-0.362134883698147,
25.7900379891063));
#47087=CARTESIAN_POINT('Ctrl Pts',(24.3350654167407,0.0230427874213672,
25.7034844082904));
#47088=CARTESIAN_POINT('Ctrl Pts',(24.3668220232423,0.398735156543778,25.8112267354052));
#47089=CARTESIAN_POINT('Ctrl Pts',(24.4091641652445,0.778918946276761,26.178335478815));
#47090=CARTESIAN_POINT('Ctrl Pts',(24.4515063072465,0.805454755862356,26.7478415326711));
#47091=CARTESIAN_POINT('Ctrl Pts',(24.4938484492488,0.461054512471806,27.1487118556139));
#47092=CARTESIAN_POINT('Ctrl Pts',(24.5256050557503,0.0970085300212661,
27.2909218690818));
#47093=CARTESIAN_POINT('Ctrl Pts',(24.5573616622519,-0.294548647426862,
27.2405598052841));
#47094=CARTESIAN_POINT('Ctrl Pts',(24.5891182687535,-0.612199858231308,
27.0096301971554));
#47095=CARTESIAN_POINT('Ctrl Pts',(24.6208748752551,-0.781826177841934,
26.6545005040255));
#47096=CARTESIAN_POINT('Ctrl Pts',(24.6526314817566,-0.760190781059477,
26.2617868774846));
#47097=CARTESIAN_POINT('Ctrl Pts',(24.6843880882583,-0.553842691960536,
25.9269547568778));
#47098=CARTESIAN_POINT('Ctrl Pts',(24.7161446947598,-0.211884413187848,
25.7321350380964));
#47099=CARTESIAN_POINT('Ctrl Pts',(24.7479013012615,0.180748963367304,25.7237799647362));
#47100=CARTESIAN_POINT('Ctrl Pts',(24.7796579077631,0.531025222621527,25.90587857232));
#47101=CARTESIAN_POINT('Ctrl Pts',(24.8114145142647,0.74881272581408,26.2304117273629));
#47102=CARTESIAN_POINT('Ctrl Pts',(24.8537566562668,0.802855019359397,26.7561378670706));
#47103=CARTESIAN_POINT('Ctrl Pts',(24.8960987982689,0.456057920405105,27.2086564487069));
#47104=CARTESIAN_POINT('Ctrl Pts',(24.9384409402711,-0.0656403540824771,
27.2931517376899));
#47105=CARTESIAN_POINT('Ctrl Pts',(24.9701975467727,-0.435634749553036,
27.1672259159165));
#47106=CARTESIAN_POINT('Ctrl Pts',(25.0019541532743,-0.702537095515253,
26.8763367645186));
#47107=CARTESIAN_POINT('Ctrl Pts',(25.0337107597758,-0.796546877646502,
26.4950325073963));
#47108=CARTESIAN_POINT('Ctrl Pts',(25.0654673662775,-0.697329274606203,
26.1141833843906));
#47109=CARTESIAN_POINT('Ctrl Pts',(25.097223972779,-0.427657617209193,25.827880607489));
#47110=CARTESIAN_POINT('Ctrl Pts',(25.1289805792807,-0.0540728476927859,
25.7048907589234));
#47111=CARTESIAN_POINT('Ctrl Pts',(25.1607371857822,0.33294494419036,25.7763569468244));
#47112=CARTESIAN_POINT('Ctrl Pts',(25.1924937922838,0.638517242951082,26.0230477368148));
#47113=CARTESIAN_POINT('Ctrl Pts',(25.2242503987854,0.788945293266577,26.3880474112795));
#47114=CARTESIAN_POINT('Ctrl Pts',(25.256007005287,0.746270734187485,26.7765471503739));
#47115=CARTESIAN_POINT('Ctrl Pts',(25.2983491472892,0.44872275221358,27.2133236857863));
#47116=CARTESIAN_POINT('Ctrl Pts',(25.3406912892913,-0.108098811743075,
27.335761590382));
#47117=CARTESIAN_POINT('Ctrl Pts',(25.3830334312934,-0.561424858091366,
27.0640926021514));
#47118=CARTESIAN_POINT('Ctrl Pts',(25.4147900377951,-0.763135503094323,
26.7293300281363));
#47119=CARTESIAN_POINT('Ctrl Pts',(25.4465466442966,-0.779697402476066,
26.3348949077807));
#47120=CARTESIAN_POINT('Ctrl Pts',(25.4783032507982,-0.605796091498349,
25.9827740341064));
#47121=CARTESIAN_POINT('Ctrl Pts',(25.5100598572998,-0.284456618484401,
25.7555491887942));
#47122=CARTESIAN_POINT('Ctrl Pts',(25.5418164638014,0.106261602193242,25.710478634078));
#47123=CARTESIAN_POINT('Ctrl Pts',(25.5735730703029,0.471160163992154,25.857247576466));
#47124=CARTESIAN_POINT('Ctrl Pts',(25.6053296768046,0.720988905220201,26.1613458949732));
#47125=CARTESIAN_POINT('Ctrl Pts',(25.6370862833062,0.795604641852137,26.5469146534013));
#47126=CARTESIAN_POINT('Ctrl Pts',(25.6688428898078,0.675347181544284,26.9229352697116));
#47127=CARTESIAN_POINT('Ctrl Pts',(25.7005994963094,0.392306217773594,27.1924551729066));
#47128=CARTESIAN_POINT('Ctrl Pts',(25.7429416383115,-0.116715244884512,
27.3346019054481));
#47129=CARTESIAN_POINT('Ctrl Pts',(25.7852837803136,-0.621351287349472,
27.0693025272348));
#47130=CARTESIAN_POINT('Ctrl Pts',(25.8276259223158,-0.792831660382392,
26.5693995118972));
#47131=CARTESIAN_POINT('Ctrl Pts',(25.8593825288174,-0.731272031625445,
26.1834415128479));
#47132=CARTESIAN_POINT('Ctrl Pts',(25.8911391353189,-0.489694400926831,
25.8712018432531));
#47133=CARTESIAN_POINT('Ctrl Pts',(25.9228957418205,-0.129772979866902,
25.714079788392));
#47134=CARTESIAN_POINT('Ctrl Pts',(25.9546523483221,0.262368055635802,25.7474805067894));
#47135=CARTESIAN_POINT('Ctrl Pts',(25.9864089548237,0.590141695668152,25.9648661194057));
#47136=CARTESIAN_POINT('Ctrl Pts',(26.0181655613253,0.774521596165084,26.3122796401661));
#47137=CARTESIAN_POINT('Ctrl Pts',(26.0499221678269,0.769515607711255,26.7058087142711));
#47138=CARTESIAN_POINT('Ctrl Pts',(26.0816787743285,0.5780380710276,27.0486892252408));
#47139=CARTESIAN_POINT('Ctrl Pts',(26.1134353808301,0.243724544676253,27.2586608600213));
#47140=CARTESIAN_POINT('Ctrl Pts',(26.1451919873318,-0.146396766368369,
27.282282661157));
#47141=CARTESIAN_POINT('Ctrl Pts',(26.1875341293338,-0.627192464881676,
27.062862066019));
#47142=CARTESIAN_POINT('Ctrl Pts',(26.2298762713361,-0.842004480180732,
26.534756044308));
#47143=CARTESIAN_POINT('Ctrl Pts',(26.2722184133381,-0.650892539114633,
26.0420259586536));
#47144=CARTESIAN_POINT('Ctrl Pts',(26.3039750198397,-0.355044020423166,
25.7866217100636));
#47145=CARTESIAN_POINT('Ctrl Pts',(26.3357316263413,0.0308983993041465,
25.7036133259667));
#47146=CARTESIAN_POINT('Ctrl Pts',(26.3674882328429,0.407379290301616,25.8154783693755));
#47147=CARTESIAN_POINT('Ctrl Pts',(26.3992448393445,0.685607456858645,26.0937785591144));
#47148=CARTESIAN_POINT('Ctrl Pts',(26.4310014458461,0.796187063432195,26.4712471071119));
#47149=CARTESIAN_POINT('Ctrl Pts',(26.4627580523477,0.713032807660742,26.855721513956));
#47150=CARTESIAN_POINT('Ctrl Pts',(26.4839291233488,0.541616553385129,27.0541076712552));
#47151=CARTESIAN_POINT('Ctrl Pts',(26.4945146588493,0.437388125541368,27.1268353453143));
#47152=CARTESIAN_POINT('',(26.4075,0.887101818743898,26.8183655338816));
#47153=CARTESIAN_POINT('Ctrl Pts',(26.4428553390594,0.547713856063084,27.2849429494197));
#47154=CARTESIAN_POINT('Ctrl Pts',(26.4403015215003,0.582091546070041,27.2596651488676));
#47155=CARTESIAN_POINT('Ctrl Pts',(26.4377478434971,0.614688075782228,27.2320922094722));
#47156=CARTESIAN_POINT('Ctrl Pts',(26.4351883782295,0.645331373578053,27.2024576259984));
#47157=CARTESIAN_POINT('Ctrl Pts',(26.4334556727824,0.666076257160053,27.1823956213061));
#47158=CARTESIAN_POINT('Ctrl Pts',(26.4317203150251,0.68592535478861,27.1613878091695));
#47159=CARTESIAN_POINT('Ctrl Pts',(26.4299804660993,0.704814988397489,27.1394978057222));
#47160=CARTESIAN_POINT('Ctrl Pts',(26.429150320803,0.713827920644061,27.1290532877378));
#47161=CARTESIAN_POINT('Ctrl Pts',(26.4283191530511,0.722622287140125,27.1184078428865));
#47162=CARTESIAN_POINT('Ctrl Pts',(26.4274867630985,0.731190377254997,27.1075679654722));
#47163=CARTESIAN_POINT('Ctrl Pts',(26.4269700334783,0.736509261675482,27.1008388047929));
#47164=CARTESIAN_POINT('Ctrl Pts',(26.4264526784239,0.741742465290211,27.0940326563995));
#47165=CARTESIAN_POINT('Ctrl Pts',(26.4259351560647,0.746883024781805,27.0871577648099));
#47166=CARTESIAN_POINT('Ctrl Pts',(26.4233544388515,0.772517338217262,27.0528748961589));
#47167=CARTESIAN_POINT('Ctrl Pts',(26.4207778202209,0.795770458426538,27.0169961987609));
#47168=CARTESIAN_POINT('Ctrl Pts',(26.4181993932428,0.81646839864648,26.9797548648337));
#47169=CARTESIAN_POINT('Ctrl Pts',(26.4168907728525,0.826973154778107,26.9608538956183));
#47170=CARTESIAN_POINT('Ctrl Pts',(26.4155816866621,0.836819115669743,26.941601383311));
#47171=CARTESIAN_POINT('Ctrl Pts',(26.4142713624564,0.845979193354906,26.9220250507742));
#47172=CARTESIAN_POINT('Ctrl Pts',(26.4120192059813,0.861723333759698,26.8883776802318));
#47173=CARTESIAN_POINT('Ctrl Pts',(26.4097633921638,0.875442884267091,26.8537738979748));
#47174=CARTESIAN_POINT('Ctrl Pts',(26.4074999999956,0.887094662747573,26.8184069534176));
#47175=CARTESIAN_POINT('Ctrl Pts',(26.4075,0.702460755335681,26.1986212829383));
#47176=CARTESIAN_POINT('Ctrl Pts',(26.4075,0.724104732401363,26.224024074543));
#47177=CARTESIAN_POINT('Ctrl Pts',(26.4075,0.743985347108709,26.2508566613889));
#47178=CARTESIAN_POINT('Ctrl Pts',(26.4075,0.762051830778776,26.2788529213646));
#47179=CARTESIAN_POINT('Ctrl Pts',(26.4075,0.781091487998052,26.3083572346052));
#47180=CARTESIAN_POINT('Ctrl Pts',(26.4075,0.79811757528923,26.3391539940486));
#47181=CARTESIAN_POINT('Ctrl Pts',(26.4075,0.813068246637555,26.3709924441191));
#47182=CARTESIAN_POINT('Ctrl Pts',(26.4075,0.818689978394547,26.3829642961975));
#47183=CARTESIAN_POINT('Ctrl Pts',(26.4075,0.824018141973892,26.3950840167916));
#47184=CARTESIAN_POINT('Ctrl Pts',(26.4075,0.829048786022781,26.4073402559923));
#47185=CARTESIAN_POINT('Ctrl Pts',(26.4075,0.832452526428086,26.415632843617));
#47186=CARTESIAN_POINT('Ctrl Pts',(26.4075,0.835716738922779,26.4239799751948));
#47187=CARTESIAN_POINT('Ctrl Pts',(26.4075,0.838839667726155,26.4323745124417));
#47188=CARTESIAN_POINT('Ctrl Pts',(26.4075,0.843376079903281,26.4445685403514));
#47189=CARTESIAN_POINT('Ctrl Pts',(26.4075,0.847615144743271,26.4568644216205));
#47190=CARTESIAN_POINT('Ctrl Pts',(26.4075,0.851554819573637,26.4692493635078));
#47191=CARTESIAN_POINT('Ctrl Pts',(26.4075,0.862536111498967,26.5037706547816));
#47192=CARTESIAN_POINT('Ctrl Pts',(26.4075,0.871193227879546,26.5389805248123));
#47193=CARTESIAN_POINT('Ctrl Pts',(26.4075,0.87759612970566,26.5746307452721));
#47194=CARTESIAN_POINT('Ctrl Pts',(26.4075,0.881461513193471,26.5961525141895));
#47195=CARTESIAN_POINT('Ctrl Pts',(26.4075,0.884504926078275,26.6178357226439));
#47196=CARTESIAN_POINT('Ctrl Pts',(26.4075,0.886736695632634,26.6396330336608));
#47197=CARTESIAN_POINT('Ctrl Pts',(26.4075,0.887583223161862,26.6479009230596));
#47198=CARTESIAN_POINT('Ctrl Pts',(26.4075,0.888312931455761,26.6561852775869));
#47199=CARTESIAN_POINT('Ctrl Pts',(26.4075,0.888926212894426,26.6644836796199));
#47200=CARTESIAN_POINT('Ctrl Pts',(26.4075,0.889537315014905,26.6727525929756));
#47201=CARTESIAN_POINT('Ctrl Pts',(26.4075,0.890032032238849,26.6810245992922));
#47202=CARTESIAN_POINT('Ctrl Pts',(26.4075,0.890411592374961,26.6892991424034));
#47203=CARTESIAN_POINT('Ctrl Pts',(26.4075,0.892188989170611,26.72804701135));
#47204=CARTESIAN_POINT('Ctrl Pts',(26.4075,0.891442494227263,26.766834586409));
#47205=CARTESIAN_POINT('Ctrl Pts',(26.4075,0.888261545772562,26.8053932068493));
#47206=CARTESIAN_POINT('Ctrl Pts',(26.4075,0.887903437733349,26.8097340983027));
#47207=CARTESIAN_POINT('Ctrl Pts',(26.4075,0.887514442749773,26.8140721311828));
#47208=CARTESIAN_POINT('Ctrl Pts',(26.4075,0.887094662732194,26.8184069534123));
#47209=CARTESIAN_POINT('',(9.6,0.66215021624593,26.1181780341239));
#47210=CARTESIAN_POINT('Ctrl Pts',(9.60000000000002,0.662150216245817,26.1181780341239));
#47211=CARTESIAN_POINT('Ctrl Pts',(9.61058553550055,0.725638504704611,26.2282785199239));
#47212=CARTESIAN_POINT('Ctrl Pts',(9.63175660650163,0.796605391005151,26.480675629033));
#47213=CARTESIAN_POINT('Ctrl Pts',(9.6635132130032,0.708650864432033,26.8640803773426));
#47214=CARTESIAN_POINT('Ctrl Pts',(9.69526981950482,0.448266436304386,27.1588859127484));
#47215=CARTESIAN_POINT('Ctrl Pts',(9.7270264260064,0.0782001173243299,27.2927247256205));
#47216=CARTESIAN_POINT('Ctrl Pts',(9.75878303250801,-0.310157515624281,
27.2341585395261));
#47217=CARTESIAN_POINT('Ctrl Pts',(9.7905396390096,-0.624341483803593,26.9951389225185));
#47218=CARTESIAN_POINT('Ctrl Pts',(9.81537842347006,-0.749031686158336,
26.716022731786));
#47219=CARTESIAN_POINT('Ctrl Pts',(9.82963167242999,-0.764213466994258,
26.5441969818453));
#47220=CARTESIAN_POINT('Ctrl Pts',(9.83329938588939,-0.764354837691052,
26.4999637734947));
#47221=CARTESIAN_POINT('Ctrl Pts',(9.6,0.899181451069003,26.9202569089796));
#47222=CARTESIAN_POINT('Ctrl Pts',(9.6,0.907250892683643,26.8807649655044));
#47223=CARTESIAN_POINT('Ctrl Pts',(9.6,0.912814425070195,26.8408626129725));
#47224=CARTESIAN_POINT('Ctrl Pts',(9.6,0.915826552715021,26.8007896179812));
#47225=CARTESIAN_POINT('Ctrl Pts',(9.6,0.918777836392666,26.7615260840352));
#47226=CARTESIAN_POINT('Ctrl Pts',(9.6,0.919279144120976,26.722097769122));
#47227=CARTESIAN_POINT('Ctrl Pts',(9.6,0.917249439708845,26.6827606307352));
#47228=CARTESIAN_POINT('Ctrl Pts',(9.6,0.91650588615301,26.6683500254524));
#47229=CARTESIAN_POINT('Ctrl Pts',(9.6,0.915422334890081,26.6539520254147));
#47230=CARTESIAN_POINT('Ctrl Pts',(9.6,0.913993735787157,26.6395806368628));
#47231=CARTESIAN_POINT('Ctrl Pts',(9.6,0.912867742205004,26.6282533924016));
#47232=CARTESIAN_POINT('Ctrl Pts',(9.6,0.911526840337707,26.6169401702507));
#47233=CARTESIAN_POINT('Ctrl Pts',(9.6,0.909972044783114,26.6056708003737));
#47234=CARTESIAN_POINT('Ctrl Pts',(9.6,0.90487132111677,26.5687000607378));
#47235=CARTESIAN_POINT('Ctrl Pts',(9.6,0.897466999839062,26.5321448048616));
#47236=CARTESIAN_POINT('Ctrl Pts',(9.6,0.887699646549959,26.4962326846631));
#47237=CARTESIAN_POINT('Ctrl Pts',(9.6,0.886096693095341,26.4903390248936));
#47238=CARTESIAN_POINT('Ctrl Pts',(9.6,0.884430025516682,26.48446277673));
#47239=CARTESIAN_POINT('Ctrl Pts',(9.6,0.882699302581969,26.4786050578291));
#47240=CARTESIAN_POINT('Ctrl Pts',(9.6,0.872596303121075,26.4444109475464));
#47241=CARTESIAN_POINT('Ctrl Pts',(9.6,0.860311415881943,26.4108446276722));
#47242=CARTESIAN_POINT('Ctrl Pts',(9.6,0.845888980484608,26.378149615024));
#47243=CARTESIAN_POINT('Ctrl Pts',(9.6,0.840991978648279,26.3670483320183));
#47244=CARTESIAN_POINT('Ctrl Pts',(9.6,0.835845528233583,26.3560424349843));
#47245=CARTESIAN_POINT('Ctrl Pts',(9.6,0.83046648420776,26.3451721019));
#47246=CARTESIAN_POINT('Ctrl Pts',(9.6,0.815111322539747,26.3141413609181));
#47247=CARTESIAN_POINT('Ctrl Pts',(9.6,0.797847456292624,26.2841727552048));
#47248=CARTESIAN_POINT('Ctrl Pts',(9.6,0.77873876852075,26.2554703858443));
#47249=CARTESIAN_POINT('Ctrl Pts',(9.6,0.76024206322928,26.2276872500494));
#47250=CARTESIAN_POINT('Ctrl Pts',(9.6,0.740015758053793,26.2010902999295));
#47251=CARTESIAN_POINT('Ctrl Pts',(9.6,0.718109952543232,26.1759118525573));
#47252=CARTESIAN_POINT('Ctrl Pts',(9.6,0.700529207372861,26.1557046126626));
#47253=CARTESIAN_POINT('Ctrl Pts',(9.6,0.681866325015503,26.1364118903963));
#47254=CARTESIAN_POINT('Ctrl Pts',(9.6,0.662150216245888,26.1181780341239));
#47255=CARTESIAN_POINT('Ctrl Pts',(26.3575,0.966230510866419,26.2733743026085));
#47256=CARTESIAN_POINT('Ctrl Pts',(26.3510374103638,0.943190455260765,26.175271874718));
#47257=CARTESIAN_POINT('Ctrl Pts',(26.3445748207275,0.905342771426808,26.0806300603281));
#47258=CARTESIAN_POINT('Ctrl Pts',(26.3381122310913,0.85397204810411,25.9939874654059));
#47259=CARTESIAN_POINT('Ctrl Pts',(26.3275266955908,0.769828284376302,25.8520693929252));
#47260=CARTESIAN_POINT('Ctrl Pts',(26.3169411600902,0.6494028879358,25.731612822717));
#47261=CARTESIAN_POINT('Ctrl Pts',(26.3063556245897,0.507714145949595,25.6471752845257));
#47262=CARTESIAN_POINT('Ctrl Pts',(26.2957700890892,0.366025403963423,25.5627377463344));
#47263=CARTESIAN_POINT('Ctrl Pts',(26.2851845535887,0.203073316431535,25.51431924016));
#47264=CARTESIAN_POINT('Ctrl Pts',(26.2745990180881,0.038073613875047,25.5080742314669));
#47265=CARTESIAN_POINT('Ctrl Pts',(26.2640134825876,-0.12692608868146,25.5018292227739));
#47266=CARTESIAN_POINT('Ctrl Pts',(26.253427947087,-0.293973406262545,25.5377577115622));
#47267=CARTESIAN_POINT('Ctrl Pts',(26.2428424115865,-0.441523068585815,
25.610995220108));
#47268=CARTESIAN_POINT('Ctrl Pts',(26.232256876086,-0.589072730909101,25.6842327286538));
#47269=CARTESIAN_POINT('Ctrl Pts',(26.2216713405855,-0.717124737974537,
25.794779256957));
#47270=CARTESIAN_POINT('Ctrl Pts',(26.2110858050849,-0.812170333563929,
25.9300280902216));
#47271=CARTESIAN_POINT('Ctrl Pts',(26.2005002695844,-0.907215929153311,
26.0652769234861));
#47272=CARTESIAN_POINT('Ctrl Pts',(26.1899147340839,-0.969255113266671,
26.2252280617121));
#47273=CARTESIAN_POINT('Ctrl Pts',(26.1793291985833,-0.987370317670422,
26.3890071383319));
#47274=CARTESIAN_POINT('Ctrl Pts',(26.1769417249343,-0.991456041359965,
26.4259460565071));
#47275=CARTESIAN_POINT('Ctrl Pts',(26.1745542512852,-0.993307404832562,
26.4630796973216));
#47276=CARTESIAN_POINT('Ctrl Pts',(26.1721667776362,-0.993011273520018,
26.5001944908134));
#47277=CARTESIAN_POINT('Origin',(26.4251776695297,0.,26.5));
#47278=CARTESIAN_POINT('',(26.4075,-0.93691208277389,26.6024792620495));
#47279=CARTESIAN_POINT('Ctrl Pts',(26.4075000000007,-0.936837214195958,
26.6024576131701));
#47280=CARTESIAN_POINT('Ctrl Pts',(26.410745248043,-0.942820328546626,26.5601312037567));
#47281=CARTESIAN_POINT('Ctrl Pts',(26.4139775393434,-0.945947559415033,
26.5174819531867));
#47282=CARTESIAN_POINT('Ctrl Pts',(26.4172042771818,-0.946194674320254,
26.4748112889781));
#47283=CARTESIAN_POINT('Ctrl Pts',(26.4199365043253,-0.946403917861382,
26.4386800775753));
#47284=CARTESIAN_POINT('Ctrl Pts',(26.4226647497551,-0.94454742016796,26.4025327690601));
#47285=CARTESIAN_POINT('Ctrl Pts',(26.4253935079933,-0.940581316298395,
26.3665500875366));
#47286=CARTESIAN_POINT('Ctrl Pts',(26.4265821111055,-0.93885374537013,26.3508766113581));
#47287=CARTESIAN_POINT('Ctrl Pts',(26.4277708115146,-0.936725552147973,
26.3352343970121));
#47288=CARTESIAN_POINT('Ctrl Pts',(26.4289599806693,-0.934201239741837,
26.319637053445));
#47289=CARTESIAN_POINT('Ctrl Pts',(26.4296389953106,-0.93275985936615,26.3107309826767));
#47290=CARTESIAN_POINT('Ctrl Pts',(26.4303182652535,-0.931188922788708,
26.3018382283537));
#47291=CARTESIAN_POINT('Ctrl Pts',(26.4309964994545,-0.929492931583898,
26.2929790744995));
#47292=CARTESIAN_POINT('Ctrl Pts',(26.434148130317,-0.921611969201675,26.2518121993028));
#47293=CARTESIAN_POINT('Ctrl Pts',(26.4372840391634,-0.911022048127747,
26.2112836035419));
#47294=CARTESIAN_POINT('Ctrl Pts',(26.4404115024132,-0.897868176129323,
26.1716298451886));
#47295=CARTESIAN_POINT('Ctrl Pts',(26.4412266454206,-0.89443974678467,26.1612944771099));
#47296=CARTESIAN_POINT('Ctrl Pts',(26.4420412146901,-0.890836862988219,
26.1510185492494));
#47297=CARTESIAN_POINT('Ctrl Pts',(26.4428553390593,-0.887061520921181,
26.1408063078486));
#47298=CARTESIAN_POINT('Origin',(26.4075,0.,26.5));
#47299=CARTESIAN_POINT('Origin',(26.4075,9.00781732476477E-17,26.5));
#47300=CARTESIAN_POINT('Ctrl Pts',(26.4075,-0.936837214193549,26.6024576131701));
#47301=CARTESIAN_POINT('Ctrl Pts',(26.4075,-0.933888297224056,26.5812044318456));
#47302=CARTESIAN_POINT('Ctrl Pts',(26.4075,-0.930200091360513,26.5600464692594));
#47303=CARTESIAN_POINT('Ctrl Pts',(26.4075,-0.925762213721532,26.5390303476949));
#47304=CARTESIAN_POINT('Ctrl Pts',(26.4075,-0.923851791507024,26.5299833056703));
#47305=CARTESIAN_POINT('Ctrl Pts',(26.4075,-0.921801990307457,26.5209608466283));
#47306=CARTESIAN_POINT('Ctrl Pts',(26.4075,-0.91961313840563,26.5119721671209));
#47307=CARTESIAN_POINT('Ctrl Pts',(26.4075,-0.910761827123966,26.4756236136786));
#47308=CARTESIAN_POINT('Ctrl Pts',(26.4075,-0.899666778401924,26.4399338213958));
#47309=CARTESIAN_POINT('Ctrl Pts',(26.4075,-0.886299889617234,26.4051323253511));
#47310=CARTESIAN_POINT('Ctrl Pts',(26.4075,-0.882533408506134,26.3953260660486));
#47311=CARTESIAN_POINT('Ctrl Pts',(26.4075,-0.878586371075686,26.3855905978107));
#47312=CARTESIAN_POINT('Ctrl Pts',(26.4075,-0.874457770423122,26.3759317127677));
#47313=CARTESIAN_POINT('Ctrl Pts',(26.4075,-0.860409573041769,26.3430658739551));
#47314=CARTESIAN_POINT('Ctrl Pts',(26.4075,-0.844259571750178,26.3110832093572));
#47315=CARTESIAN_POINT('Ctrl Pts',(26.4075,-0.826080250833576,26.280221179434));
#47316=CARTESIAN_POINT('Ctrl Pts',(26.4075,-0.819767876265086,26.2695050094674));
#47317=CARTESIAN_POINT('Ctrl Pts',(26.4075,-0.813206985360593,26.2589189247773));
#47318=CARTESIAN_POINT('Ctrl Pts',(26.4075,-0.806420124795332,26.2485029477329));
#47319=CARTESIAN_POINT('Ctrl Pts',(26.4075,-0.787519580466189,26.2194957751282));
#47320=CARTESIAN_POINT('Ctrl Pts',(26.4075,-0.766849244348869,26.1917685090718));
#47321=CARTESIAN_POINT('Ctrl Pts',(26.4075,-0.744495822943584,26.1655159597568));
#47322=CARTESIAN_POINT('Ctrl Pts',(26.4075,-0.722855094261229,26.1401004188136));
#47323=CARTESIAN_POINT('Ctrl Pts',(26.4075,-0.699635820512491,26.116066939103));
#47324=CARTESIAN_POINT('Ctrl Pts',(26.4075,-0.674914432867557,26.0936401042275));
#47325=CARTESIAN_POINT('Ctrl Pts',(26.4075,-0.655118740238286,26.0756817785778));
#47326=CARTESIAN_POINT('Ctrl Pts',(26.4075,-0.634359630469717,26.0587545344762));
#47327=CARTESIAN_POINT('Ctrl Pts',(26.4075,-0.612682133358436,26.0429972363723));
#47328=CARTESIAN_POINT('Ctrl Pts',(9.53886739174678,-0.692454762064432,
26.8236314647775));
#47329=CARTESIAN_POINT('Ctrl Pts',(9.54947659464505,-0.746387612144165,
26.7082345923037));
#47330=CARTESIAN_POINT('Ctrl Pts',(9.57069500044159,-0.795395645701817,
26.4500764782137));
#47331=CARTESIAN_POINT('Ctrl Pts',(9.60252260913642,-0.67404341179918,26.0748447559888));
#47332=CARTESIAN_POINT('Ctrl Pts',(9.63435021783122,-0.387770113791111,
25.8037814721796));
#47333=CARTESIAN_POINT('Ctrl Pts',(9.66617782652605,-0.00653957363242062,
25.7030919772491));
#47334=CARTESIAN_POINT('Ctrl Pts',(9.69800543522088,0.376272204290504,25.7974986628543));
#47335=CARTESIAN_POINT('Ctrl Pts',(9.72983304391567,0.66698890097209,26.0638527475773));
#47336=CARTESIAN_POINT('Ctrl Pts',(9.76166065261051,0.794431941545588,26.4369759237776));
#47337=CARTESIAN_POINT('Ctrl Pts',(9.79348826130532,0.727413669545738,26.8255225525671));
#47338=CARTESIAN_POINT('Ctrl Pts',(9.82531587000014,0.482334658244354,27.1343885069846));
#47339=CARTESIAN_POINT('Ctrl Pts',(9.85714347869494,0.119188665110999,27.2879652485877));
#47340=CARTESIAN_POINT('Ctrl Pts',(9.88897108738978,-0.273133232602854,
27.2486612961868));
#47341=CARTESIAN_POINT('Ctrl Pts',(9.92079869608458,-0.598596265249733,
27.0260967569105));
#47342=CARTESIAN_POINT('Ctrl Pts',(9.95262630477941,-0.77753264721618,26.6747523236194));
#47343=CARTESIAN_POINT('Ctrl Pts',(9.98445391347422,-0.766141435875682,
26.2806312379679));
#47344=CARTESIAN_POINT('Ctrl Pts',(10.016281522169,-0.567211114828819,25.9402081539091));
#47345=CARTESIAN_POINT('Ctrl Pts',(10.0481091308639,-0.229436586427856,
25.7368131175217));
#47346=CARTESIAN_POINT('Ctrl Pts',(10.0799367395587,0.164500331356799,25.7202340098908));
#47347=CARTESIAN_POINT('Ctrl Pts',(10.1117643482535,0.518170209717155,25.8945291116224));
#47348=CARTESIAN_POINT('Ctrl Pts',(10.1435919569483,0.745000323495275,26.2170337856481));
#47349=CARTESIAN_POINT('Ctrl Pts',(10.1754195656431,0.789466300620247,26.608804051599));
#47350=CARTESIAN_POINT('Ctrl Pts',(10.207247174338,0.640683580453765,26.9739408306562));
#47351=CARTESIAN_POINT('Ctrl Pts',(10.2390747830327,0.335071789291362,27.2230644903377));
#47352=CARTESIAN_POINT('Ctrl Pts',(10.2709023917276,-0.0525602054491083,
27.2951935525961));
#47353=CARTESIAN_POINT('Ctrl Pts',(10.3027300004224,-0.427326304238472,
27.1726719786772));
#47354=CARTESIAN_POINT('Ctrl Pts',(10.3345576091172,-0.697489773146787,
26.8854910862812));
#47355=CARTESIAN_POINT('Ctrl Pts',(10.366385217812,-0.796918925171605,26.5039481547106));
#47356=CARTESIAN_POINT('Ctrl Pts',(10.3982128265068,-0.701275097630571,
26.121438778171));
#47357=CARTESIAN_POINT('Ctrl Pts',(10.4300404352017,-0.433970366467297,
25.8315951210098));
#47358=CARTESIAN_POINT('Ctrl Pts',(10.4618680438965,-0.0604366454286784,
25.7053662648007));
#47359=CARTESIAN_POINT('Ctrl Pts',(10.4936956525913,0.327890997713297,25.7736510102933));
#47360=CARTESIAN_POINT('Ctrl Pts',(10.5255232612861,0.635956180167181,26.0197343462881));
#47361=CARTESIAN_POINT('Ctrl Pts',(10.5573508699809,0.78834948304845,26.3833790164421));
#47362=CARTESIAN_POINT('Ctrl Pts',(10.5891784786757,0.747767468424727,26.775570634129));
#47363=CARTESIAN_POINT('Ctrl Pts',(10.6210060873706,0.524143963013505,27.1003069775249));
#47364=CARTESIAN_POINT('Ctrl Pts',(10.6528336960654,0.172218416622154,27.2780977947564));
#47365=CARTESIAN_POINT('Ctrl Pts',(10.6846613047602,-0.221863437780272,
27.2654227434594));
#47366=CARTESIAN_POINT('Ctrl Pts',(10.716488913455,-0.561636678720128,27.0653844730313));
#47367=CARTESIAN_POINT('Ctrl Pts',(10.7483165221498,-0.763930262821534,
26.7269491457883));
#47368=CARTESIAN_POINT('Ctrl Pts',(10.7801441308446,-0.779225963129924,
26.3329603052779));
#47369=CARTESIAN_POINT('Ctrl Pts',(10.8119717395395,-0.603779637374724,
25.9798601046639));
#47370=CARTESIAN_POINT('Ctrl Pts',(10.8437993482343,-0.280537733984753,
25.7540818134411));
#47371=CARTESIAN_POINT('Ctrl Pts',(10.8756269569291,0.111375310126204,25.7108923384462));
#47372=CARTESIAN_POINT('Ctrl Pts',(10.9074545656239,0.476025463481309,25.8608637709017));
#47373=CARTESIAN_POINT('Ctrl Pts',(10.9392821743187,0.724152213281463,26.1672855079379));
#47374=CARTESIAN_POINT('Ctrl Pts',(10.9711097830136,0.795018108239294,26.5551504197647));
#47375=CARTESIAN_POINT('Ctrl Pts',(11.0029373917084,0.671276313132874,26.9295153928038));
#47376=CARTESIAN_POINT('Ctrl Pts',(11.0347650004032,0.383216836026789,27.1987418821097));
#47377=CARTESIAN_POINT('Ctrl Pts',(11.066592609098,0.00135201979696231,
27.2969275583584));
#47378=CARTESIAN_POINT('Ctrl Pts',(11.0984202177928,-0.380843749208507,
27.2000381417591));
#47379=CARTESIAN_POINT('Ctrl Pts',(11.1302478264876,-0.669815072706669,
26.9317906085171));
#47380=CARTESIAN_POINT('Ctrl Pts',(11.1620754351825,-0.794826402440226,
26.5578476552035));
#47381=CARTESIAN_POINT('Ctrl Pts',(11.1939030438773,-0.725276968616409,
26.1697445230988));
#47382=CARTESIAN_POINT('Ctrl Pts',(11.2257306525721,-0.478191357872257,
25.8624826382875));
#47383=CARTESIAN_POINT('Ctrl Pts',(11.2575582612669,-0.114052167341973,
25.7112747852685));
#47384=CARTESIAN_POINT('Ctrl Pts',(11.2893858699617,0.278005165684963,25.7531342228479));
#47385=CARTESIAN_POINT('Ctrl Pts',(11.3212134786565,0.6020112901178,25.977814431644));
#47386=CARTESIAN_POINT('Ctrl Pts',(11.3530410873514,0.778654699980662,26.3303172977978));
#47387=CARTESIAN_POINT('Ctrl Pts',(11.3848686960462,0.764695919842463,26.7243557697161));
#47388=CARTESIAN_POINT('Ctrl Pts',(11.416696304741,0.563551835344745,27.0634755452618));
#47389=CARTESIAN_POINT('Ctrl Pts',(11.4485239134358,0.224459294363696,27.2646655389139));
#47390=CARTESIAN_POINT('Ctrl Pts',(11.4803515221306,-0.169577284164262,
27.2786776649706));
#47391=CARTESIAN_POINT('Ctrl Pts',(11.5121791308255,-0.522104061573776,
27.1020819795649));
#47392=CARTESIAN_POINT('Ctrl Pts',(11.5440067395203,-0.746828133179442,
26.7781062759456));
#47393=CARTESIAN_POINT('Ctrl Pts',(11.5758343482151,-0.788740648209462,
26.386054613561));
#47394=CARTESIAN_POINT('Ctrl Pts',(11.6076619569099,-0.637582094773173,
26.0218949554196));
#47395=CARTESIAN_POINT('Ctrl Pts',(11.6394895656047,-0.330353663928771,
25.7747677489538));
#47396=CARTESIAN_POINT('Ctrl Pts',(11.6713171742995,0.0577400488194873,
25.7051657732641));
#47397=CARTESIAN_POINT('Ctrl Pts',(11.7031447829944,0.431699923094752,25.8301264763938));
#47398=CARTESIAN_POINT('Ctrl Pts',(11.7349723916892,0.69998657563618,26.1190614811315));
#47399=CARTESIAN_POINT('Ctrl Pts',(11.766800000384,0.796927734095428,26.5012441294702));
#47400=CARTESIAN_POINT('Ctrl Pts',(11.7986276090788,0.698793756689006,26.883122234856));
#47401=CARTESIAN_POINT('Ctrl Pts',(11.8304552177736,0.42960626815974,27.1712181579684));
#47402=CARTESIAN_POINT('Ctrl Pts',(11.8622828264684,0.055258051066885,27.2950106345332));
#47403=CARTESIAN_POINT('Ctrl Pts',(11.8941104351633,-0.332616451231466,
27.2241972504773));
#47404=CARTESIAN_POINT('Ctrl Pts',(11.9259380438581,-0.639071777563019,
26.9761119871953));
#47405=CARTESIAN_POINT('Ctrl Pts',(11.9577656525529,-0.789092576016674,
26.6114821407401));
#47406=CARTESIAN_POINT('Ctrl Pts',(11.9895932612477,-0.745956159717636,
26.219563253107));
#47407=CARTESIAN_POINT('Ctrl Pts',(12.0214208699425,-0.520221631970104,
25.8962907861735));
#47408=CARTESIAN_POINT('Ctrl Pts',(12.0532484786374,-0.167145187013454,
25.720796658319));
#47409=CARTESIAN_POINT('Ctrl Pts',(12.0850760873322,0.226845720661642,25.7360390191599));
#47410=CARTESIAN_POINT('Ctrl Pts',(12.116903696027,0.565308431882582,25.9382867830725));
#47411=CARTESIAN_POINT('Ctrl Pts',(12.1487313047218,0.76539269994308,26.2780329391498));
#47412=CARTESIAN_POINT('Ctrl Pts',(12.1805589134166,0.778121103043664,26.6721130739564));
#47413=CARTESIAN_POINT('Ctrl Pts',(12.2123865221114,0.600377932120684,27.0240626869479));
#47414=CARTESIAN_POINT('Ctrl Pts',(12.2442141308062,0.275671866485382,27.2477301540376));
#47415=CARTESIAN_POINT('Ctrl Pts',(12.2760417395011,-0.116514253498911,
27.2883652643034));
#47416=CARTESIAN_POINT('Ctrl Pts',(12.3078693481959,-0.480179551758527,
27.1360211940663));
#47417=CARTESIAN_POINT('Ctrl Pts',(12.3396969568907,-0.726304592236129,
26.8279893298955));
#47418=CARTESIAN_POINT('Ctrl Pts',(12.3715245655855,-0.794641910002403,
26.4396709348958));
#47419=CARTESIAN_POINT('Ctrl Pts',(12.4033521742804,-0.668463625002977,
26.0661201280579));
#47420=CARTESIAN_POINT('Ctrl Pts',(12.4351797829751,-0.378656158975322,
25.7987761594907));
#47421=CARTESIAN_POINT('Ctrl Pts',(12.46700739167,0.00384026553403038,25.7030805476152));
#47422=CARTESIAN_POINT('Ctrl Pts',(12.4988350003648,0.385396654593795,25.8024580443755));
#47423=CARTESIAN_POINT('Ctrl Pts',(12.5306626090596,0.672614119883514,26.0725826314222));
#47424=CARTESIAN_POINT('Ctrl Pts',(12.5624902177544,0.79518642952386,26.4473321394994));
#47425=CARTESIAN_POINT('Ctrl Pts',(12.5943178264493,0.723109846747402,26.8349738956479));
#47426=CARTESIAN_POINT('Ctrl Pts',(12.626145435144,0.474027563748743,27.1406194112225));
#47427=CARTESIAN_POINT('Ctrl Pts',(12.6579730438389,0.108910931026614,27.2894515630053));
#47428=CARTESIAN_POINT('Ctrl Pts',(12.6898006525337,-0.282865351947728,
27.2450386257746));
#47429=CARTESIAN_POINT('Ctrl Pts',(12.7216282612285,-0.605400730631636,
27.0182521746981));
#47430=CARTESIAN_POINT('Ctrl Pts',(12.7534558699233,-0.779743714034942,
26.6646058979855));
#47431=CARTESIAN_POINT('Ctrl Pts',(12.7852834786181,-0.763217934251803,
26.2706667358078));
#47432=CARTESIAN_POINT('Ctrl Pts',(12.817111087313,-0.559868637292059,25.9328646808695));
#47433=CARTESIAN_POINT('Ctrl Pts',(12.8489386960078,-0.219472471696671,
25.7338882618077));
#47434=CARTESIAN_POINT('Ctrl Pts',(12.8807663047026,0.174647037187299,25.7224437167444));
#47435=CARTESIAN_POINT('Ctrl Pts',(12.9125939133974,0.526015750672588,25.9013324868735));
#47436=CARTESIAN_POINT('Ctrl Pts',(12.9444215220922,0.748624239560586,26.2267654685606));
#47437=CARTESIAN_POINT('Ctrl Pts',(12.976249130787,0.787981513819465,26.6190818840437));
#47438=CARTESIAN_POINT('Ctrl Pts',(13.0080767394819,0.634453543543031,26.9822489629997));
#47439=CARTESIAN_POINT('Ctrl Pts',(13.0399043481767,0.325621515054088,27.2273692254711));
#47440=CARTESIAN_POINT('Ctrl Pts',(13.0717319568715,-0.0629174411427496,
27.2944411600796));
#47441=CARTESIAN_POINT('Ctrl Pts',(13.1035595655663,-0.436055216210945,
27.1670466322858));
#47442=CARTESIAN_POINT('Ctrl Pts',(13.1353871742611,-0.702453663598643,
26.8763697805689));
#47443=CARTESIAN_POINT('Ctrl Pts',(13.167214782956,-0.796902713314313,26.4935636391573));
#47444=CARTESIAN_POINT('Ctrl Pts',(13.1990423916508,-0.696282751850487,
26.1123330157156));
#47445=CARTESIAN_POINT('Ctrl Pts',(13.2308700003456,-0.425223933001015,
25.8259970563627));
#47446=CARTESIAN_POINT('Ctrl Pts',(13.2626976090404,-0.0500771109931841,
25.7046462144535));
#47447=CARTESIAN_POINT('Ctrl Pts',(13.2945252177352,0.337327785132049,25.777985231033));
#47448=CARTESIAN_POINT('Ctrl Pts',(13.32635282643,0.64216024626656,26.0280618903463));
#47449=CARTESIAN_POINT('Ctrl Pts',(13.3581804351249,0.789802171887619,26.3936614345112));
#47450=CARTESIAN_POINT('Ctrl Pts',(13.3900080438197,0.744113185060425,26.7852909550754));
#47451=CARTESIAN_POINT('Ctrl Pts',(13.4218356525145,0.516277217440969,27.107085822582));
#47452=CARTESIAN_POINT('Ctrl Pts',(13.4536632612093,0.162064862066652,27.2802758113077));
#47453=CARTESIAN_POINT('Ctrl Pts',(13.4854908699041,-0.231818373908386,
27.2624667879633));
#47454=CARTESIAN_POINT('Ctrl Pts',(13.5173184785989,-0.568956187617919,
27.058018116014));
#47455=CARTESIAN_POINT('Ctrl Pts',(13.5491460872938,-0.766822646030525,
26.7169755533772));
#47456=CARTESIAN_POINT('Ctrl Pts',(13.5809736959886,-0.776983211600699,
26.3228208530349));
#47457=CARTESIAN_POINT('Ctrl Pts',(13.6128013046834,-0.59695074073402,25.9720367679793));
#47458=CARTESIAN_POINT('Ctrl Pts',(13.6446289133782,-0.270794296674234,
25.7504896197401));
#47459=CARTESIAN_POINT('Ctrl Pts',(13.676456522073,0.121648250824199,25.7124105991698));
#47460=CARTESIAN_POINT('Ctrl Pts',(13.7082841307678,0.484313256342262,25.86712084016));
#47461=CARTESIAN_POINT('Ctrl Pts',(13.7401117394627,0.728426139452693,26.176749755467));
#47462=CARTESIAN_POINT('Ctrl Pts',(13.7719393481575,0.794231979098091,26.5655051494659));
#47463=CARTESIAN_POINT('Ctrl Pts',(13.8037669568523,0.665622560492644,26.9382259328153));
#47464=CARTESIAN_POINT('Ctrl Pts',(13.8355945655471,0.374079407913512,27.2036760318525));
#47465=CARTESIAN_POINT('Ctrl Pts',(13.8674221742419,-0.00903238784518047,
27.2968775170617));
#47466=CARTESIAN_POINT('Ctrl Pts',(13.8992497829368,-0.389933199833693,
27.1950161587302));
#47467=CARTESIAN_POINT('Ctrl Pts',(13.9310773916315,-0.675384614490799,
26.9230259847075));
#47468=CARTESIAN_POINT('Ctrl Pts',(13.9629050003264,-0.795512700825137,
26.5474858300392));
#47469=CARTESIAN_POINT('Ctrl Pts',(13.9947326090212,-0.720912028757716,
26.160321905297));
#47470=CARTESIAN_POINT('Ctrl Pts',(14.026560217716,-0.469843647084554,25.856305733657));
#47471=CARTESIAN_POINT('Ctrl Pts',(14.0583878264108,-0.10376507142601,25.7098556010573));
#47472=CARTESIAN_POINT('Ctrl Pts',(14.0902154351057,0.287713530534183,25.7568201526036));
#47473=CARTESIAN_POINT('Ctrl Pts',(14.1220430438004,0.608764471794302,25.9857032188419));
#47474=CARTESIAN_POINT('Ctrl Pts',(14.1538706524953,0.780799627852441,26.3404778937761));
#47475=CARTESIAN_POINT('Ctrl Pts',(14.1856982611901,0.761707549946172,26.734301023437));
#47476=CARTESIAN_POINT('Ctrl Pts',(14.2175258698849,0.556161672732346,27.0707710180205));
#47477=CARTESIAN_POINT('Ctrl Pts',(14.2493534785797,0.214476332390549,27.2675254159133));
#47478=CARTESIAN_POINT('Ctrl Pts',(14.2811810872745,-0.17970937641759,27.2764018941606));
#47479=CARTESIAN_POINT('Ctrl Pts',(14.3130086959694,-0.529905110324446,
27.0952276331628));
#47480=CARTESIAN_POINT('Ctrl Pts',(14.3448363046642,-0.750388566731274,
26.7683511880868));
#47481=CARTESIAN_POINT('Ctrl Pts',(14.376663913359,-0.787188929496858,26.3757866733952));
#47482=CARTESIAN_POINT('Ctrl Pts',(14.4084915220538,-0.631298059665474,
26.0136275901214));
#47483=CARTESIAN_POINT('Ctrl Pts',(14.4403191307486,-0.3208755434976,25.7705246770357));
#47484=CARTESIAN_POINT('Ctrl Pts',(14.4721467394435,0.0680921626112602,
25.7059856307223));
#47485=CARTESIAN_POINT('Ctrl Pts',(14.5039743481383,0.440391998718261,25.8358085752634));
#47486=CARTESIAN_POINT('Ctrl Pts',(14.5358019568331,0.704890932298469,26.128214934684));
#47487=CARTESIAN_POINT('Ctrl Pts',(14.5676295655279,0.79684386389434,26.5116283189908));
#47488=CARTESIAN_POINT('Ctrl Pts',(14.5994571742227,0.693742189705464,26.8921952771914));
#47489=CARTESIAN_POINT('Ctrl Pts',(14.6312847829175,0.42082354702301,27.1767591177809));
#47490=CARTESIAN_POINT('Ctrl Pts',(14.6631123916124,0.0448940451386551,
27.2956631736732));
#47491=CARTESIAN_POINT('Ctrl Pts',(14.6949400003072,-0.342024799417935,
27.2198016378223));
#47492=CARTESIAN_POINT('Ctrl Pts',(14.726767609002,-0.645221455172022,26.967744198269));
#47493=CARTESIAN_POINT('Ctrl Pts',(14.7585952176968,-0.790478240538743,
26.6011904761496));
#47494=CARTESIAN_POINT('Ctrl Pts',(14.7904228263916,-0.742238622687695,
26.2098669473857));
#47495=CARTESIAN_POINT('Ctrl Pts',(14.8222504350865,-0.512310886867079,
25.8895633395461));
#47496=CARTESIAN_POINT('Ctrl Pts',(14.8540780437813,-0.156977657442333,
25.71868484189));
#47497=CARTESIAN_POINT('Ctrl Pts',(14.8859056524761,0.236781186430625,25.7390597717421));
#47498=CARTESIAN_POINT('Ctrl Pts',(14.9177332611709,0.572579791078355,25.9457006728515));
#47499=CARTESIAN_POINT('Ctrl Pts',(14.9495608698657,0.768220040382449,26.2880251647402));
#47500=CARTESIAN_POINT('Ctrl Pts',(14.9813884785605,0.775812337104691,26.6822376986926));
#47501=CARTESIAN_POINT('Ctrl Pts',(15.0132160872554,0.593498208699499,27.0318413649756));
#47502=CARTESIAN_POINT('Ctrl Pts',(15.0450436959502,0.265905231604842,27.2512587896549));
#47503=CARTESIAN_POINT('Ctrl Pts',(15.076871304645,-0.126777084163142,27.2867801040696));
#47504=CARTESIAN_POINT('Ctrl Pts',(15.1086989133398,-0.488426401756141,
27.129710259799));
#47505=CARTESIAN_POINT('Ctrl Pts',(15.1405265220346,-0.730516764871153,
26.8184974371495));
#47506=CARTESIAN_POINT('Ctrl Pts',(15.1723541307294,-0.793788332927985,
26.4293215468758));
#47507=CARTESIAN_POINT('Ctrl Pts',(15.2041817394243,-0.6627532402055,26.0574466090676));
#47508=CARTESIAN_POINT('Ctrl Pts',(15.2360093481191,-0.369486777125133,
25.7939016479567));
#47509=CARTESIAN_POINT('Ctrl Pts',(15.2678369568139,0.0142241267301174,
25.7031982458306));
#47510=CARTESIAN_POINT('Ctrl Pts',(15.2996645655087,0.394453192351198,25.8075391417037));
#47511=CARTESIAN_POINT('Ctrl Pts',(15.3314921742035,0.678126438920626,26.0813833566788));
#47512=CARTESIAN_POINT('Ctrl Pts',(15.3633197828983,0.795805202493795,26.4576982162029));
#47513=CARTESIAN_POINT('Ctrl Pts',(15.3951473915932,0.718683607945039,26.8443678743723));
#47514=CARTESIAN_POINT('Ctrl Pts',(15.426975000288,0.465639785487568,27.1467417965461));
#47515=CARTESIAN_POINT('Ctrl Pts',(15.4588026089828,0.0986148069826778,
27.2908036931327));
#47516=CARTESIAN_POINT('Ctrl Pts',(15.4906302176776,-0.292549495638406,
27.2412895209231));
#47517=CARTESIAN_POINT('Ctrl Pts',(15.5224578263724,-0.612102370814474,
27.0103195556432));
#47518=CARTESIAN_POINT('Ctrl Pts',(15.5542854350672,-0.781822396609454,
26.6544315427252));
#47519=CARTESIAN_POINT('Ctrl Pts',(15.5861130437621,-0.760164831041612,
26.2607411634315));
#47520=CARTESIAN_POINT('Ctrl Pts',(15.6179406524569,-0.552431099026793,
25.9256175124043));
#47521=CARTESIAN_POINT('Ctrl Pts',(15.6497682611517,-0.209471088532158,
25.7310934879338));
#47522=CARTESIAN_POINT('Ctrl Pts',(15.6815958698465,0.184764086958111,25.7247854533105));
#47523=CARTESIAN_POINT('Ctrl Pts',(15.7134234785413,0.533771975425466,25.9082375143023));
#47524=CARTESIAN_POINT('Ctrl Pts',(15.7452510872362,0.752121039795552,26.2365435468138));
#47525=CARTESIAN_POINT('Ctrl Pts',(15.7770786959309,0.78636292888696,26.6293394962914));
#47526=CARTESIAN_POINT('Ctrl Pts',(15.8089063046258,0.628115777091278,26.9904752101765));
#47527=CARTESIAN_POINT('Ctrl Pts',(15.8407339133206,0.316115950726511,27.2315504541211));
#47528=CARTESIAN_POINT('Ctrl Pts',(15.8725615220154,-0.073263993557323,
27.2935538724477));
#47529=CARTESIAN_POINT('Ctrl Pts',(15.9043891307102,-0.444710086519647,
27.1613080221623));
#47530=CARTESIAN_POINT('Ctrl Pts',(15.9362167394051,-0.707298278273243,
26.8671845677318));
#47531=CARTESIAN_POINT('Ctrl Pts',(15.9680443480998,-0.796751188333675,
26.483180216485));
#47532=CARTESIAN_POINT('Ctrl Pts',(15.9998719567947,-0.691172178101171,
26.1032930786494));
#47533=CARTESIAN_POINT('Ctrl Pts',(16.0316995654895,-0.416405297022751,
25.8205134366008));
#47534=CARTESIAN_POINT('Ctrl Pts',(16.0635271741844,-0.0397090735252242,
25.7040612142204));
#47535=CARTESIAN_POINT('Ctrl Pts',(16.0953547828791,0.346707294700135,25.782442049009));
#47536=CARTESIAN_POINT('Ctrl Pts',(16.127182391574,0.648255274330614,26.0364695689265));
#47537=CARTESIAN_POINT('Ctrl Pts',(16.1590100002688,0.791120753270836,26.4039619087403));
#47538=CARTESIAN_POINT('Ctrl Pts',(16.1908376089636,0.740332552174896,26.7949628339619));
#47539=CARTESIAN_POINT('Ctrl Pts',(16.2226652176584,0.508322808619745,27.1137615851986));
#47540=CARTESIAN_POINT('Ctrl Pts',(16.2544928263532,0.151883789093077,27.2823213379676));
#47541=CARTESIAN_POINT('Ctrl Pts',(16.2863204350481,-0.24173394755624,27.2593813665264));
#47542=CARTESIAN_POINT('Ctrl Pts',(16.3181480437429,-0.576179088441399,
27.0505570081939));
#47543=CARTESIAN_POINT('Ctrl Pts',(16.3499756524377,-0.769584823679254,
26.706965118779));
#47544=CARTESIAN_POINT('Ctrl Pts',(16.3818032611325,-0.774608529259432,
26.3127114855973));
#47545=CARTESIAN_POINT('Ctrl Pts',(16.4136308698273,-0.590020482577639,
25.9643030788146));
#47546=CARTESIAN_POINT('Ctrl Pts',(16.4454584785221,-0.261004878818793,
25.7470246919976));
#47547=CARTESIAN_POINT('Ctrl Pts',(16.477286087217,0.131900535795971,25.7140625916236));
#47548=CARTESIAN_POINT('Ctrl Pts',(16.5091136959118,0.492518813396506,25.8734853715362));
#47549=CARTESIAN_POINT('Ctrl Pts',(16.5409413046066,0.732576379744177,26.1862688904977));
#47550=CARTESIAN_POINT('Ctrl Pts',(16.5727689133014,0.793310990324887,26.5758487564716));
#47551=CARTESIAN_POINT('Ctrl Pts',(16.6045965219962,0.659855785944694,26.9468620625921));
#47552=CARTESIAN_POINT('Ctrl Pts',(16.636424130691,0.364878461567863,27.2084906982538));
#47553=CARTESIAN_POINT('Ctrl Pts',(16.6682517393859,-0.0194152617984515,
27.2966921669241));
#47554=CARTESIAN_POINT('Ctrl Pts',(16.7000793480807,-0.398956440272542,
27.1898761627955));
#47555=CARTESIAN_POINT('Ctrl Pts',(16.7319069567755,-0.680839476780989,
26.9141895315969));
#47556=CARTESIAN_POINT('Ctrl Pts',(16.7637345654703,-0.796063922115232,
26.5371159418362));
#47557=CARTESIAN_POINT('Ctrl Pts',(16.7955621741651,-0.716424678902143,
26.1509569644296));
#47558=CARTESIAN_POINT('Ctrl Pts',(16.8273897828599,-0.461416157419982,
25.8502381275293));
#47559=CARTESIAN_POINT('Ctrl Pts',(16.8592173915548,-0.0934603563117058,
25.7085705824253));
#47560=CARTESIAN_POINT('Ctrl Pts',(16.8910450002496,0.29737304194578,25.7606322733754));
#47561=CARTESIAN_POINT('Ctrl Pts',(16.9228726089444,0.615414286049196,25.9936793330608));
#47562=CARTESIAN_POINT('Ctrl Pts',(16.9547002176392,0.782811976792353,26.3506655763249));
#47563=CARTESIAN_POINT('Ctrl Pts',(16.986527826334,0.758589843209824,26.7442064932981));
#47564=CARTESIAN_POINT('Ctrl Pts',(17.0183554350289,0.548677074193156,27.0779695742253));
#47565=CARTESIAN_POINT('Ctrl Pts',(17.0501830437237,0.204456953247554,27.270254968634));
#47566=CARTESIAN_POINT('Ctrl Pts',(17.0820106524185,-0.189810955467986,
27.273994290092));
#47567=CARTESIAN_POINT('Ctrl Pts',(17.1138382611133,-0.537616179499631,
27.0882722200051));
#47568=CARTESIAN_POINT('Ctrl Pts',(17.1456658698081,-0.753821589603515,
26.7585505304068));
#47569=CARTESIAN_POINT('Ctrl Pts',(17.1774934785029,-0.785503538757171,
26.3655398322693));
#47570=CARTESIAN_POINT('Ctrl Pts',(17.2093210871977,-0.624906846574195,
26.0054427956063));
#47571=CARTESIAN_POINT('Ctrl Pts',(17.2411486958926,-0.311342909206791,
25.7664054968385));
#47572=CARTESIAN_POINT('Ctrl Pts',(17.2729763045874,0.0784326585839467,
25.7069402585764));
#47573=CARTESIAN_POINT('Ctrl Pts',(17.3048039132822,0.449009401771598,25.8416035517627));
#47574=CARTESIAN_POINT('Ctrl Pts',(17.336631521977,0.709675400200942,26.1374313304758));
#47575=CARTESIAN_POINT('Ctrl Pts',(17.3684591306719,0.796625066564042,26.5220108860288));
#47576=CARTESIAN_POINT('Ctrl Pts',(17.4002867393666,0.688572116174983,26.9012010606094));
#47577=CARTESIAN_POINT('Ctrl Pts',(17.4321143480615,0.411970711104484,27.1821864196729));
#47578=CARTESIAN_POINT('Ctrl Pts',(17.4639419567563,0.0345198850269114,
27.296178240544));
#47579=CARTESIAN_POINT('Ctrl Pts',(17.4957695654511,-0.351370292731717,
27.2152882780459));
#47580=CARTESIAN_POINT('Ctrl Pts',(17.5275971741459,-0.651270599572141,
26.9592885385028));
#47581=CARTESIAN_POINT('Ctrl Pts',(17.5594247828408,-0.791712642528938,
26.5908975818914));
#47582=CARTESIAN_POINT('Ctrl Pts',(17.5912523915355,-0.73842722970491,26.2001897847722));
#47583=CARTESIAN_POINT('Ctrl Pts',(17.6230800002304,-0.504252400540365,
25.882996417912));
#47584=CARTESIAN_POINT('Ctrl Pts',(17.6549076089252,-0.146898168000676,
25.7165983131021));
#47585=CARTESIAN_POINT('Ctrl Pts',(17.68673521762,0.246892880351082,25.7424124008351));
#47586=CARTESIAN_POINT('Ctrl Pts',(17.7185628263148,0.579346349872695,25.9528266796507));
#47587=CARTESIAN_POINT('Ctrl Pts',(17.7503904350096,0.771677592213418,26.2987691287884));
#47588=CARTESIAN_POINT('Ctrl Pts',(17.7822180437045,0.772008340680367,26.6910250850529));
#47589=CARTESIAN_POINT('Ctrl Pts',(17.8246548552975,0.527363192762192,27.1585233970218));
#47590=CARTESIAN_POINT('Ctrl Pts',(17.8777008697889,-0.155425403013523,
27.3905262878577));
#47591=CARTESIAN_POINT('Ctrl Pts',(17.9307468842803,-0.719256274148258,
26.9409483117146));
#47592=CARTESIAN_POINT('Ctrl Pts',(17.9731836958734,-0.791074584357761,
26.4182169749722));
#47593=CARTESIAN_POINT('Ctrl Pts',(18.0050113045682,-0.657888459085232,
26.0492639960516));
#47594=CARTESIAN_POINT('Ctrl Pts',(18.036838913263,-0.35974177500854,25.7889256783384));
#47595=CARTESIAN_POINT('Ctrl Pts',(18.0686665219578,0.0243332818644455,
25.7035686117623));
#47596=CARTESIAN_POINT('Ctrl Pts',(18.1004941306526,0.403587040260669,25.8126756400868));
#47597=CARTESIAN_POINT('Ctrl Pts',(18.1323217393475,0.683447187528216,26.0902880943639));
#47598=CARTESIAN_POINT('Ctrl Pts',(18.1641493480422,0.796329325103614,26.468054034611));
#47599=CARTESIAN_POINT('Ctrl Pts',(18.1959769567371,0.71411390092001,26.8537126167479));
#47600=CARTESIAN_POINT('Ctrl Pts',(18.2278045654319,0.457184295086093,27.1527494739896));
#47601=CARTESIAN_POINT('Ctrl Pts',(18.2596321741268,0.0882959257025597,
27.2920241365189));
#47602=CARTESIAN_POINT('Ctrl Pts',(18.2914597828215,-0.302180780501247,
27.237413173922));
#47603=CARTESIAN_POINT('Ctrl Pts',(18.3232873915164,-0.618701763158597,
27.0023010116041));
#47604=CARTESIAN_POINT('Ctrl Pts',(18.3551150002112,-0.783767433557126,
26.6442305803327));
#47605=CARTESIAN_POINT('Ctrl Pts',(18.386942608906,-0.756983125763724,26.2508564207311));
#47606=CARTESIAN_POINT('Ctrl Pts',(18.4187702176008,-0.544899508122728,
25.9184677654519));
#47607=CARTESIAN_POINT('Ctrl Pts',(18.4505978262956,-0.199434270097742,
25.7284293306239));
#47608=CARTESIAN_POINT('Ctrl Pts',(18.4824254349904,0.194849834271444,25.7272587900961));
#47609=CARTESIAN_POINT('Ctrl Pts',(18.5142530436853,0.541437529129979,25.9152430383213));
#47610=CARTESIAN_POINT('Ctrl Pts',(18.5460806523801,0.755490150492264,26.2463663511633));
#47611=CARTESIAN_POINT('Ctrl Pts',(18.5779082610749,0.784610810040825,26.639575151346));
#47612=CARTESIAN_POINT('Ctrl Pts',(18.6097358697697,0.621671362865706,26.9986181728724));
#47613=CARTESIAN_POINT('Ctrl Pts',(18.6415634784645,0.306556707364476,27.2356074676479));
#47614=CARTESIAN_POINT('Ctrl Pts',(18.6733910871593,-0.0835981042838541,
27.2925318396574));
#47615=CARTESIAN_POINT('Ctrl Pts',(18.7052186958542,-0.453289446413202,
27.1554571230883));
#47616=CARTESIAN_POINT('Ctrl Pts',(18.737046304549,-0.71202279411859,26.8579370072105));
#47617=CARTESIAN_POINT('Ctrl Pts',(18.7688739132438,-0.796464376192686,
26.472799649891));
#47618=CARTESIAN_POINT('Ctrl Pts',(18.8007015219386,-0.685944244027812,
26.0943205018872));
#47619=CARTESIAN_POINT('Ctrl Pts',(18.8325291306334,-0.407515955991956,
25.8151451928656));
#47620=CARTESIAN_POINT('Ctrl Pts',(18.8643567393282,-0.0293342934702721,
25.7036113634181));
#47621=CARTESIAN_POINT('Ctrl Pts',(18.8961843480231,0.356027933769703,25.7870207074674));
#47622=CARTESIAN_POINT('Ctrl Pts',(18.9280119567179,0.654240229440685,26.0449559544106));
#47623=CARTESIAN_POINT('Ctrl Pts',(18.9598395654127,0.792305003299414,26.4142786901237));
#47624=CARTESIAN_POINT('Ctrl Pts',(18.9916671741075,0.736426211717768,26.8045846285138));
#47625=CARTESIAN_POINT('Ctrl Pts',(19.0234947828023,0.500282087197375,27.1203331318392));
#47626=CARTESIAN_POINT('Ctrl Pts',(19.0553223914972,0.141676926436067,27.2842340274076));
#47627=CARTESIAN_POINT('Ctrl Pts',(19.087150000192,-0.25160847507182,27.2561670030497));
#47628=CARTESIAN_POINT('Ctrl Pts',(19.1189776088868,-0.5833041547505,27.0430024164579));
#47629=CARTESIAN_POINT('Ctrl Pts',(19.1508052175816,-0.772216326753395,
26.6969195417532));
#47630=CARTESIAN_POINT('Ctrl Pts',(19.1826328262764,-0.772102319324263,
26.3026339195236));
#47631=CARTESIAN_POINT('Ctrl Pts',(19.2144604349712,-0.582990039655113,
25.956660350341));
#47632=CARTESIAN_POINT('Ctrl Pts',(19.2462880436661,-0.251171142649758,
25.7436876185539));
#47633=CARTESIAN_POINT('Ctrl Pts',(19.2781156523609,0.142130424215859,25.7158480353013));
#47634=CARTESIAN_POINT('Ctrl Pts',(19.3099432610557,0.500640741350412,25.8799562843406));
#47635=CARTESIAN_POINT('Ctrl Pts',(19.3417708697505,0.736602229450057,26.1958412966923));
#47636=CARTESIAN_POINT('Ctrl Pts',(19.3735984784453,0.792255298302605,26.58617948445));
#47637=CARTESIAN_POINT('Ctrl Pts',(19.4054260871402,0.653976968680098,26.9554223157297));
#47638=CARTESIAN_POINT('Ctrl Pts',(19.437253695835,0.355615559299935,27.2131850637895));
#47639=CARTESIAN_POINT('Ctrl Pts',(19.4690813045298,-0.0297948390643188,
27.2963715394172));
#47640=CARTESIAN_POINT('Ctrl Pts',(19.5009089132246,-0.407911938387894,
27.1846190267216));
#47641=CARTESIAN_POINT('Ctrl Pts',(19.5327365219194,-0.686178733351599,
26.9052827496015));
#47642=CARTESIAN_POINT('Ctrl Pts',(19.5645641306142,-0.796479972707378,
26.526739751395));
#47643=CARTESIAN_POINT('Ctrl Pts',(19.5963917393091,-0.711815681008405,
26.1416512906412));
#47644=CARTESIAN_POINT('Ctrl Pts',(19.6282193480038,-0.452910319833234,
25.8442808501979));
#47645=CARTESIAN_POINT('Ctrl Pts',(19.6600469566987,-0.0831397717704243,
25.7074199475267));
#47646=CARTESIAN_POINT('Ctrl Pts',(19.6918745653935,0.306982059827983,25.7645699379462));
#47647=CARTESIAN_POINT('Ctrl Pts',(19.7237021740883,0.621959603598031,26.0017414198222));
#47648=CARTESIAN_POINT('Ctrl Pts',(19.7555297827831,0.784691405396808,26.3608786158601));
#47649=CARTESIAN_POINT('Ctrl Pts',(19.787357391478,0.755343328467109,26.7540704968485));
#47650=CARTESIAN_POINT('Ctrl Pts',(19.8191850001728,0.54109931163992,27.0850699925406));
#47651=CARTESIAN_POINT('Ctrl Pts',(19.8510126088676,0.194402856255303,27.2728537317685));
#47652=CARTESIAN_POINT('Ctrl Pts',(19.8828402175624,-0.199880302382556,
27.2714552650336));
#47653=CARTESIAN_POINT('Ctrl Pts',(19.9146678262572,-0.545235966749666,
27.0812169145776));
#47654=CARTESIAN_POINT('Ctrl Pts',(19.9464954349521,-0.75712660569227,26.7487059793843));
#47655=CARTESIAN_POINT('Ctrl Pts',(19.9783230436469,-0.783684787055667,
26.3553158067855));
#47656=CARTESIAN_POINT('Ctrl Pts',(20.0101506523417,-0.618409493726067,
25.9973420056359));
#47657=CARTESIAN_POINT('Ctrl Pts',(20.0419782610365,-0.301757468419426,
25.7624108247258));
#47658=CARTESIAN_POINT('Ctrl Pts',(20.0738058697313,0.0887599484803642,
25.7080296515813));
#47659=CARTESIAN_POINT('Ctrl Pts',(20.1056334784261,0.457550352668162,25.8475101257477));
#47660=CARTESIAN_POINT('Ctrl Pts',(20.137461087121,0.71433976430242,26.1467096627914));
#47661=CARTESIAN_POINT('Ctrl Pts',(20.1692886958158,0.796270251327002,26.5323890117207));
#47662=CARTESIAN_POINT('Ctrl Pts',(20.2011163045106,0.683286543729253,26.9101400497234));
#47663=CARTESIAN_POINT('Ctrl Pts',(20.2329439132054,0.403045242186098,27.1874953774243));
#47664=CARTESIAN_POINT('Ctrl Pts',(20.2647715219002,0.0241449255081358,
27.2965628561519));
#47665=CARTESIAN_POINT('Ctrl Pts',(20.296599130595,-0.360665681930769,27.210644515286));
#47666=CARTESIAN_POINT('Ctrl Pts',(20.3284267392899,-0.657191111310729,
26.9507717875409));
#47667=CARTESIAN_POINT('Ctrl Pts',(20.3602543479846,-0.792846690334467,
26.5805573513361));
#47668=CARTESIAN_POINT('Ctrl Pts',(20.3920819566795,-0.734426107592801,
26.1906237667262));
#47669=CARTESIAN_POINT('Ctrl Pts',(20.4239095653743,-0.496229785355027,
25.8764205252295));
#47670=CARTESIAN_POINT('Ctrl Pts',(20.4557371740691,-0.136564365409659,
25.7148595442031));
#47671=CARTESIAN_POINT('Ctrl Pts',(20.4875647827639,0.256529822285824,25.7454883622458));
#47672=CARTESIAN_POINT('Ctrl Pts',(20.5193923914588,0.586829621236875,25.9608095356299));
#47673=CARTESIAN_POINT('Ctrl Pts',(20.5512200001536,0.773482934822817,26.3081158923556));
#47674=CARTESIAN_POINT('Ctrl Pts',(20.5830476088484,0.77080002362345,26.7023924030459));
#47675=CARTESIAN_POINT('Ctrl Pts',(20.6148752175432,0.579437621297725,27.047126497488));
#47676=CARTESIAN_POINT('Ctrl Pts',(20.646702826238,0.2462381767104,27.2579327948828));
#47677=CARTESIAN_POINT('Ctrl Pts',(20.6785304349328,-0.147236426742641,
27.2832092925066));
#47678=CARTESIAN_POINT('Ctrl Pts',(20.7103580436277,-0.504669912886847,
27.1167687088815));
#47679=CARTESIAN_POINT('Ctrl Pts',(20.7421856523225,-0.738568293385044,
26.7993530311103));
#47680=CARTESIAN_POINT('Ctrl Pts',(20.7740132610173,-0.791676993697611,
26.40866052946));
#47681=CARTESIAN_POINT('Ctrl Pts',(20.8058408697121,-0.650995855233153,
26.0403264661764));
#47682=CARTESIAN_POINT('Ctrl Pts',(20.8376684784069,-0.350961365800501,
25.7845131161621));
#47683=CARTESIAN_POINT('Ctrl Pts',(20.8694960871017,0.034982840646634,25.7038394872333));
#47684=CARTESIAN_POINT('Ctrl Pts',(20.9013236957965,0.412363808420875,25.8180531906862));
#47685=CARTESIAN_POINT('Ctrl Pts',(20.9331513044914,0.688804725407329,26.0991965425734));
#47686=CARTESIAN_POINT('Ctrl Pts',(20.9649789131862,0.796637286020959,26.4784501566183));
#47687=CARTESIAN_POINT('Ctrl Pts',(20.996806521881,0.70946580780214,26.8629788269146));
#47688=CARTESIAN_POINT('Ctrl Pts',(21.0286341305758,0.448628471403418,27.1586560983357));
#47689=CARTESIAN_POINT('Ctrl Pts',(21.0604617392707,0.0779740759816852,
27.2931049140583));
#47690=CARTESIAN_POINT('Ctrl Pts',(21.0922893479654,-0.311767123444173,
27.2334143589867));
#47691=CARTESIAN_POINT('Ctrl Pts',(21.1241169566603,-0.625192728165132,
26.9941957242612));
#47692=CARTESIAN_POINT('Ctrl Pts',(21.1559445653551,-0.785581173842449,
26.6340058973812));
#47693=CARTESIAN_POINT('Ctrl Pts',(21.1877721740499,-0.753671939737323,
26.2410135747164));
#47694=CARTESIAN_POINT('Ctrl Pts',(21.2195997827447,-0.537275894906149,
25.9114169778345));
#47695=CARTESIAN_POINT('Ctrl Pts',(21.2514273914396,-0.189363322650899,
25.7258960707611));
#47696=CARTESIAN_POINT('Ctrl Pts',(21.2832550001344,0.204902355806668,25.7298633979523));
#47697=CARTESIAN_POINT('Ctrl Pts',(21.3150826088292,0.549011221810531,25.9223478213019));
#47698=CARTESIAN_POINT('Ctrl Pts',(21.346910217524,0.758730940462114,26.2562322391823));
#47699=CARTESIAN_POINT('Ctrl Pts',(21.3787378262188,0.782725486097683,26.6497870977146));
#47700=CARTESIAN_POINT('Ctrl Pts',(21.4105654349136,0.615121378538741,27.0066764755672));
#47701=CARTESIAN_POINT('Ctrl Pts',(21.4423930436085,0.296945416897534,27.2395395733916));
#47702=CARTESIAN_POINT('Ctrl Pts',(21.4742206523033,-0.0939180232535311,
27.2913752372527));
#47703=CARTESIAN_POINT('Ctrl Pts',(21.5060482609981,-0.461791836663578,
27.1494949274779));
#47704=CARTESIAN_POINT('Ctrl Pts',(21.5378758696929,-0.716626410222027,
26.848628669792));
#47705=CARTESIAN_POINT('Ctrl Pts',(21.5697034783877,-0.79604232490086,26.4624237016852));
#47706=CARTESIAN_POINT('Ctrl Pts',(21.6015310870826,-0.6805998376932,26.0854168091196));
#47707=CARTESIAN_POINT('Ctrl Pts',(21.6333586957773,-0.398557419114277,
25.8098932365948));
#47708=CARTESIAN_POINT('Ctrl Pts',(21.6651863044722,-0.0189545325561093,
25.7032967384752));
#47709=CARTESIAN_POINT('Ctrl Pts',(21.697013913167,0.36528811976181,25.791720428934));
#47710=CARTESIAN_POINT('Ctrl Pts',(21.7288415218618,0.660114095329825,26.053519605833));
#47711=CARTESIAN_POINT('Ctrl Pts',(21.7606691305566,0.793354720904365,26.4246100268778));
#47712=CARTESIAN_POINT('Ctrl Pts',(21.7924967392514,0.732394826972873,26.8141547049655));
#47713=CARTESIAN_POINT('Ctrl Pts',(21.8243243479463,0.492156418482947,27.126799346661));
#47714=CARTESIAN_POINT('Ctrl Pts',(21.856151956641,0.131446007206347,27.2860135548564));
#47715=CARTESIAN_POINT('Ctrl Pts',(21.8879795653359,-0.261440279771059,
27.2528242433277));
#47716=CARTESIAN_POINT('Ctrl Pts',(21.9198071740307,-0.590330176718207,
27.0353556235666));
#47717=CARTESIAN_POINT('Ctrl Pts',(21.9516347827255,-0.774716708426573,
26.6868405280267));
#47718=CARTESIAN_POINT('Ctrl Pts',(21.9834623914203,-0.769465007346789,
26.2925898659722));
#47719=CARTESIAN_POINT('Ctrl Pts',(22.0152900001152,-0.575860605727061,
25.9491098802844));
#47720=CARTESIAN_POINT('Ctrl Pts',(22.04711760881,-0.241294757923752,25.7404789660404));
#47721=CARTESIAN_POINT('Ctrl Pts',(22.0789452175048,0.152336179061179,25.7177666270366));
#47722=CARTESIAN_POINT('Ctrl Pts',(22.1107728261996,0.508677661110342,25.8865324798199));
#47723=CARTESIAN_POINT('Ctrl Pts',(22.1426004348944,0.740503004985982,26.2054653486679));
#47724=CARTESIAN_POINT('Ctrl Pts',(22.1744280435892,0.791065082286333,26.5964955792559));
#47725=CARTESIAN_POINT('Ctrl Pts',(22.2062556522841,0.647987106915214,26.9639052387075));
#47726=CARTESIAN_POINT('Ctrl Pts',(22.2380832609789,0.346292273938845,27.2177583313615));
#47727=CARTESIAN_POINT('Ctrl Pts',(22.2699108696737,-0.0401693572021401,
27.2959156889838));
#47728=CARTESIAN_POINT('Ctrl Pts',(22.3017384783685,-0.416798173548772,
27.1792456431623));
#47729=CARTESIAN_POINT('Ctrl Pts',(22.3335660870633,-0.691401477599888,
26.8963071510852));
#47730=CARTESIAN_POINT('Ctrl Pts',(22.3653936957582,-0.796760781963107,
26.5163590205743));
#47731=CARTESIAN_POINT('Ctrl Pts',(22.397221304453,-0.707085817666679,26.132406464035));
#47732=CARTESIAN_POINT('Ctrl Pts',(22.4290489131478,-0.444327578628173,
25.8384349131801));
#47733=CARTESIAN_POINT('Ctrl Pts',(22.4608765218426,-0.0728050701817948,
25.7064038917784));
#47734=CARTESIAN_POINT('Ctrl Pts',(22.4927041305374,0.316538952499552,25.768632477629));
#47735=CARTESIAN_POINT('Ctrl Pts',(22.5245317392322,0.628399313207805,26.0098881103375));
#47736=CARTESIAN_POINT('Ctrl Pts',(22.5563593479271,0.786437594250266,26.3711152779478));
#47737=CARTESIAN_POINT('Ctrl Pts',(22.5881869566219,0.751968557521462,26.7638913597064));
#47738=CARTESIAN_POINT('Ctrl Pts',(22.6200145653167,0.533429670730638,27.0920710663534));
#47739=CARTESIAN_POINT('Ctrl Pts',(22.6518421740115,0.184315750545256,27.2753212658824));
#47740=CARTESIAN_POINT('Ctrl Pts',(22.6836697827063,-0.209915711095263,
27.2687852466482));
#47741=CARTESIAN_POINT('Ctrl Pts',(22.7154973914012,-0.552763171263273,
27.0740629213976));
#47742=CARTESIAN_POINT('Ctrl Pts',(22.7473250000959,-0.760303066990549,
26.7388191942734));
#47743=CARTESIAN_POINT('Ctrl Pts',(22.7791526087908,-0.78173295832624,26.3451163562699));
#47744=CARTESIAN_POINT('Ctrl Pts',(22.8109802174856,-0.611807151357293,
25.9893265517215));
#47745=CARTESIAN_POINT('Ctrl Pts',(22.8428078261804,-0.292120759998493,
25.7585414220562));
#47746=CARTESIAN_POINT('Ctrl Pts',(22.8746354348752,0.0990721111926007,
25.7092534679099));
#47747=CARTESIAN_POINT('Ctrl Pts',(22.9064630435701,0.466013717526745,25.853527590453));
#47748=CARTESIAN_POINT('Ctrl Pts',(22.9382906522649,0.718882635243795,26.1560477969637));
#47749=CARTESIAN_POINT('Ctrl Pts',(22.9701182609597,0.795780606359475,26.5427619897895));
#47750=CARTESIAN_POINT('Ctrl Pts',(23.0019458696545,0.677884240092678,26.9190087329192));
#47751=CARTESIAN_POINT('Ctrl Pts',(23.0337734783493,0.394052677220659,27.1926888542512));
#47752=CARTESIAN_POINT('Ctrl Pts',(23.0656010870442,0.0137633349813457,
27.2968098467256));
#47753=CARTESIAN_POINT('Ctrl Pts',(23.0974286957389,-0.369895051057782,
27.2058845602728));
#47754=CARTESIAN_POINT('Ctrl Pts',(23.1292563044338,-0.663009057407268,
26.9421700476339));
#47755=CARTESIAN_POINT('Ctrl Pts',(23.1610839131286,-0.793829073448207,
26.5702193945928));
#47756=CARTESIAN_POINT('Ctrl Pts',(23.1929115218234,-0.730332456083478,
26.1810801592568));
#47757=CARTESIAN_POINT('Ctrl Pts',(23.2247391305182,-0.488062159497627,
25.8700073891742));
#47758=CARTESIAN_POINT('Ctrl Pts',(23.2565667392131,-0.126322069100469,
25.7131467124763));
#47759=CARTESIAN_POINT('Ctrl Pts',(23.2883943479078,0.266339639077475,25.7488951086002));
#47760=CARTESIAN_POINT('Ctrl Pts',(23.3202219566027,0.593805672595626,25.9685019431627));
#47761=CARTESIAN_POINT('Ctrl Pts',(23.3520495652975,0.775917595190683,26.3182109829992));
#47762=CARTESIAN_POINT('Ctrl Pts',(23.3838771739923,0.768097327165974,26.7124190604186));
#47763=CARTESIAN_POINT('Ctrl Pts',(23.4157047826871,0.572259144787906,27.0546303565756));
#47764=CARTESIAN_POINT('Ctrl Pts',(23.4475323913819,0.236341096138676,27.2610770312554));
#47765=CARTESIAN_POINT('Ctrl Pts',(23.4793600000768,-0.157429464686238,
27.281224247497));
#47766=CARTESIAN_POINT('Ctrl Pts',(23.5111876087716,-0.512663815891357,
27.1101402896911));
#47767=CARTESIAN_POINT('Ctrl Pts',(23.5430152174664,-0.742406282124077,
26.7897037685142));
#47768=CARTESIAN_POINT('Ctrl Pts',(23.5748428261612,-0.790419590044506,
26.39835240828));
#47769=CARTESIAN_POINT('Ctrl Pts',(23.6066704348561,-0.644950851448086,
26.0318827492551));
#47770=CARTESIAN_POINT('Ctrl Pts',(23.6384980435508,-0.341608481918587,
25.7800006900629));
#47771=CARTESIAN_POINT('Ctrl Pts',(23.6703256522457,0.0453541685624505,
25.7043629215386));
#47772=CARTESIAN_POINT('Ctrl Pts',(23.7021532609405,0.421214845532138,25.8234843570678));
#47773=CARTESIAN_POINT('Ctrl Pts',(23.7339808696353,0.693968879696766,26.1082059785538));
#47774=CARTESIAN_POINT('Ctrl Pts',(23.7658084783301,0.796850455291405,26.4888324966759));
#47775=CARTESIAN_POINT('Ctrl Pts',(23.797636087025,0.704675811632944,26.8721926406151));
#47776=CARTESIAN_POINT('Ctrl Pts',(23.8294636957197,0.440007824081036,27.1644459917676));
#47777=CARTESIAN_POINT('Ctrl Pts',(23.8612913044146,0.0676329737958395,
27.2940536141119));
#47778=CARTESIAN_POINT('Ctrl Pts',(23.8931189131094,-0.321297344429241,
27.229289639095));
#47779=CARTESIAN_POINT('Ctrl Pts',(23.9249465218042,-0.631579222606048,
26.9860072497412));
#47780=CARTESIAN_POINT('Ctrl Pts',(23.956774130499,-0.787260630265086,26.6237580755475));
#47781=CARTESIAN_POINT('Ctrl Pts',(23.9886017391939,-0.750233254128349,
26.2312149080983));
#47782=CARTESIAN_POINT('Ctrl Pts',(24.0204293478886,-0.529560802386153,
25.9044660229636));
#47783=CARTESIAN_POINT('Ctrl Pts',(24.0522569565835,-0.179260354208531,
25.7234943099773));
#47784=CARTESIAN_POINT('Ctrl Pts',(24.0840845652783,0.214920155430682,25.7325987437994));
#47785=CARTESIAN_POINT('Ctrl Pts',(24.1159121739731,0.556491655837079,25.9295507049594));
#47786=CARTESIAN_POINT('Ctrl Pts',(24.1477397826679,0.761842918540557,26.2661395101813));
#47787=CARTESIAN_POINT('Ctrl Pts',(24.1795673913627,0.780707245874303,26.6599736149119));
#47788=CARTESIAN_POINT('Ctrl Pts',(24.2113950000576,0.608466952871163,27.0146487428259));
#47789=CARTESIAN_POINT('Ctrl Pts',(24.2432226087524,0.287283702529686,27.2433461074691));
#47790=CARTESIAN_POINT('Ctrl Pts',(24.2750502174472,-0.104221993505796,
27.2900842596193));
#47791=CARTESIAN_POINT('Ctrl Pts',(24.306877826142,-0.470215816038203,27.1434224487661));
#47792=CARTESIAN_POINT('Ctrl Pts',(24.3387054348368,-0.721108343590642,
26.8392611354584));
#47793=CARTESIAN_POINT('Ctrl Pts',(24.3705330435317,-0.795485106812842,
26.4520541339887));
#47794=CARTESIAN_POINT('Ctrl Pts',(24.4023606522264,-0.675139866205197,
26.076583512025));
#47795=CARTESIAN_POINT('Ctrl Pts',(24.4341882609213,-0.389531207732191,
25.8047584596478));
#47796=CARTESIAN_POINT('Ctrl Pts',(24.4660158696161,-0.00857155315095306,
25.7031173927703));
#47797=CARTESIAN_POINT('Ctrl Pts',(24.4978434783109,0.37448628025374,25.7965404154251));
#47798=CARTESIAN_POINT('Ctrl Pts',(24.5296710870057,0.66587587465148,26.0621590690836));
#47799=CARTESIAN_POINT('Ctrl Pts',(24.5614986957005,0.79426972782966,26.4349541647604));
#47800=CARTESIAN_POINT('Ctrl Pts',(24.5933263043954,0.728239082472559,26.8236714383262));
#47801=CARTESIAN_POINT('Ctrl Pts',(24.6251539130902,0.483947182200952,27.1331591317105));
#47802=CARTESIAN_POINT('Ctrl Pts',(24.656981521785,0.121192768603945,27.2876596181516));
#47803=CARTESIAN_POINT('Ctrl Pts',(24.6888091304798,-0.271227692226556,
27.2493536549575));
#47804=CARTESIAN_POINT('Ctrl Pts',(24.7206367391747,-0.597255961333821,
27.0276179279363));
#47805=CARTESIAN_POINT('Ctrl Pts',(24.7524643478694,-0.777085544137324,
26.676729789004));
#47806=CARTESIAN_POINT('Ctrl Pts',(24.7842919565643,-0.766697041139229,
26.2825810304114));
#47807=CARTESIAN_POINT('Ctrl Pts',(24.8161195652591,-0.568633391362849,
25.9416529507056));
#47808=CARTESIAN_POINT('Ctrl Pts',(24.8479471739539,-0.231377401638892,
25.7373992792821));
#47809=CARTESIAN_POINT('Ctrl Pts',(24.8797747826487,0.16251606740706,25.7198180410551));
#47810=CARTESIAN_POINT('Ctrl Pts',(24.9116023913435,0.516628208017037,25.8932128413441));
#47811=CARTESIAN_POINT('Ctrl Pts',(24.9434300000383,0.744278044004932,26.2151394122719));
#47812=CARTESIAN_POINT('Ctrl Pts',(24.9752576087332,0.78974054437337,26.6067952892288));
#47813=CARTESIAN_POINT('Ctrl Pts',(25.007085217428,0.641887217721265,26.9723093911354));
#47814=CARTESIAN_POINT('Ctrl Pts',(25.0389128261228,0.336910188567394,27.2222097244347));
#47815=CARTESIAN_POINT('Ctrl Pts',(25.0707404348176,-0.0505370546315667,
27.2953246930265));
#47816=CARTESIAN_POINT('Ctrl Pts',(25.1025680435124,-0.425613636882587,
27.1737569245123));
#47817=CARTESIAN_POINT('Ctrl Pts',(25.1343956522073,-0.696506822711343,
26.8872642600927));
#47818=CARTESIAN_POINT('Ctrl Pts',(25.1662232609021,-0.796906302199207,
26.5059755120117));
#47819=CARTESIAN_POINT('Ctrl Pts',(25.1980508695969,-0.702235892006071,
26.1232240543678));
#47820=CARTESIAN_POINT('Ctrl Pts',(25.2298784782917,-0.435669391136255,
25.832701309116));
#47821=CARTESIAN_POINT('Ctrl Pts',(25.2617060869866,-0.0624580063800852,
25.705522587692));
#47822=CARTESIAN_POINT('Ctrl Pts',(25.2935336956813,0.326042097238796,25.7728192026347));
#47823=CARTESIAN_POINT('Ctrl Pts',(25.3253613043762,0.634732321372251,26.0181180212604));
#47824=CARTESIAN_POINT('Ctrl Pts',(25.357188913071,0.78805024694888,26.3813738245058));
#47825=CARTESIAN_POINT('Ctrl Pts',(25.3890165217658,0.748466103221927,26.7736674141299));
#47826=CARTESIAN_POINT('Ctrl Pts',(25.4208441304606,0.525669454106653,27.0989716072131));
#47827=CARTESIAN_POINT('Ctrl Pts',(25.4526717391554,0.174197348243338,27.2776571513812));
#47828=CARTESIAN_POINT('Ctrl Pts',(25.4844993478503,-0.219915476373876,
27.2659846894545));
#47829=CARTESIAN_POINT('Ctrl Pts',(25.5163269565451,-0.560196517256405,
27.0668114530277));
#47830=CARTESIAN_POINT('Ctrl Pts',(25.5481545652399,-0.763350429746691,
26.7288918579483));
#47831=CARTESIAN_POINT('Ctrl Pts',(25.5799821739347,-0.779648392280715,
26.3349432048161));
#47832=CARTESIAN_POINT('Ctrl Pts',(25.6118097826295,-0.605100924877577,
25.9813978095313));
#47833=CARTESIAN_POINT('Ctrl Pts',(25.6436373913244,-0.282434449814925,
25.7547979181797));
#47834=CARTESIAN_POINT('Ctrl Pts',(25.6754650000191,0.109367451560953,25.710611552006));
#47835=CARTESIAN_POINT('Ctrl Pts',(25.707292608714,0.474397953853924,25.8596548254688));
#47836=CARTESIAN_POINT('Ctrl Pts',(25.7391202174087,0.723303440713549,26.1654443336632));
#47837=CARTESIAN_POINT('Ctrl Pts',(25.7709478261036,0.795155838932149,26.553127707192));
#47838=CARTESIAN_POINT('Ctrl Pts',(25.8027754347984,0.672366832289694,26.9278062684317));
#47839=CARTESIAN_POINT('Ctrl Pts',(25.8346030434933,0.384993203039443,27.1977647143017));
#47840=CARTESIAN_POINT('Ctrl Pts',(25.8664306521881,0.00337940660061129,
27.2969215381445));
#47841=CARTESIAN_POINT('Ctrl Pts',(25.8982582608829,-0.379061610834525,
27.2010047503193));
#47842=CARTESIAN_POINT('Ctrl Pts',(25.9300858695777,-0.668714428418505,
26.9334932213543));
#47843=CARTESIAN_POINT('Ctrl Pts',(25.9619134782725,-0.794676659578473,
26.5598695268258));
#47844=CARTESIAN_POINT('Ctrl Pts',(25.9937410869674,-0.726114805888509,
26.1715906810597));
#47845=CARTESIAN_POINT('Ctrl Pts',(26.0255686956621,-0.479811640722421,
25.8637012684045));
#47846=CARTESIAN_POINT('Ctrl Pts',(26.057396304357,-0.116058362262509,25.7115674057289));
#47847=CARTESIAN_POINT('Ctrl Pts',(26.0892239130518,0.276104304993651,25.7524295460381));
#47848=CARTESIAN_POINT('Ctrl Pts',(26.1210515217466,0.600680758111244,25.9762843069252));
#47849=CARTESIAN_POINT('Ctrl Pts',(26.1528791304414,0.778220766932473,26.3283374916096));
#47850=CARTESIAN_POINT('Ctrl Pts',(26.1847067391362,0.765263715417021,26.7224086099901));
#47851=CARTESIAN_POINT('Ctrl Pts',(26.216534347831,0.564984430859093,27.0620420026143));
#47852=CARTESIAN_POINT('Ctrl Pts',(26.2483619565259,0.226402125810272,27.2640883311776));
#47853=CARTESIAN_POINT('Ctrl Pts',(26.2801895652207,-0.167592445455861,
27.2791135571752));
#47854=CARTESIAN_POINT('Ctrl Pts',(26.3120171739155,-0.520576980781025,
27.1033949839955));
#47855=CARTESIAN_POINT('Ctrl Pts',(26.3438447826103,-0.746106034620935,
26.7800308690168));
#47856=CARTESIAN_POINT('Ctrl Pts',(26.3756723913052,-0.789053050339413,
26.3880094871026));
#47857=CARTESIAN_POINT('Ctrl Pts',(26.3968907971017,-0.688841172942706,
26.1451000824837));
#47858=CARTESIAN_POINT('Ctrl Pts',(26.4075,-0.612682133358295,26.0429972363724));
#47859=CARTESIAN_POINT('Ctrl Pts',(9.55924498047908,-0.761351629614349,
26.8558316825899));
#47860=CARTESIAN_POINT('Ctrl Pts',(9.56985418337735,-0.820650612807892,
26.7289532181421));
#47861=CARTESIAN_POINT('Ctrl Pts',(9.59107258917389,-0.874534777171298,
26.4451092594775));
#47862=CARTESIAN_POINT('Ctrl Pts',(9.62290019786871,-0.74110841331227,26.0325432712716));
#47863=CARTESIAN_POINT('Ctrl Pts',(9.65472780656354,-0.426351906614665,
25.7345101228801));
#47864=CARTESIAN_POINT('Ctrl Pts',(9.68655541525833,-0.00719023871993623,
25.6238023694641));
#47865=CARTESIAN_POINT('Ctrl Pts',(9.71838302395318,0.413709994658858,25.7276021956329));
#47866=CARTESIAN_POINT('Ctrl Pts',(9.75021063264797,0.73335200291761,26.0204575958235));
#47867=CARTESIAN_POINT('Ctrl Pts',(9.78203824134281,0.873475187765602,26.4307052449264));
#47868=CARTESIAN_POINT('Ctrl Pts',(9.81386585003761,0.799788828170189,26.8579109271115));
#47869=CARTESIAN_POINT('Ctrl Pts',(9.84569345873243,0.530325298043976,27.1975079818376));
#47870=CARTESIAN_POINT('Ctrl Pts',(9.87752106742726,0.131047527412838,27.3663650810967));
#47871=CARTESIAN_POINT('Ctrl Pts',(9.90934867612206,-0.300309049971829,
27.3231505205938));
#47872=CARTESIAN_POINT('Ctrl Pts',(9.94117628481689,-0.658154535135611,
27.0784415750344));
#47873=CARTESIAN_POINT('Ctrl Pts',(9.97300389351169,-0.85489447176523,26.6921395788655));
#47874=CARTESIAN_POINT('Ctrl Pts',(10.0048315022065,-0.842369874069455,
26.2588048005306));
#47875=CARTESIAN_POINT('Ctrl Pts',(10.0366591109013,-0.62364667017783,25.8845107902855));
#47876=CARTESIAN_POINT('Ctrl Pts',(10.0684867195962,-0.252264737770291,
25.6608786472305));
#47877=CARTESIAN_POINT('Ctrl Pts',(10.100314328291,0.180867548628353,25.6426499754042));
#47878=CARTESIAN_POINT('Ctrl Pts',(10.1321419369858,0.569726363653874,25.8342868403763));
#47879=CARTESIAN_POINT('Ctrl Pts',(10.1639695456806,0.819125293709173,26.1888796204097));
#47880=CARTESIAN_POINT('Ctrl Pts',(10.1957971543754,0.868015482644472,26.6196296805679));
#47881=CARTESIAN_POINT('Ctrl Pts',(10.2276247630702,0.704429393468763,27.0210963134763));
#47882=CARTESIAN_POINT('Ctrl Pts',(10.2594523717651,0.368410280050912,27.2950069205873));
#47883=CARTESIAN_POINT('Ctrl Pts',(10.2912799804599,-0.0577897651425869,
27.3743125764966));
#47884=CARTESIAN_POINT('Ctrl Pts',(10.3231075891547,-0.469843801982232,
27.2396005273108));
#47885=CARTESIAN_POINT('Ctrl Pts',(10.3549351978495,-0.766887606984555,
26.9238461237048));
#47886=CARTESIAN_POINT('Ctrl Pts',(10.3867628065443,-0.876209617709942,
26.5043409825269));
#47887=CARTESIAN_POINT('Ctrl Pts',(10.4185904152391,-0.771049558237124,
26.0837732384293));
#47888=CARTESIAN_POINT('Ctrl Pts',(10.450418023934,-0.477148925554562,25.7650911341209));
#47889=CARTESIAN_POINT('Ctrl Pts',(10.4822456326288,-0.0664498838138394,
25.6263029408061));
#47890=CARTESIAN_POINT('Ctrl Pts',(10.5140732413236,0.360515024404849,25.7013817836515));
#47891=CARTESIAN_POINT('Ctrl Pts',(10.5459008500184,0.699231633110719,25.9719495653243));
#47892=CARTESIAN_POINT('Ctrl Pts',(10.5777284587132,0.866787545564904,26.3717756296248));
#47893=CARTESIAN_POINT('Ctrl Pts',(10.609556067408,0.822167760043173,26.8029889645678));
#47894=CARTESIAN_POINT('Ctrl Pts',(10.6413836761029,0.576294484860074,27.1600354573993));
#47895=CARTESIAN_POINT('Ctrl Pts',(10.6732112847977,0.189353556835892,27.3555158495422));
#47896=CARTESIAN_POINT('Ctrl Pts',(10.7050388934925,-0.243938086875568,
27.3415796742293));
#47897=CARTESIAN_POINT('Ctrl Pts',(10.7368665021873,-0.617517596846251,
27.121638283803));
#47898=CARTESIAN_POINT('Ctrl Pts',(10.7686941108822,-0.839938696900418,
26.7495298053411));
#47899=CARTESIAN_POINT('Ctrl Pts',(10.8005217195769,-0.856756266789251,
26.3163404300841));
#47900=CARTESIAN_POINT('Ctrl Pts',(10.8323493282718,-0.663853634961942,
25.9281079737816));
#47901=CARTESIAN_POINT('Ctrl Pts',(10.8641769369666,-0.308450273777893,
25.6798655190088));
#47902=CARTESIAN_POINT('Ctrl Pts',(10.8960045456614,0.122456770476399,25.6323788397758));
#47903=CARTESIAN_POINT('Ctrl Pts',(10.9278321543562,0.523388360098695,25.7972719140254));
#47904=CARTESIAN_POINT('Ctrl Pts',(10.9596597630511,0.796202868223438,26.1341815601461));
#47905=CARTESIAN_POINT('Ctrl Pts',(10.9914873717458,0.874119676029564,26.5606376968752));
#47906=CARTESIAN_POINT('Ctrl Pts',(11.0233149804407,0.738065997844413,26.9722506973317));
#47907=CARTESIAN_POINT('Ctrl Pts',(11.0551425891355,0.421345593371013,27.2682642964835));
#47908=CARTESIAN_POINT('Ctrl Pts',(11.0869701978303,0.00148654111727426,
27.3762191098691));
#47909=CARTESIAN_POINT('Ctrl Pts',(11.1187978065251,-0.418736392575163,
27.2696895295101));
#47910=CARTESIAN_POINT('Ctrl Pts',(11.1506254152199,-0.736459369020887,
26.9747522891842));
#47911=CARTESIAN_POINT('Ctrl Pts',(11.1824530239148,-0.873908896162748,
26.5636032979645));
#47912=CARTESIAN_POINT('Ctrl Pts',(11.2142806326096,-0.79743953284627,26.1368852388593));
#47913=CARTESIAN_POINT('Ctrl Pts',(11.2461082413044,-0.525769753533207,
25.7990518531489));
#47914=CARTESIAN_POINT('Ctrl Pts',(11.2779358499992,-0.125399965779644,
25.6327993387417));
#47915=CARTESIAN_POINT('Ctrl Pts',(11.309763458694,0.305665723641568,25.6788236464102));
#47916=CARTESIAN_POINT('Ctrl Pts',(11.3415910673888,0.661909343234156,25.9258587633311));
#47917=CARTESIAN_POINT('Ctrl Pts',(11.3734186760837,0.856128164921163,26.3134344524488));
#47918=CARTESIAN_POINT('Ctrl Pts',(11.4052462847785,0.840780534161899,26.7466783972681));
#47919=CARTESIAN_POINT('Ctrl Pts',(11.4370738934733,0.61962330496895,27.1195394242853));
#47920=CARTESIAN_POINT('Ctrl Pts',(11.4689015021681,0.246792222262105,27.3407471304354));
#47921=CARTESIAN_POINT('Ctrl Pts',(11.5007291108629,-0.186449640781078,
27.3561534148486));
#47922=CARTESIAN_POINT('Ctrl Pts',(11.5325567195578,-0.574051620242147,
27.1619870660381));
#47923=CARTESIAN_POINT('Ctrl Pts',(11.5643843282526,-0.821134964171277,
26.8057768940254));
#47924=CARTESIAN_POINT('Ctrl Pts',(11.5962119369474,-0.867217630314253,
26.3747174394559));
#47925=CARTESIAN_POINT('Ctrl Pts',(11.6280395456422,-0.701019320628618,
25.9743251476343));
#47926=CARTESIAN_POINT('Ctrl Pts',(11.659867154337,-0.363222717439855,25.7026096339684));
#47927=CARTESIAN_POINT('Ctrl Pts',(11.6916947630318,0.0634849851154085,
25.626082501051));
#47928=CARTESIAN_POINT('Ctrl Pts',(11.7235223717267,0.474652580874319,25.7634763644161));
#47929=CARTESIAN_POINT('Ctrl Pts',(11.7553499804215,0.769632832735413,26.0811594085096));
#47930=CARTESIAN_POINT('Ctrl Pts',(11.7871775891163,0.876219303091394,26.5013679160741));
#47931=CARTESIAN_POINT('Ctrl Pts',(11.8190051978111,0.76832133240493,26.9212415797091));
#47932=CARTESIAN_POINT('Ctrl Pts',(11.8508328065059,0.472350614473056,27.2380020564411));
#47933=CARTESIAN_POINT('Ctrl Pts',(11.8826604152007,0.0607560371216617,
27.3741114587154));
#47934=CARTESIAN_POINT('Ctrl Pts',(11.9144880238956,-0.365710644297763,
27.2962523864653));
#47935=CARTESIAN_POINT('Ctrl Pts',(11.9463156325904,-0.702657221733247,
27.0234834926246));
#47936=CARTESIAN_POINT('Ctrl Pts',(11.9781432412852,-0.867604573728051,
26.6225742303689));
#47937=CARTESIAN_POINT('Ctrl Pts',(12.00997084998,-0.820176232348615,26.1916607611821));
#47938=CARTESIAN_POINT('Ctrl Pts',(12.0417984586748,-0.571981895366318,
25.8362237954871));
#47939=CARTESIAN_POINT('Ctrl Pts',(12.0736260673696,-0.183775558327402,
25.6432686054161));
#47940=CARTESIAN_POINT('Ctrl Pts',(12.1054536760645,0.249416089770113,25.6600275287438));
#47941=CARTESIAN_POINT('Ctrl Pts',(12.1372812847593,0.621554676821614,25.882398249658));
#47942=CARTESIAN_POINT('Ctrl Pts',(12.1691088934541,0.841546641486399,26.2559479799154));
#47943=CARTESIAN_POINT('Ctrl Pts',(12.2009365021489,0.855541476923898,26.6892377329373));
#47944=CARTESIAN_POINT('Ctrl Pts',(12.2327641108438,0.660113471733214,27.0762051221055));
#47945=CARTESIAN_POINT('Ctrl Pts',(12.2645917195385,0.303100269195515,27.3221267330029));
#47946=CARTESIAN_POINT('Ctrl Pts',(12.2964193282334,-0.128107021042431,
27.3668048970004));
#47947=CARTESIAN_POINT('Ctrl Pts',(12.3282469369282,-0.527955765874044,
27.1993031156693));
#47948=CARTESIAN_POINT('Ctrl Pts',(12.360074545623,-0.798569401482301,26.860623140301));
#47949=CARTESIAN_POINT('Ctrl Pts',(12.3919021543178,-0.873706047361805,
26.4336684003829));
#47950=CARTESIAN_POINT('Ctrl Pts',(12.4237297630126,-0.734973456918116,
26.0229505728646));
#47951=CARTESIAN_POINT('Ctrl Pts',(12.4555573717074,-0.41633114463659,25.7290067987914));
#47952=CARTESIAN_POINT('Ctrl Pts',(12.4873849804023,0.00422235874845611,
25.623789802621));
#47953=CARTESIAN_POINT('Ctrl Pts',(12.5192125890971,0.423742296389348,25.7330550185607));
#47954=CARTESIAN_POINT('Ctrl Pts',(12.5510401977919,0.739536911766215,26.0300560730899));
#47955=CARTESIAN_POINT('Ctrl Pts',(12.5828678064867,0.874304744703109,26.4420918684986));
#47956=CARTESIAN_POINT('Ctrl Pts',(12.6146954151816,0.795056789803791,26.8683026463267));
#47957=CARTESIAN_POINT('Ctrl Pts',(12.6465230238764,0.521191676213231,27.2043588396197));
#47958=CARTESIAN_POINT('Ctrl Pts',(12.6783506325712,0.119747194131051,27.3679992786875));
#47959=CARTESIAN_POINT('Ctrl Pts',(12.710178241266,-0.311009481723835,27.3191674069336));
#47960=CARTESIAN_POINT('Ctrl Pts',(12.7420058499608,-0.665636021423207,
27.0698164838685));
#47961=CARTESIAN_POINT('Ctrl Pts',(12.7738334586556,-0.857325532128846,
26.6809836187735));
#47962=CARTESIAN_POINT('Ctrl Pts',(12.8056610673504,-0.839155494087598,
26.2478488646725));
#47963=CARTESIAN_POINT('Ctrl Pts',(12.8374886760453,-0.615573641376133,
25.8764366669317));
#47964=CARTESIAN_POINT('Ctrl Pts',(12.8693162847401,-0.241309227888843,
25.6576627784313));
#47965=CARTESIAN_POINT('Ctrl Pts',(12.9011438934349,0.192023816795586,25.6450795404907));
#47966=CARTESIAN_POINT('Ctrl Pts',(12.9329715021297,0.578352508954422,25.841767128069));
#47967=CARTESIAN_POINT('Ctrl Pts',(12.9647991108245,0.823109776960734,26.1995795723057));
#47968=CARTESIAN_POINT('Ctrl Pts',(12.9966267195193,0.866382964663031,26.6309301219966));
#47969=CARTESIAN_POINT('Ctrl Pts',(13.0284543282142,0.697579489309818,27.0302310764173));
#47970=CARTESIAN_POINT('Ctrl Pts',(13.060281936909,0.35801973602548,27.299739962063));
#47971=CARTESIAN_POINT('Ctrl Pts',(13.0921095456038,-0.0691775101703559,
27.3734853235121));
#47972=CARTESIAN_POINT('Ctrl Pts',(13.1239371542986,-0.479441210678199,
27.2334154782984));
#47973=CARTESIAN_POINT('Ctrl Pts',(13.1557647629934,-0.772345387466099,
26.9138172794413));
#47974=CARTESIAN_POINT('Ctrl Pts',(13.1875923716883,-0.876191792828601,
26.4929232433873));
#47975=CARTESIAN_POINT('Ctrl Pts',(13.2194199803831,-0.765560491220048,
26.0737614839233));
#47976=CARTESIAN_POINT('Ctrl Pts',(13.2512475890779,-0.467532252036404,
25.7589360812925));
#47977=CARTESIAN_POINT('Ctrl Pts',(13.2830751977727,-0.0550596113273092,
25.6255112479255));
#47978=CARTESIAN_POINT('Ctrl Pts',(13.3149028064675,0.370890739719697,25.7061472444499));
#47979=CARTESIAN_POINT('Ctrl Pts',(13.3467304151623,0.706052982451886,25.9811056713789));
#47980=CARTESIAN_POINT('Ctrl Pts',(13.3785580238572,0.868384771947934,26.3830811129317));
#47981=CARTESIAN_POINT('Ctrl Pts',(13.410385632552,0.818149888050798,26.8136764240213));
#47982=CARTESIAN_POINT('Ctrl Pts',(13.4422132412468,0.567645025155941,27.1674887742277));
#47983=CARTESIAN_POINT('Ctrl Pts',(13.4740408499416,0.17818975851907,27.3579105712504));
#47984=CARTESIAN_POINT('Ctrl Pts',(13.5058684586364,-0.254883504914502,
27.3383296113265));
#47985=CARTESIAN_POINT('Ctrl Pts',(13.5376960673312,-0.625565371708389,
27.1135389995947));
#47986=CARTESIAN_POINT('Ctrl Pts',(13.5695236760261,-0.843118862292117,
26.7385638747833));
#47987=CARTESIAN_POINT('Ctrl Pts',(13.6013512847209,-0.854290369195441,
26.3051921372114));
#47988=CARTESIAN_POINT('Ctrl Pts',(13.6331788934157,-0.656345286589309,
25.9195062420005));
#47989=CARTESIAN_POINT('Ctrl Pts',(13.6650065021105,-0.297737397961583,
25.6759159143877));
#47990=CARTESIAN_POINT('Ctrl Pts',(13.6968341108053,0.133751833446335,25.6340481622203));
#47991=CARTESIAN_POINT('Ctrl Pts',(13.7286617195001,0.532500759848507,25.8041515401575));
#47992=CARTESIAN_POINT('Ctrl Pts',(13.760489328195,0.800902035351146,26.1445874677579));
#47993=CARTESIAN_POINT('Ctrl Pts',(13.7923169368898,0.873255329742221,26.5720226865728));
#47994=CARTESIAN_POINT('Ctrl Pts',(13.8241445455846,0.731849716259112,26.9818279061198));
#47995=CARTESIAN_POINT('Ctrl Pts',(13.8559721542794,0.411299022583071,27.2736893771576));
#47996=CARTESIAN_POINT('Ctrl Pts',(13.8877997629742,-0.00993107937442886,
27.3761640896355));
#47997=CARTESIAN_POINT('Ctrl Pts',(13.9196273716691,-0.428730212279938,
27.2641678764399));
#47998=CARTESIAN_POINT('Ctrl Pts',(13.9514549803639,-0.742583061059497,
26.9651156154462));
#47999=CARTESIAN_POINT('Ctrl Pts',(13.9832825890587,-0.874663478876854,
26.5522105068295));
#48000=CARTESIAN_POINT('Ctrl Pts',(14.0151101977535,-0.792640296482183,
26.1265251029895));
#48001=CARTESIAN_POINT('Ctrl Pts',(14.0469378064483,-0.516591474228984,
25.7922603677493));
#48002=CARTESIAN_POINT('Ctrl Pts',(14.0787654151431,-0.11408933919623,25.6312389505819));
#48003=CARTESIAN_POINT('Ctrl Pts',(14.110593023838,0.31634003740729,25.6828763135011));
#48004=CARTESIAN_POINT('Ctrl Pts',(14.1424206325327,0.669334443264024,25.9345324577265));
#48005=CARTESIAN_POINT('Ctrl Pts',(14.1742482412276,0.858486505740013,26.3246059927858));
#48006=CARTESIAN_POINT('Ctrl Pts',(14.2060758499224,0.837494831737601,26.7576131695336));
#48007=CARTESIAN_POINT('Ctrl Pts',(14.2379034586172,0.61149784659057,27.127560771495));
#48008=CARTESIAN_POINT('Ctrl Pts',(14.269731067312,0.235815989902934,27.3438915553615));
#48009=CARTESIAN_POINT('Ctrl Pts',(14.3015586760069,-0.197589841370465,
27.3536512126692));
#48010=CARTESIAN_POINT('Ctrl Pts',(14.3333862847017,-0.582628846516562,
27.1544507357404));
#48011=CARTESIAN_POINT('Ctrl Pts',(14.3652138933965,-0.82504964861758,26.7950512084713));
#48012=CARTESIAN_POINT('Ctrl Pts',(14.3970415020913,-0.865511520925932,
26.363427874554));
#48013=CARTESIAN_POINT('Ctrl Pts',(14.4288691107861,-0.694110045637806,
25.9652352079194));
#48014=CARTESIAN_POINT('Ctrl Pts',(14.4606967194809,-0.352801556619993,
25.697944390986));
#48015=CARTESIAN_POINT('Ctrl Pts',(14.4925243281758,0.0748670986296862,
25.6269839315069));
#48016=CARTESIAN_POINT('Ctrl Pts',(14.5243519368706,0.484209488131278,25.7697238125832));
#48017=CARTESIAN_POINT('Ctrl Pts',(14.5561795455654,0.775025156020058,26.0912235992129));
#48018=CARTESIAN_POINT('Ctrl Pts',(14.5880071542602,0.876127088093716,26.5127852967419));
#48019=CARTESIAN_POINT('Ctrl Pts',(14.619834762955,0.762767151878309,26.9312173585558));
#48020=CARTESIAN_POINT('Ctrl Pts',(14.6516623716498,0.462694042786029,27.2440943227002));
#48021=CARTESIAN_POINT('Ctrl Pts',(14.6834899803447,0.0493608482442458,
27.3748289232558));
#48022=CARTESIAN_POINT('Ctrl Pts',(14.7153175890395,-0.376055090774514,
27.2914194254673));
#48023=CARTESIAN_POINT('Ctrl Pts',(14.7471451977343,-0.709418771116283,
27.0142831374761));
#48024=CARTESIAN_POINT('Ctrl Pts',(14.7789728064291,-0.869128107104919,
26.6112585805436));
#48025=CARTESIAN_POINT('Ctrl Pts',(14.8108004151239,-0.816088813168395,
26.1809997063861));
#48026=CARTESIAN_POINT('Ctrl Pts',(14.8426280238187,-0.56328405832972,25.8288269910552));
#48027=CARTESIAN_POINT('Ctrl Pts',(14.8744556325136,-0.172596394528967,
25.6409466705146));
#48028=CARTESIAN_POINT('Ctrl Pts',(14.9062832412084,0.260340100216139,25.6633488358199));
#48029=CARTESIAN_POINT('Ctrl Pts',(14.9381108499032,0.629549511251965,25.8905497959745));
#48030=CARTESIAN_POINT('Ctrl Pts',(14.969938458598,0.844655292576574,26.26693439759));
#48031=CARTESIAN_POINT('Ctrl Pts',(15.0017660672929,0.853002996713588,26.7003697230172));
#48032=CARTESIAN_POINT('Ctrl Pts',(15.0335936759876,0.652549239490231,27.0847577518469));
#48033=CARTESIAN_POINT('Ctrl Pts',(15.0654212846825,0.29236188773074,27.3260064557296));
#48034=CARTESIAN_POINT('Ctrl Pts',(15.0972488933773,-0.139390968065011,
27.3650620187745));
#48035=CARTESIAN_POINT('Ctrl Pts',(15.1290765020721,-0.537023149086413,
27.1923642651449));
#48036=CARTESIAN_POINT('Ctrl Pts',(15.1609041107669,-0.803200670809313,
26.8501868368683));
#48037=CARTESIAN_POINT('Ctrl Pts',(15.1927317194618,-0.872767542303841,
26.4222892838454));
#48038=CARTESIAN_POINT('Ctrl Pts',(15.2245593281565,-0.728694908470672,
26.0134140685621));
#48039=CARTESIAN_POINT('Ctrl Pts',(15.2563869368514,-0.406249440824799,
25.7236472901227));
#48040=CARTESIAN_POINT('Ctrl Pts',(15.2882145455462,0.015639378424601,25.6239192114041));
#48041=CARTESIAN_POINT('Ctrl Pts',(15.320042154241,0.433699928509178,25.7386416675996));
#48042=CARTESIAN_POINT('Ctrl Pts',(15.3518697629358,0.745597687591262,26.0397324402448));
#48043=CARTESIAN_POINT('Ctrl Pts',(15.3836973716307,0.874985083455662,26.4534893341863));
#48044=CARTESIAN_POINT('Ctrl Pts',(15.4155249803254,0.790190155461937,26.8786312936292));
#48045=CARTESIAN_POINT('Ctrl Pts',(15.4473525890203,0.511969342859715,27.2110903812289));
#48046=CARTESIAN_POINT('Ctrl Pts',(15.4791801977151,0.108426641151977,27.3694859411127));
#48047=CARTESIAN_POINT('Ctrl Pts',(15.5110078064099,-0.321657164409033,
27.3150452790421));
#48048=CARTESIAN_POINT('Ctrl Pts',(15.5428354151047,-0.673004451758036,
27.061094596497));
#48049=CARTESIAN_POINT('Ctrl Pts',(15.5746630237996,-0.85961103647116,26.6697969501533));
#48050=CARTESIAN_POINT('Ctrl Pts',(15.6064906324944,-0.835798617607276,
26.2369357319776));
#48051=CARTESIAN_POINT('Ctrl Pts',(15.6383182411892,-0.607396093630348,
25.8684684301265));
#48052=CARTESIAN_POINT('Ctrl Pts',(15.670145849884,-0.230312741493113,25.6545899341678));
#48053=CARTESIAN_POINT('Ctrl Pts',(15.7019734585788,0.203147478227175,25.6476542717921));
#48054=CARTESIAN_POINT('Ctrl Pts',(15.7338010672736,0.586880451397411,25.8493591819813));
#48055=CARTESIAN_POINT('Ctrl Pts',(15.7656286759684,0.826954496793968,26.2103305357195));
#48056=CARTESIAN_POINT('Ctrl Pts',(15.7974562846633,0.864603336095876,26.6422083313882));
#48057=CARTESIAN_POINT('Ctrl Pts',(15.8292838933581,0.690611136890996,27.0392758068989));
#48058=CARTESIAN_POINT('Ctrl Pts',(15.8611115020529,0.347568400735895,27.304337208585));
#48059=CARTESIAN_POINT('Ctrl Pts',(15.8929391107477,-0.0805535089695269,
27.372509753812));
#48060=CARTESIAN_POINT('Ctrl Pts',(15.9247667194425,-0.488957210819473,
27.2271058962022));
#48061=CARTESIAN_POINT('Ctrl Pts',(15.9565943281374,-0.777672024640725,
26.9037181695138));
#48062=CARTESIAN_POINT('Ctrl Pts',(15.9884219368322,-0.876025191633466,
26.4815067058666));
#48063=CARTESIAN_POINT('Ctrl Pts',(16.020249545527,-0.759941432957373,26.0638221042063));
#48064=CARTESIAN_POINT('Ctrl Pts',(16.0520771542218,-0.457836192104619,
25.7529068602219));
#48065=CARTESIAN_POINT('Ctrl Pts',(16.0839047629166,-0.0436599897858236,
25.6248680421809));
#48066=CARTESIAN_POINT('Ctrl Pts',(16.1157323716114,0.381203478234709,25.7110475004881));
#48067=CARTESIAN_POINT('Ctrl Pts',(16.1475599803063,0.712754444848184,25.9903498850648));
#48068=CARTESIAN_POINT('Ctrl Pts',(16.1793875890011,0.869834547644324,26.3944064489244));
#48069=CARTESIAN_POINT('Ctrl Pts',(16.2112151976959,0.813993095194338,26.8243106215965));
#48070=CARTESIAN_POINT('Ctrl Pts',(16.2430428063907,0.558899180011339,27.1748287522675));
#48071=CARTESIAN_POINT('Ctrl Pts',(16.2748704150855,0.166995703796211,27.3601596207786));
#48072=CARTESIAN_POINT('Ctrl Pts',(16.3066980237803,-0.265785644041754,
27.334937201067));
#48073=CARTESIAN_POINT('Ctrl Pts',(16.3385256324752,-0.633506926325045,
27.1053355372044));
#48074=CARTESIAN_POINT('Ctrl Pts',(16.37035324117,-0.84615586711807,26.7275574363672));
#48075=CARTESIAN_POINT('Ctrl Pts',(16.4021808498648,-0.851679414127489,
26.2940769224788));
#48076=CARTESIAN_POINT('Ctrl Pts',(16.4340084585596,-0.648725491578761,
25.9110030773592));
#48077=CARTESIAN_POINT('Ctrl Pts',(16.4658360672544,-0.286973966694253,
25.6721062382503));
#48078=CARTESIAN_POINT('Ctrl Pts',(16.4976636759493,0.145024185516322,25.6358645222422));
#48079=CARTESIAN_POINT('Ctrl Pts',(16.5294912846441,0.541522741611643,25.8111493205188));
#48080=CARTESIAN_POINT('Ctrl Pts',(16.5613188933389,0.805465210279413,26.1550537239889));
#48081=CARTESIAN_POINT('Ctrl Pts',(16.5931465020337,0.872242705753262,26.583395446905));
#48082=CARTESIAN_POINT('Ctrl Pts',(16.6249741107285,0.725509167474942,26.9913233011108));
#48083=CARTESIAN_POINT('Ctrl Pts',(16.6568017194234,0.401182613717069,27.2789830863088));
#48084=CARTESIAN_POINT('Ctrl Pts',(16.6886293281181,-0.0213470135804936,
27.3759602977967));
#48085=CARTESIAN_POINT('Ctrl Pts',(16.720456936813,-0.438651234112523,27.2585164685856));
#48086=CARTESIAN_POINT('Ctrl Pts',(16.7522845455078,-0.748580663388893,
26.9553999656387));
#48087=CARTESIAN_POINT('Ctrl Pts',(16.7841121542026,-0.875269544789723,
26.5408088504112));
#48088=CARTESIAN_POINT('Ctrl Pts',(16.8159397628974,-0.787706470747481,
26.1162283827109));
#48089=CARTESIAN_POINT('Ctrl Pts',(16.8477673715922,-0.507325478323994,
25.7855890556777));
#48090=CARTESIAN_POINT('Ctrl Pts',(16.8795949802871,-0.10275934036483,25.629826077015));
#48091=CARTESIAN_POINT('Ctrl Pts',(16.9114225889819,0.326960636986347,25.6870677271803));
#48092=CARTESIAN_POINT('Ctrl Pts',(16.9432501976767,0.676645891169302,25.9433021678813));
#48093=CARTESIAN_POINT('Ctrl Pts',(16.9750778063715,0.8606990764792,26.3358073147138));
#48094=CARTESIAN_POINT('Ctrl Pts',(17.0069054150664,0.834066923902435,26.7685041995821));
#48095=CARTESIAN_POINT('Ctrl Pts',(17.0387330237611,0.60326855623544,27.1354755592871));
#48096=CARTESIAN_POINT('Ctrl Pts',(17.070560632456,0.224799716990748,27.3468926891914));
#48097=CARTESIAN_POINT('Ctrl Pts',(17.1023882411507,-0.208696492798159,
27.3510040602751));
#48098=CARTESIAN_POINT('Ctrl Pts',(17.1342158498456,-0.591107140557163,
27.1468032828924));
#48099=CARTESIAN_POINT('Ctrl Pts',(17.1660434585404,-0.82882424545982,26.7842754190553));
#48100=CARTESIAN_POINT('Ctrl Pts',(17.1978710672352,-0.863658439603519,
26.3521615079739));
#48101=CARTESIAN_POINT('Ctrl Pts',(17.22969867593,-0.687082928822622,25.9562360544967));
#48102=CARTESIAN_POINT('Ctrl Pts',(17.2615262846249,-0.342320457998925,
25.6934153665245));
#48103=CARTESIAN_POINT('Ctrl Pts',(17.2933538933197,0.086236438391831,25.6280335415497));
#48104=CARTESIAN_POINT('Ctrl Pts',(17.3251815020145,0.493684293154122,25.7760953693158));
#48105=CARTESIAN_POINT('Ctrl Pts',(17.3570091107093,0.780285662025571,26.1013569946918));
#48106=CARTESIAN_POINT('Ctrl Pts',(17.3888367194041,0.875886521181471,26.5242008934958));
#48107=CARTESIAN_POINT('Ctrl Pts',(17.4206643280989,0.757082673810857,26.9411191864539));
#48108=CARTESIAN_POINT('Ctrl Pts',(17.4524919367938,0.452960380137535,27.2500616224666));
#48109=CARTESIAN_POINT('Ctrl Pts',(17.4843195454886,0.0379544948769752,
27.375395237509));
#48110=CARTESIAN_POINT('Ctrl Pts',(17.5161471541834,-0.386330428534896,
27.2864570019139));
#48111=CARTESIAN_POINT('Ctrl Pts',(17.5479747628782,-0.716069784581872,
27.0049861686412));
#48112=CARTESIAN_POINT('Ctrl Pts',(17.579802371573,-0.870485327848165,26.5999415787028));
#48113=CARTESIAN_POINT('Ctrl Pts',(17.6116299802679,-0.811898199690783,
26.1703596993712));
#48114=CARTESIAN_POINT('Ctrl Pts',(17.6434575889627,-0.554423780325743,
25.8216066833014));
#48115=CARTESIAN_POINT('Ctrl Pts',(17.6752851976575,-0.161514030550117,
25.6386525392877));
#48116=CARTESIAN_POINT('Ctrl Pts',(17.7071128063523,0.271457872908683,25.6670350399784));
#48117=CARTESIAN_POINT('Ctrl Pts',(17.7389404150471,0.636989319376892,25.8983848159446));
#48118=CARTESIAN_POINT('Ctrl Pts',(17.7707680237419,0.848456858924584,26.2787473491137));
#48119=CARTESIAN_POINT('Ctrl Pts',(17.8025956324368,0.848820515726568,26.7100314241014));
#48120=CARTESIAN_POINT('Ctrl Pts',(17.8450324440298,0.579834016898176,27.2240442104363));
#48121=CARTESIAN_POINT('Ctrl Pts',(17.8980784585212,-0.170889696122602,
27.4791305910779));
#48122=CARTESIAN_POINT('Ctrl Pts',(17.9511244730126,-0.790819799983081,
26.9848211523576));
#48123=CARTESIAN_POINT('Ctrl Pts',(17.9935612846056,-0.869783785083159,
26.4100798452247));
#48124=CARTESIAN_POINT('Ctrl Pts',(18.0253888933005,-0.723346098358382,
26.0044173136901));
#48125=CARTESIAN_POINT('Ctrl Pts',(18.0572165019953,-0.395534844509592,
25.7181762286391));
#48126=CARTESIAN_POINT('Ctrl Pts',(18.0890441106901,0.0267543597305262,
25.6243264274723));
#48127=CARTESIAN_POINT('Ctrl Pts',(18.1208717193849,0.443742562875346,25.7442892299081));
#48128=CARTESIAN_POINT('Ctrl Pts',(18.1526993280798,0.75144783238784,26.0495231687072));
#48129=CARTESIAN_POINT('Ctrl Pts',(18.1845269367746,0.875561354462757,26.4648755209135));
#48130=CARTESIAN_POINT('Ctrl Pts',(18.2163545454694,0.785165778302637,26.8889058057357));
#48131=CARTESIAN_POINT('Ctrl Pts',(18.2481821541642,0.50267256024079,27.2176958019182));
#48132=CARTESIAN_POINT('Ctrl Pts',(18.280009762859,0.097081066669982,27.370827814419));
#48133=CARTESIAN_POINT('Ctrl Pts',(18.3118373715538,-0.332246728994801,
27.3107832488446));
#48134=CARTESIAN_POINT('Ctrl Pts',(18.3436649802486,-0.680260460945816,
27.052278234901));
#48135=CARTESIAN_POINT('Ctrl Pts',(18.3754925889435,-0.861749597906357,
26.6585810270827));
#48136=CARTESIAN_POINT('Ctrl Pts',(18.4073201976383,-0.832300343595772,
26.2260674913711));
#48137=CARTESIAN_POINT('Ctrl Pts',(18.4391478063331,-0.599115135331636,
25.8606073079395));
#48138=CARTESIAN_POINT('Ctrl Pts',(18.4709754150279,-0.219277294139984,
25.6516607023674));
#48139=CARTESIAN_POINT('Ctrl Pts',(18.5028030237227,0.214236722714413,25.6503736970824));
#48140=CARTESIAN_POINT('Ctrl Pts',(18.5346306324176,0.59530870133453,25.8570617315489));
#48141=CARTESIAN_POINT('Ctrl Pts',(18.5664582411124,0.830658822419003,26.2211306753223));
#48142=CARTESIAN_POINT('Ctrl Pts',(18.5982858498072,0.862676887449892,26.6534623989214));
#48143=CARTESIAN_POINT('Ctrl Pts',(18.630113458502,0.683525525611608,27.0482289663804));
#48144=CARTESIAN_POINT('Ctrl Pts',(18.6619410671968,0.33705804553252,27.308797881006));
#48145=CARTESIAN_POINT('Ctrl Pts',(18.6937686758916,-0.0919158281754816,
27.3713860322737));
#48146=CARTESIAN_POINT('Ctrl Pts',(18.7255962845865,-0.498390187518964,
27.2206728527908));
#48147=CARTESIAN_POINT('Ctrl Pts',(18.7574238932813,-0.782866613565596,
26.893550508522));
#48148=CARTESIAN_POINT('Ctrl Pts',(18.7892515019761,-0.875709842670763,
26.4700933085941));
#48149=CARTESIAN_POINT('Ctrl Pts',(18.8210791106709,-0.754193337422004,
26.053956786912));
#48150=CARTESIAN_POINT('Ctrl Pts',(18.8529067193657,-0.448062392210722,
25.7470044946958));
#48151=CARTESIAN_POINT('Ctrl Pts',(18.8847343280605,-0.0322529547931279,
25.6243734327709));
#48152=CARTESIAN_POINT('Ctrl Pts',(18.9165619367554,0.39145148883905,25.7160817197175));
#48153=CARTESIAN_POINT('Ctrl Pts',(18.9483895454502,0.719334882410106,25.9996806367208));
#48154=CARTESIAN_POINT('Ctrl Pts',(18.980217154145,0.87113662647824,26.4057497145772));
#48155=CARTESIAN_POINT('Ctrl Pts',(19.0120447628398,0.809698087295199,26.834889751618));
#48156=CARTESIAN_POINT('Ctrl Pts',(19.0438723715346,0.550058434458596,27.1820541452));
#48157=CARTESIAN_POINT('Ctrl Pts',(19.0756999802295,0.155773293405102,27.3622626162404));
#48158=CARTESIAN_POINT('Ctrl Pts',(19.1075275889243,-0.276642653087724,
27.3314030194782));
#48159=CARTESIAN_POINT('Ctrl Pts',(19.1393551976191,-0.641340912229586,
27.09702928957));
#48160=CARTESIAN_POINT('Ctrl Pts',(19.1711828063139,-0.849049195698639,
26.716512358973));
#48161=CARTESIAN_POINT('Ctrl Pts',(19.2030104150088,-0.84892384492235,26.2829966732363));
#48162=CARTESIAN_POINT('Ctrl Pts',(19.2348380237035,-0.64099554376236,25.902599923685));
#48163=CARTESIAN_POINT('Ctrl Pts',(19.2666656323984,-0.276161807593532,
25.6684371374749));
#48164=CARTESIAN_POINT('Ctrl Pts',(19.2984932410932,0.156271912654531,25.6378276114259));
#48165=CARTESIAN_POINT('Ctrl Pts',(19.330320849788,0.550452773466548,25.8182640668944));
#48166=CARTESIAN_POINT('Ctrl Pts',(19.3621484584828,0.809891618186575,26.1655785516815));
#48167=CARTESIAN_POINT('Ctrl Pts',(19.3939760671776,0.871081976005171,26.594754046791));
#48168=CARTESIAN_POINT('Ctrl Pts',(19.4258036758724,0.719045428109123,27.0007352699978));
#48169=CARTESIAN_POINT('Ctrl Pts',(19.4576312845673,0.39099808452758,27.2841445250718));
#48170=CARTESIAN_POINT('Ctrl Pts',(19.4894588932621,-0.0327593230900933,
27.3756077689554));
#48171=CARTESIAN_POINT('Ctrl Pts',(19.5212865019569,-0.448497773493383,
27.2527362655511));
#48172=CARTESIAN_POINT('Ctrl Pts',(19.5531141106517,-0.754451157627163,
26.9456069894642));
#48173=CARTESIAN_POINT('Ctrl Pts',(19.5849417193465,-0.875726990985035,
26.5294002647037));
#48174=CARTESIAN_POINT('Ctrl Pts',(19.6167693280414,-0.782638893413152,
26.1059968263815));
#48175=CARTESIAN_POINT('Ctrl Pts',(19.6485969367361,-0.497973339148,25.7790390497384));
#48176=CARTESIAN_POINT('Ctrl Pts',(19.680424545431,-0.0914118931530433,
25.6285609579009));
#48177=CARTESIAN_POINT('Ctrl Pts',(19.7122521541258,0.337525719103477,25.6913971758347));
#48178=CARTESIAN_POINT('Ctrl Pts',(19.7440797628206,0.683842445305621,25.9521664045508));
#48179=CARTESIAN_POINT('Ctrl Pts',(19.7759073715154,0.86276550176665,26.3470365165613));
#48180=CARTESIAN_POINT('Ctrl Pts',(19.8077349802103,0.830497392107225,26.7793496375646));
#48181=CARTESIAN_POINT('Ctrl Pts',(19.839562588905,0.594936832367246,27.1432824448073));
#48182=CARTESIAN_POINT('Ctrl Pts',(19.8713901975999,0.213745271922699,27.3497500203207));
#48183=CARTESIAN_POINT('Ctrl Pts',(19.9032178062947,-0.219767705103356,
27.3482124109549));
#48184=CARTESIAN_POINT('Ctrl Pts',(19.9350454149895,-0.599485070434967,
27.1390459988373));
#48185=CARTESIAN_POINT('Ctrl Pts',(19.9668730236843,-0.832458099283822,
26.7734513690606));
#48186=CARTESIAN_POINT('Ctrl Pts',(19.9987006323791,-0.861658728362201,
26.3409202271136));
#48187=CARTESIAN_POINT('Ctrl Pts',(20.030528241074,-0.679939111709783,25.9473292637821));
#48188=CARTESIAN_POINT('Ctrl Pts',(20.0623558497688,-0.33178129881649,25.6890232382737));
#48189=CARTESIAN_POINT('Ctrl Pts',(20.0941834584636,0.0975912581185316,
25.6292313254123));
#48190=CARTESIAN_POINT('Ctrl Pts',(20.1260110671584,0.503075039293507,25.7825896271002));
#48191=CARTESIAN_POINT('Ctrl Pts',(20.1578386758532,0.78541411431491,26.1115584891656));
#48192=CARTESIAN_POINT('Ctrl Pts',(20.189666284548,0.875496403048518,26.5356116070047));
#48193=CARTESIAN_POINT('Ctrl Pts',(20.2214938932429,0.751271205083277,26.9509475742446));
#48194=CARTESIAN_POINT('Ctrl Pts',(20.2533215019377,0.443146857755472,27.2558988032573));
#48195=CARTESIAN_POINT('Ctrl Pts',(20.2851491106325,0.0265472625644233,
27.3758181210472));
#48196=CARTESIAN_POINT('Ctrl Pts',(20.3169767193273,-0.396550676993438,
27.2813512007288));
#48197=CARTESIAN_POINT('Ctrl Pts',(20.3488043280222,-0.722579366878462,
26.9956220302467));
#48198=CARTESIAN_POINT('Ctrl Pts',(20.3806319367169,-0.871732209510478,
26.5885725307662));
#48199=CARTESIAN_POINT('Ctrl Pts',(20.4124595454118,-0.807498979687936,
26.1598418954261));
#48200=CARTESIAN_POINT('Ctrl Pts',(20.4442871541066,-0.545602942518351,
25.8143765119107));
#48201=CARTESIAN_POINT('Ctrl Pts',(20.4761147628014,-0.150152050138101,
25.6367407688628));
#48202=CARTESIAN_POINT('Ctrl Pts',(20.5079423714962,0.282053657425552,25.6704170489714));
#48203=CARTESIAN_POINT('Ctrl Pts',(20.539769980191,0.645217150507662,25.9071619386416));
#48204=CARTESIAN_POINT('Ctrl Pts',(20.5715975888859,0.850441826915244,26.2890240835133));
#48205=CARTESIAN_POINT('Ctrl Pts',(20.6034251975807,0.847491975277755,26.7225297511439));
#48206=CARTESIAN_POINT('Ctrl Pts',(20.6352528062755,0.637089671994789,27.1015637024804));
#48207=CARTESIAN_POINT('Ctrl Pts',(20.6670804149703,0.270738028507132,27.3333445015265));
#48208=CARTESIAN_POINT('Ctrl Pts',(20.6989080236651,-0.161885944873748,
27.3611359237407));
#48209=CARTESIAN_POINT('Ctrl Pts',(20.7307356323599,-0.554882833714983,
27.1781350744157));
#48210=CARTESIAN_POINT('Ctrl Pts',(20.7625632410548,-0.812053298722016,
26.8291376282637));
#48211=CARTESIAN_POINT('Ctrl Pts',(20.7943908497496,-0.870446132080706,
26.3995725662476));
#48212=CARTESIAN_POINT('Ctrl Pts',(20.8262184584444,-0.715767704125924,
25.9945905303274));
#48213=CARTESIAN_POINT('Ctrl Pts',(20.8580460671392,-0.385880814780212,
25.7133246317007));
#48214=CARTESIAN_POINT('Ctrl Pts',(20.8898736758341,0.0384635129888852,
25.6246242541211));
#48215=CARTESIAN_POINT('Ctrl Pts',(20.9217012845288,0.453392589285155,25.7502018282994));
#48216=CARTESIAN_POINT('Ctrl Pts',(20.9535288932237,0.757338426861943,26.0593179768783));
#48217=CARTESIAN_POINT('Ctrl Pts',(20.9853565019185,0.875899956432333,26.4763060213094));
#48218=CARTESIAN_POINT('Ctrl Pts',(21.0171841106133,0.780055215903818,26.8990939719485));
#48219=CARTESIAN_POINT('Ctrl Pts',(21.0490117193081,0.493265461524222,27.2241901150745));
#48220=CARTESIAN_POINT('Ctrl Pts',(21.080839328003,0.0857322283975826,27.3720161256069));
#48221=CARTESIAN_POINT('Ctrl Pts',(21.1126669366977,-0.342786880094173,
27.3063865655749));
#48222=CARTESIAN_POINT('Ctrl Pts',(21.1444945453926,-0.687397254648788,
27.0433664993406));
#48223=CARTESIAN_POINT('Ctrl Pts',(21.1763221540874,-0.863743799112817,
26.6473390233391));
#48224=CARTESIAN_POINT('Ctrl Pts',(21.2081497627822,-0.828659705946547,
26.2152453160263));
#48225=CARTESIAN_POINT('Ctrl Pts',(21.239977371477,-0.590732998816771,25.8528549912012));
#48226=CARTESIAN_POINT('Ctrl Pts',(21.2718049801718,-0.208204322055058,
25.6488753918597));
#48227=CARTESIAN_POINT('Ctrl Pts',(21.3036325888667,0.22528943557288,25.6532374544635));
#48228=CARTESIAN_POINT('Ctrl Pts',(21.3354601975615,0.603635950391702,25.8648734160034));
#48229=CARTESIAN_POINT('Ctrl Pts',(21.3672878062563,0.834222059846133,26.2319781852714));
#48230=CARTESIAN_POINT('Ctrl Pts',(21.3991154149511,0.860603980257829,26.6646903988359));
#48231=CARTESIAN_POINT('Ctrl Pts',(21.4309430236459,0.676323840368784,27.0570890424817));
#48232=CARTESIAN_POINT('Ctrl Pts',(21.4627706323408,0.326490464716284,27.313121217749));
#48233=CARTESIAN_POINT('Ctrl Pts',(21.4945982410355,-0.103262543593578,
27.3701143519073));
#48234=CARTESIAN_POINT('Ctrl Pts',(21.5264258497304,-0.507738536360471,
27.2141174392205));
#48235=CARTESIAN_POINT('Ctrl Pts',(21.5582534584252,-0.787928273639996,
26.8833160235407));
#48236=CARTESIAN_POINT('Ctrl Pts',(21.59008106712,-0.875245798726787,26.4586849892235));
#48237=CARTESIAN_POINT('Ctrl Pts',(21.6219086758148,-0.748317181035922,
26.0441672073328));
#48238=CARTESIAN_POINT('Ctrl Pts',(21.6537362845097,-0.438212511721132,
25.741229986837));
#48239=CARTESIAN_POINT('Ctrl Pts',(21.6855638932045,-0.0208404433628588,
25.6240275037281));
#48240=CARTESIAN_POINT('Ctrl Pts',(21.7173915018993,0.401633031492615,25.7212490473082));
#48241=CARTESIAN_POINT('Ctrl Pts',(21.7492191105941,0.725793177755637,26.0090963420102));
#48242=CARTESIAN_POINT('Ctrl Pts',(21.7810467192889,0.872290787375023,26.4171089838099));
#48243=CARTESIAN_POINT('Ctrl Pts',(21.8128743279837,0.805265593631672,26.8454120177663));
#48244=CARTESIAN_POINT('Ctrl Pts',(21.8447019366786,0.541124289650361,27.18916372616));
#48245=CARTESIAN_POINT('Ctrl Pts',(21.8765295453734,0.144524432895027,27.3642192005508));
#48246=CARTESIAN_POINT('Ctrl Pts',(21.9083571540682,-0.287452688544044,
27.3277276666593));
#48247=CARTESIAN_POINT('Ctrl Pts',(21.940184762763,-0.649065999221366,27.0886216670826));
#48248=CARTESIAN_POINT('Ctrl Pts',(21.9720123714578,-0.851798356749761,
26.7054305180414));
#48249=CARTESIAN_POINT('Ctrl Pts',(22.0038399801527,-0.846024129472541,
26.271953270897));
#48250=CARTESIAN_POINT('Ctrl Pts',(22.0356675888474,-0.633156755675803,
25.894298207823));
#48251=CARTESIAN_POINT('Ctrl Pts',(22.0674951975423,-0.265302756551086,
25.6649092350704));
#48252=CARTESIAN_POINT('Ctrl Pts',(22.0993228062371,0.167493105010496,25.639937096441));
#48253=CARTESIAN_POINT('Ctrl Pts',(22.1311504149319,0.559289339104509,25.8254945712091));
#48254=CARTESIAN_POINT('Ctrl Pts',(22.1629780236267,0.814180507473988,26.1761601637325));
#48255=CARTESIAN_POINT('Ctrl Pts',(22.1948056323215,0.869773337588301,26.6060965575542));
#48256=CARTESIAN_POINT('Ctrl Pts',(22.2266332410164,0.712459595697104,27.01006221464));
#48257=CARTESIAN_POINT('Ctrl Pts',(22.2584608497112,0.380747164334811,27.2891728170403));
#48258=CARTESIAN_POINT('Ctrl Pts',(22.290288458406,-0.0441660701058053,
27.3751065629715));
#48259=CARTESIAN_POINT('Ctrl Pts',(22.3221160671008,-0.458268158493986,
27.2468282488062));
#48260=CARTESIAN_POINT('Ctrl Pts',(22.3539436757956,-0.760193546967717,
26.9357383497616));
#48261=CARTESIAN_POINT('Ctrl Pts',(22.3857712844904,-0.876035739796036,
26.5179866868646));
#48262=CARTESIAN_POINT('Ctrl Pts',(22.4175988931853,-0.777438424934401,
26.09583217132));
#48263=CARTESIAN_POINT('Ctrl Pts',(22.4494265018801,-0.488536644708137,
25.7726114620908));
#48264=CARTESIAN_POINT('Ctrl Pts',(22.4812541105749,-0.080048924296243,
25.6274438080998));
#48265=CARTESIAN_POINT('Ctrl Pts',(22.5130817192697,0.348033489730768,25.6958639242453));
#48266=CARTESIAN_POINT('Ctrl Pts',(22.5449093279645,0.690922883876116,25.9611236627568));
#48267=CARTESIAN_POINT('Ctrl Pts',(22.5767369366594,0.864685430406076,26.358291691324));
#48268=CARTESIAN_POINT('Ctrl Pts',(22.6085645453542,0.826786843057951,26.790147642504));
#48269=CARTESIAN_POINT('Ctrl Pts',(22.640392154049,0.586504088562538,27.1509801013885));
#48270=CARTESIAN_POINT('Ctrl Pts',(22.6722197627438,0.202654533882945,27.3524630655935));
#48271=CARTESIAN_POINT('Ctrl Pts',(22.7040473714386,-0.230801602472313,
27.3452767349221));
#48272=CARTESIAN_POINT('Ctrl Pts',(22.7358749801335,-0.607761205912453,
27.1311802079376));
#48273=CARTESIAN_POINT('Ctrl Pts',(22.7677025888282,-0.835950607557777,
26.7625808828307));
#48274=CARTESIAN_POINT('Ctrl Pts',(22.7995301975231,-0.859512699386321,
26.3297059663465));
#48275=CARTESIAN_POINT('Ctrl Pts',(22.8313578062179,-0.672679858980042,
25.9385162997673));
#48276=CARTESIAN_POINT('Ctrl Pts',(22.8631854149127,-0.321185771047252,
25.6847688433449));
#48277=CARTESIAN_POINT('Ctrl Pts',(22.8950130236075,0.108929445558247,25.630576907257));
#48278=CARTESIAN_POINT('Ctrl Pts',(22.9268406323023,0.51238047985094,25.7892058088504));
#48279=CARTESIAN_POINT('Ctrl Pts',(22.9586682409972,0.790408985292522,26.1218257355752));
#48280=CARTESIAN_POINT('Ctrl Pts',(22.990495849692,0.874958040090555,26.5470166607199));
#48281=CARTESIAN_POINT('Ctrl Pts',(23.0223234583868,0.745331390812788,26.9606986609199));
#48282=CARTESIAN_POINT('Ctrl Pts',(23.0541510670816,0.433259563500411,27.2616090131687));
#48283=CARTESIAN_POINT('Ctrl Pts',(23.0859786757764,0.0151327394813605,
27.3760896863336));
#48284=CARTESIAN_POINT('Ctrl Pts',(23.1178062844713,-0.406698336609806,
27.2761176465609));
#48285=CARTESIAN_POINT('Ctrl Pts',(23.1496338931661,-0.728976178604333,
26.9861644467994));
#48286=CARTESIAN_POINT('Ctrl Pts',(23.1814615018609,-0.872812336365727,
26.577205982878));
#48287=CARTESIAN_POINT('Ctrl Pts',(23.2132891105557,-0.802998023931051,
26.1493487318329));
#48288=CARTESIAN_POINT('Ctrl Pts',(23.2451167192505,-0.536622665975705,
25.807325290872));
#48289=CARTESIAN_POINT('Ctrl Pts',(23.2769443279453,-0.138890680568273,
25.6348575162694));
#48290=CARTESIAN_POINT('Ctrl Pts',(23.3087719366402,0.292839517253094,25.6741627548728));
#48291=CARTESIAN_POINT('Ctrl Pts',(23.340599545335,0.652887294986739,25.9156197142705));
#48292=CARTESIAN_POINT('Ctrl Pts',(23.3724271540298,0.853118727617184,26.30012360096));
#48293=CARTESIAN_POINT('Ctrl Pts',(23.4042547627246,0.844520369817035,26.7335540264445));
#48294=CARTESIAN_POINT('Ctrl Pts',(23.4360823714194,0.62919696175823,27.1098141697423));
#48295=CARTESIAN_POINT('Ctrl Pts',(23.4679099801142,0.25985622245349,27.3368015786055));
#48296=CARTESIAN_POINT('Ctrl Pts',(23.4997375888091,-0.173093155040001,
27.3589533735789));
#48297=CARTESIAN_POINT('Ctrl Pts',(23.5315651975039,-0.56367210257829,27.1708471503102));
#48298=CARTESIAN_POINT('Ctrl Pts',(23.5633928061987,-0.816273154142162,
26.818528297222));
#48299=CARTESIAN_POINT('Ctrl Pts',(23.5952204148935,-0.869063621088188,
26.3882388224586));
#48300=CARTESIAN_POINT('Ctrl Pts',(23.6270480235883,-0.709121243252345,
25.9853066926095));
#48301=CARTESIAN_POINT('Ctrl Pts',(23.6588756322832,-0.375597351115582,
25.7083632347223));
#48302=CARTESIAN_POINT('Ctrl Pts',(23.6907032409779,0.0498667523664727,
25.6251997683398));
#48303=CARTESIAN_POINT('Ctrl Pts',(23.7225308496728,0.463124274151249,25.7561733770587));
#48304=CARTESIAN_POINT('Ctrl Pts',(23.7543584583676,0.763016396744221,26.0692238207563));
#48305=CARTESIAN_POINT('Ctrl Pts',(23.7861860670624,0.876134335312124,26.487721368499));
#48306=CARTESIAN_POINT('Ctrl Pts',(23.8180136757572,0.774788631588053,26.909224528427));
#48307=CARTESIAN_POINT('Ctrl Pts',(23.8498412844521,0.483787089438719,27.2305560829921));
#48308=CARTESIAN_POINT('Ctrl Pts',(23.8816688931468,0.0743622221061536,
27.3730592180533));
#48309=CARTESIAN_POINT('Ctrl Pts',(23.9134965018417,-0.353265325293876,
27.3018514502384));
#48310=CARTESIAN_POINT('Ctrl Pts',(23.9453241105365,-0.694419183324126,
27.0343632997651));
#48311=CARTESIAN_POINT('Ctrl Pts',(23.9771517192313,-0.865590355674041,
26.6360715784741));
#48312=CARTESIAN_POINT('Ctrl Pts',(24.0089793279262,-0.824878882944739,
26.2044717157763));
#48313=CARTESIAN_POINT('Ctrl Pts',(24.0408069366209,-0.582250281122388,
25.8452124402241));
#48314=CARTESIAN_POINT('Ctrl Pts',(24.0726345453158,-0.197096142995666,
25.6462346641374));
#48315=CARTESIAN_POINT('Ctrl Pts',(24.1044621540105,0.236303971809375,25.6562449578157));
#48316=CARTESIAN_POINT('Ctrl Pts',(24.1362897627054,0.611860661879505,25.872792961815));
#48317=CARTESIAN_POINT('Ctrl Pts',(24.1681173714002,0.837643669041631,26.2428711956648));
#48318=CARTESIAN_POINT('Ctrl Pts',(24.1999449800951,0.858384932072728,26.675890439464));
#48319=CARTESIAN_POINT('Ctrl Pts',(24.2317725887899,0.669007322231117,27.0658545229169));
#48320=CARTESIAN_POINT('Ctrl Pts',(24.2636001974847,0.315867442994404,27.317306488877));
#48321=CARTESIAN_POINT('Ctrl Pts',(24.2954278061795,-0.114591723451727,
27.3686949264389));
#48322=CARTESIAN_POINT('Ctrl Pts',(24.3272554148743,-0.517000672713736,
27.2074407697595));
#48323=CARTESIAN_POINT('Ctrl Pts',(24.3590830235691,-0.792856143965913,
26.873016451755));
#48324=CARTESIAN_POINT('Ctrl Pts',(24.390910632264,-0.874633139355223,26.447283685201));
#48325=CARTESIAN_POINT('Ctrl Pts',(24.4227382409587,-0.742313961161101,
26.0344550275541));
#48326=CARTESIAN_POINT('Ctrl Pts',(24.4545658496536,-0.428288223346675,
25.7355843172417));
#48327=CARTESIAN_POINT('Ctrl Pts',(24.4863934583483,-0.00942439321280878,
25.6238303137423));
#48328=CARTESIAN_POINT('Ctrl Pts',(24.5182210670433,0.411746377322031,25.7265486058798));
#48329=CARTESIAN_POINT('Ctrl Pts',(24.550048675738,0.732128234305675,26.0185954021441));
#48330=CARTESIAN_POINT('Ctrl Pts',(24.5818762844329,0.873296834342774,26.4284823278396));
#48331=CARTESIAN_POINT('Ctrl Pts',(24.6137038931277,0.800696366844726,26.8558756333693));
#48332=CARTESIAN_POINT('Ctrl Pts',(24.6455315018225,0.532098262588963,27.1961562879513));
#48333=CARTESIAN_POINT('Ctrl Pts',(24.6773591105173,0.133251032311443,27.3660290414832));
#48334=CARTESIAN_POINT('Ctrl Pts',(24.7091867192121,-0.298213914881034,
27.3239117666811));
#48335=CARTESIAN_POINT('Ctrl Pts',(24.741014327907,-0.656680875589221,27.0801140973462));
#48336=CARTESIAN_POINT('Ctrl Pts',(24.7728419366017,-0.854402883467569,
26.6943137952556));
#48337=CARTESIAN_POINT('Ctrl Pts',(24.8046695452966,-0.842980760146056,
26.2609485906171));
#48338=CARTESIAN_POINT('Ctrl Pts',(24.8364971539914,-0.625210458335947,
25.8860993393946));
#48339=CARTESIAN_POINT('Ctrl Pts',(24.8683247626862,-0.254398657420573,
25.6615231300704));
#48340=CARTESIAN_POINT('Ctrl Pts',(24.900152371381,0.178685857239278,25.6421926190997));
#48341=CARTESIAN_POINT('Ctrl Pts',(24.9319799800758,0.568030938087369,25.8328396057319));
#48342=CARTESIAN_POINT('Ctrl Pts',(24.9638075887707,0.818331149893379,26.1867967633971));
#48343=CARTESIAN_POINT('Ctrl Pts',(24.9956351974655,0.868317012707937,26.6174210532499));
#48344=CARTESIAN_POINT('Ctrl Pts',(25.0274628061603,0.705752788505203,27.0193025513335));
#48345=CARTESIAN_POINT('Ctrl Pts',(25.0592904148551,0.370431593732857,27.2940671084165));
#48346=CARTESIAN_POINT('Ctrl Pts',(25.0911180235499,-0.0555653177760932,
27.3744567649488));
#48347=CARTESIAN_POINT('Ctrl Pts',(25.1229456322447,-0.467960730114108,
27.2407934215255));
#48348=CARTESIAN_POINT('Ctrl Pts',(25.1547732409396,-0.765806856361044,
26.9257957222128));
#48349=CARTESIAN_POINT('Ctrl Pts',(25.1866008496344,-0.876195738795198,
26.5065700549077));
#48350=CARTESIAN_POINT('Ctrl Pts',(25.2184284583292,-0.772105948348922,
26.0857361434682));
#48351=CARTESIAN_POINT('Ctrl Pts',(25.250256067024,-0.479016997335324,25.7663073841395));
#48352=CARTESIAN_POINT('Ctrl Pts',(25.2820836757188,-0.0686723632286731,
25.6264748172875));
#48353=CARTESIAN_POINT('Ctrl Pts',(25.3139112844136,0.358482164691299,25.7004672139914));
#48354=CARTESIAN_POINT('Ctrl Pts',(25.3457388931085,0.697886004574409,25.9701724215148));
#48355=CARTESIAN_POINT('Ctrl Pts',(25.3775665018033,0.866458536502466,26.3695709279865));
#48356=CARTESIAN_POINT('Ctrl Pts',(25.4093941104981,0.822935906600167,26.8008963807238));
#48357=CARTESIAN_POINT('Ctrl Pts',(25.4412217191929,0.577971757070994,27.1585672223336));
#48358=CARTESIAN_POINT('Ctrl Pts',(25.4730493278877,0.191529385348056,27.3550313636665));
#48359=CARTESIAN_POINT('Ctrl Pts',(25.5048769365825,-0.241796310008061,
27.3421975319184));
#48360=CARTESIAN_POINT('Ctrl Pts',(25.5367045452774,-0.615934144269444,
27.1232072434019));
#48361=CARTESIAN_POINT('Ctrl Pts',(25.5685321539722,-0.839301172428612,
26.7516658106803));
#48362=CARTESIAN_POINT('Ctrl Pts',(25.600359762667,-0.857220726187857,26.3185206213073));
#48363=CARTESIAN_POINT('Ctrl Pts',(25.6321873713618,-0.665306386027568,
25.9297986749954));
#48364=CARTESIAN_POINT('Ctrl Pts',(25.6640149800566,-0.310535706310569,
25.6806528737063));
#48365=CARTESIAN_POINT('Ctrl Pts',(25.6958425887515,0.120249136888709,25.6320701160504));
#48366=CARTESIAN_POINT('Ctrl Pts',(25.7276701974463,0.521598918860212,25.7959426826794));
#48367=CARTESIAN_POINT('Ctrl Pts',(25.7594978061411,0.795269645703851,26.1321571953627));
#48368=CARTESIAN_POINT('Ctrl Pts',(25.7913254148359,0.874271110452719,26.5584137313573));
#48369=CARTESIAN_POINT('Ctrl Pts',(25.8231530235307,0.739265019907162,26.9703715209621));
#48370=CARTESIAN_POINT('Ctrl Pts',(25.8549806322256,0.423298702792696,27.2671899038389));
#48371=CARTESIAN_POINT('Ctrl Pts',(25.8868082409203,0.00371564593592677,
27.3762124906646));
#48372=CARTESIAN_POINT('Ctrl Pts',(25.9186358496152,-0.416776937561546,
27.2707523122981));
#48373=CARTESIAN_POINT('Ctrl Pts',(25.95046345831,-0.735249214411046,26.9766243061436));
#48374=CARTESIAN_POINT('Ctrl Pts',(25.9822910670048,-0.873744254401199,
26.5658263388602));
#48375=CARTESIAN_POINT('Ctrl Pts',(26.0141186756997,-0.798360732045715,
26.1389150831885));
#48376=CARTESIAN_POINT('Ctrl Pts',(26.0459462843944,-0.527551248954989,
25.8003917327718));
#48377=CARTESIAN_POINT('Ctrl Pts',(26.0777738930893,-0.127605770195691,
25.6331210739316));
#48378=CARTESIAN_POINT('Ctrl Pts',(26.1096015017841,0.303575733848321,25.6780488566812));
#48379=CARTESIAN_POINT('Ctrl Pts',(26.1414291104789,0.6604464278685,25.9241763964648));
#48380=CARTESIAN_POINT('Ctrl Pts',(26.1732567191737,0.855651057026928,26.3112576623533));
#48381=CARTESIAN_POINT('Ctrl Pts',(26.2050843278685,0.841404823443538,26.7445375018455));
#48382=CARTESIAN_POINT('Ctrl Pts',(26.2369119365634,0.621198438810439,27.117963249074));
#48383=CARTESIAN_POINT('Ctrl Pts',(26.2687395452581,0.248928358756431,27.3401124925143));
#48384=CARTESIAN_POINT('Ctrl Pts',(26.300567153953,-0.184267317446832,27.3566326768286));
#48385=CARTESIAN_POINT('Ctrl Pts',(26.3323947626478,-0.572372600161979,
27.1634307098942));
#48386=CARTESIAN_POINT('Ctrl Pts',(26.3642223713426,-0.820341019289417,
26.8078929774887));
#48387=CARTESIAN_POINT('Ctrl Pts',(26.3960499800375,-0.867561115381817,
26.3768668161923));
#48388=CARTESIAN_POINT('Ctrl Pts',(26.417268385834,-0.757378500801713,26.1097887611524));
#48389=CARTESIAN_POINT('Ctrl Pts',(26.4278775887323,-0.673641898681181,
25.9975270329735));
#48390=CARTESIAN_POINT('Ctrl Pts',(9.57962256921138,-0.830248497164267,
26.8880319004024));
#48391=CARTESIAN_POINT('Ctrl Pts',(9.59023177210965,-0.894913613471617,
26.7496718439806));
#48392=CARTESIAN_POINT('Ctrl Pts',(9.6114501779062,-0.953673908640778,26.4401420407412));
#48393=CARTESIAN_POINT('Ctrl Pts',(9.643277786601,-0.80817341482536,25.9902417865545));
#48394=CARTESIAN_POINT('Ctrl Pts',(9.67510539529583,-0.464933699438219,
25.6652387735807));
#48395=CARTESIAN_POINT('Ctrl Pts',(9.70693300399065,-0.00784090380745088,
25.5445127616791));
#48396=CARTESIAN_POINT('Ctrl Pts',(9.73876061268547,0.45114778502721,25.6577057284115));
#48397=CARTESIAN_POINT('Ctrl Pts',(9.77058822138028,0.799715104863132,25.9770624440697));
#48398=CARTESIAN_POINT('Ctrl Pts',(9.8024158300751,0.952518433985614,26.4244345660751));
#48399=CARTESIAN_POINT('Ctrl Pts',(9.83424343876991,0.87216398679464,26.8902993016558));
#48400=CARTESIAN_POINT('Ctrl Pts',(9.86607104746474,0.578315937843598,27.2606274566905));
#48401=CARTESIAN_POINT('Ctrl Pts',(9.89789865615955,0.142906389714678,27.4447649136056));
#48402=CARTESIAN_POINT('Ctrl Pts',(9.92972626485437,-0.327484867340805,
27.3976397450008));
#48403=CARTESIAN_POINT('Ctrl Pts',(9.96155387354919,-0.717712805021489,
27.1307863931583));
#48404=CARTESIAN_POINT('Ctrl Pts',(9.993381482244,-0.932256296314281,26.7095268341116));
#48405=CARTESIAN_POINT('Ctrl Pts',(10.0252090909388,-0.918598312263225,
26.2369783630933));
#48406=CARTESIAN_POINT('Ctrl Pts',(10.0570366996336,-0.680082225526843,
25.8288134266618));
#48407=CARTESIAN_POINT('Ctrl Pts',(10.0888643083285,-0.275092889112725,
25.5849441769394));
#48408=CARTESIAN_POINT('Ctrl Pts',(10.1206919170233,0.197234765899907,25.5650659409174));
#48409=CARTESIAN_POINT('Ctrl Pts',(10.1525195257181,0.621282517590593,25.7740445691304));
#48410=CARTESIAN_POINT('Ctrl Pts',(10.1843471344129,0.893250263923072,26.1607254551713));
#48411=CARTESIAN_POINT('Ctrl Pts',(10.2161747431077,0.946564664668695,26.630455309537));
#48412=CARTESIAN_POINT('Ctrl Pts',(10.2480023518025,0.768175206483761,27.0682517962964));
#48413=CARTESIAN_POINT('Ctrl Pts',(10.2798299604974,0.401748770810461,27.366949350837));
#48414=CARTESIAN_POINT('Ctrl Pts',(10.3116575691922,-0.0630193248360654,
27.453431600397));
#48415=CARTESIAN_POINT('Ctrl Pts',(10.343485177887,-0.512361299725991,27.3065290759445));
#48416=CARTESIAN_POINT('Ctrl Pts',(10.3753127865818,-0.836285440822322,
26.9622011611285));
#48417=CARTESIAN_POINT('Ctrl Pts',(10.4071403952766,-0.95550031024828,26.5047338103433));
#48418=CARTESIAN_POINT('Ctrl Pts',(10.4389680039715,-0.840824018843678,
26.0461076986875));
#48419=CARTESIAN_POINT('Ctrl Pts',(10.4707956126662,-0.520327484641828,
25.6985871472319));
#48420=CARTESIAN_POINT('Ctrl Pts',(10.5026232213611,-0.0724631221990005,
25.5472396168115));
#48421=CARTESIAN_POINT('Ctrl Pts',(10.5344508300559,0.393139051096402,25.6291125570096));
#48422=CARTESIAN_POINT('Ctrl Pts',(10.5662784387507,0.762507086054255,25.9241647843606));
#48423=CARTESIAN_POINT('Ctrl Pts',(10.5981060474455,0.94522560808136,26.3601722428075));
#48424=CARTESIAN_POINT('Ctrl Pts',(10.6299336561403,0.896568051661617,26.8304072950067));
#48425=CARTESIAN_POINT('Ctrl Pts',(10.6617612648352,0.628445006706643,27.2197639372736));
#48426=CARTESIAN_POINT('Ctrl Pts',(10.69358887353,0.206488697049629,27.432933904328));
#48427=CARTESIAN_POINT('Ctrl Pts',(10.7254164822248,-0.266012735970864,
27.4177366049992));
#48428=CARTESIAN_POINT('Ctrl Pts',(10.7572440909196,-0.673398514972374,
27.1778920945748));
#48429=CARTESIAN_POINT('Ctrl Pts',(10.7890716996145,-0.915947130979303,
26.772110464894));
#48430=CARTESIAN_POINT('Ctrl Pts',(10.8208993083092,-0.934286570448576,
26.2997205548902));
#48431=CARTESIAN_POINT('Ctrl Pts',(10.8527269170041,-0.723927632549161,
25.8763558428994));
#48432=CARTESIAN_POINT('Ctrl Pts',(10.8845545256989,-0.336362813571031,
25.6056492245765));
#48433=CARTESIAN_POINT('Ctrl Pts',(10.9163821343937,0.133538230826593,25.5538653411054));
#48434=CARTESIAN_POINT('Ctrl Pts',(10.9482097430885,0.570751256716081,25.7336800571491));
#48435=CARTESIAN_POINT('Ctrl Pts',(10.9800373517833,0.868253523165414,26.1010776123544));
#48436=CARTESIAN_POINT('Ctrl Pts',(11.0118649604781,0.953221243819833,26.5661249739856));
#48437=CARTESIAN_POINT('Ctrl Pts',(11.043692569173,0.804855682555953,27.0149860018597));
#48438=CARTESIAN_POINT('Ctrl Pts',(11.0755201778678,0.459474350715236,27.3377867108572));
#48439=CARTESIAN_POINT('Ctrl Pts',(11.1073477865626,0.00162106243758639,
27.4555106613799));
#48440=CARTESIAN_POINT('Ctrl Pts',(11.1391753952574,-0.456629035941818,
27.3393409172612));
#48441=CARTESIAN_POINT('Ctrl Pts',(11.1710030039522,-0.803103665335106,
27.0177139698514));
#48442=CARTESIAN_POINT('Ctrl Pts',(11.2028306126471,-0.952991389885271,
26.5693589407255));
#48443=CARTESIAN_POINT('Ctrl Pts',(11.2346582213419,-0.869602097076131,
26.1040259546197));
#48444=CARTESIAN_POINT('Ctrl Pts',(11.2664858300367,-0.573348149194159,
25.7356210680104));
#48445=CARTESIAN_POINT('Ctrl Pts',(11.2983134387315,-0.136747764217315,
25.5543238922149));
#48446=CARTESIAN_POINT('Ctrl Pts',(11.3301410474263,0.333326281598174,25.6045130699726));
#48447=CARTESIAN_POINT('Ctrl Pts',(11.3619686561212,0.721807396350512,25.8739030950183));
#48448=CARTESIAN_POINT('Ctrl Pts',(11.393796264816,0.933601629861665,26.2965516070998));
#48449=CARTESIAN_POINT('Ctrl Pts',(11.4256238735108,0.916865148481333,26.7690010248202));
#48450=CARTESIAN_POINT('Ctrl Pts',(11.4574514822056,0.675694774593156,27.1756033033086));
#48451=CARTESIAN_POINT('Ctrl Pts',(11.4892790909004,0.269125150160512,27.4168287219569));
#48452=CARTESIAN_POINT('Ctrl Pts',(11.5211066995952,-0.203321997397894,
27.4336291647267));
#48453=CARTESIAN_POINT('Ctrl Pts',(11.5529343082901,-0.625999178910517,
27.2218921525113));
#48454=CARTESIAN_POINT('Ctrl Pts',(11.5847619169849,-0.895441795163115,
26.8334475121051));
#48455=CARTESIAN_POINT('Ctrl Pts',(11.6165895256797,-0.945694612419042,
26.3633802653508));
#48456=CARTESIAN_POINT('Ctrl Pts',(11.6484171343745,-0.764456546484064,
25.926755339849));
#48457=CARTESIAN_POINT('Ctrl Pts',(11.6802447430693,-0.396091770950939,
25.630451518983));
#48458=CARTESIAN_POINT('Ctrl Pts',(11.7120723517642,0.0692299214113307,
25.546999228838));
#48459=CARTESIAN_POINT('Ctrl Pts',(11.743899960459,0.517605238653885,25.6968262524384));
#48460=CARTESIAN_POINT('Ctrl Pts',(11.7757275691538,0.839279089834648,26.0432573358878));
#48461=CARTESIAN_POINT('Ctrl Pts',(11.8075551778486,0.955510872087357,26.501491702678));
#48462=CARTESIAN_POINT('Ctrl Pts',(11.8393827865434,0.837848908120856,26.9593609245623));
#48463=CARTESIAN_POINT('Ctrl Pts',(11.8712103952382,0.515094960786372,27.3047859549138));
#48464=CARTESIAN_POINT('Ctrl Pts',(11.903038003933,0.0662540231764387,27.4532122828976));
#48465=CARTESIAN_POINT('Ctrl Pts',(11.9348656126279,-0.398804837364059,
27.3683075224534));
#48466=CARTESIAN_POINT('Ctrl Pts',(11.9666932213227,-0.766242665903474,
27.0708549980539));
#48467=CARTESIAN_POINT('Ctrl Pts',(11.9985208300175,-0.946116571439429,
26.6336663199977));
#48468=CARTESIAN_POINT('Ctrl Pts',(12.0303484387123,-0.894396304979596,
26.1637582692573));
#48469=CARTESIAN_POINT('Ctrl Pts',(12.0621760474071,-0.623742158762532,
25.7761568048007));
#48470=CARTESIAN_POINT('Ctrl Pts',(12.094003656102,-0.200405929641351,25.5657405525131));
#48471=CARTESIAN_POINT('Ctrl Pts',(12.1258312647968,0.271986458878584,25.5840160383278));
#48472=CARTESIAN_POINT('Ctrl Pts',(12.1576588734916,0.677800921760648,25.8265097162434));
#48473=CARTESIAN_POINT('Ctrl Pts',(12.1894864821864,0.917700583029717,26.2338630206812));
#48474=CARTESIAN_POINT('Ctrl Pts',(12.2213140908812,0.932961850804134,26.7063623919181));
#48475=CARTESIAN_POINT('Ctrl Pts',(12.253141699576,0.719849011345744,27.1283475572632));
#48476=CARTESIAN_POINT('Ctrl Pts',(12.2849693082708,0.330528671905649,27.3965233119681));
#48477=CARTESIAN_POINT('Ctrl Pts',(12.3167969169657,-0.139699788585952,
27.4452445296975));
#48478=CARTESIAN_POINT('Ctrl Pts',(12.3486245256605,-0.575731979989561,
27.2625850372721));
#48479=CARTESIAN_POINT('Ctrl Pts',(12.3804521343553,-0.870834210728471,
26.8932569507065));
#48480=CARTESIAN_POINT('Ctrl Pts',(12.4122797430501,-0.952770184721209,
26.42766586587));
#48481=CARTESIAN_POINT('Ctrl Pts',(12.444107351745,-0.801483288833254,25.9797810176714));
#48482=CARTESIAN_POINT('Ctrl Pts',(12.4759349604397,-0.454006130297858,
25.659237438092));
#48483=CARTESIAN_POINT('Ctrl Pts',(12.5077625691346,0.00460445196288184,
25.5444990576268));
#48484=CARTESIAN_POINT('Ctrl Pts',(12.5395901778294,0.4620879381849,25.6636519927458));
#48485=CARTESIAN_POINT('Ctrl Pts',(12.5714177865242,0.806459703648916,25.9875295147577));
#48486=CARTESIAN_POINT('Ctrl Pts',(12.603245395219,0.95342305988236,26.4368515974978));
#48487=CARTESIAN_POINT('Ctrl Pts',(12.6350730039139,0.867003732860179,26.9016313970055));
#48488=CARTESIAN_POINT('Ctrl Pts',(12.6669006126086,0.568355788677721,27.2680982680169));
#48489=CARTESIAN_POINT('Ctrl Pts',(12.6987282213035,0.130583457235488,27.4465469943698));
#48490=CARTESIAN_POINT('Ctrl Pts',(12.7305558299983,-0.33915361149994,27.3932961880925));
#48491=CARTESIAN_POINT('Ctrl Pts',(12.7623834386931,-0.725871312214778,
27.1213807930388));
#48492=CARTESIAN_POINT('Ctrl Pts',(12.7942110473879,-0.934907350222748,
26.6973613395615));
#48493=CARTESIAN_POINT('Ctrl Pts',(12.8260386560827,-0.915093053923393,
26.2250309935371));
#48494=CARTESIAN_POINT('Ctrl Pts',(12.8578662647776,-0.671278645460207,
25.8200086529939));
#48495=CARTESIAN_POINT('Ctrl Pts',(12.8896938734724,-0.263145984081015,
25.5814372950549));
#48496=CARTESIAN_POINT('Ctrl Pts',(12.9215214821672,0.209400596403874,25.567715364237));
#48497=CARTESIAN_POINT('Ctrl Pts',(12.953349090862,0.630689267236257,25.7822017692645));
#48498=CARTESIAN_POINT('Ctrl Pts',(12.9851766995568,0.897595314360882,26.1723936760509));
#48499=CARTESIAN_POINT('Ctrl Pts',(13.0170043082516,0.944784415506595,26.6427783599496));
#48500=CARTESIAN_POINT('Ctrl Pts',(13.0488319169465,0.760705435076608,27.0782131898348));
#48501=CARTESIAN_POINT('Ctrl Pts',(13.0806595256413,0.39041795699687,27.3721106986549));
#48502=CARTESIAN_POINT('Ctrl Pts',(13.1124871343361,-0.075437579197961,
27.4525294869445));
#48503=CARTESIAN_POINT('Ctrl Pts',(13.1443147430309,-0.522827205145454,
27.2997843243111));
#48504=CARTESIAN_POINT('Ctrl Pts',(13.1761423517257,-0.842237111333554,
26.9512647783138));
#48505=CARTESIAN_POINT('Ctrl Pts',(13.2079699604206,-0.955480872342886,
26.4922828476173));
#48506=CARTESIAN_POINT('Ctrl Pts',(13.2397975691154,-0.83483823058961,26.035189952131));
#48507=CARTESIAN_POINT('Ctrl Pts',(13.2716251778102,-0.509840571071793,
25.6918751062223));
#48508=CARTESIAN_POINT('Ctrl Pts',(13.303452786505,-0.0600421116614344,
25.5463762813975));
#48509=CARTESIAN_POINT('Ctrl Pts',(13.3352803951998,0.404453694307345,25.6343092578668));
#48510=CARTESIAN_POINT('Ctrl Pts',(13.3671080038946,0.769945718637211,25.9341494524114));
#48511=CARTESIAN_POINT('Ctrl Pts',(13.3989356125895,0.946967372008249,26.3725007913522));
#48512=CARTESIAN_POINT('Ctrl Pts',(13.4307632212843,0.892186591041172,26.8420618929672));
#48513=CARTESIAN_POINT('Ctrl Pts',(13.4625908299791,0.619012832870912,27.2278917258736));
#48514=CARTESIAN_POINT('Ctrl Pts',(13.4944184386739,0.194314654971488,27.4355453311932));
#48515=CARTESIAN_POINT('Ctrl Pts',(13.5262460473687,-0.277948635920619,
27.4141924346897));
#48516=CARTESIAN_POINT('Ctrl Pts',(13.5580736560635,-0.682174555798859,
27.1690598831754));
#48517=CARTESIAN_POINT('Ctrl Pts',(13.5899012647584,-0.91941507855371,26.7601521961893));
#48518=CARTESIAN_POINT('Ctrl Pts',(13.6217288734532,-0.931597526790183,
26.2875634213878));
#48519=CARTESIAN_POINT('Ctrl Pts',(13.653556482148,-0.7157398324446,25.8669757160217));
#48520=CARTESIAN_POINT('Ctrl Pts',(13.6853840908428,-0.32468049924893,25.6013422090353));
#48521=CARTESIAN_POINT('Ctrl Pts',(13.7172116995376,0.145855416068471,25.5556857252707));
#48522=CARTESIAN_POINT('Ctrl Pts',(13.7490393082324,0.580688263354752,25.7411822401551));
#48523=CARTESIAN_POINT('Ctrl Pts',(13.7808669169273,0.873377931249599,26.1124251800488));
#48524=CARTESIAN_POINT('Ctrl Pts',(13.8126945256221,0.952278680386351,26.5785402236797));
#48525=CARTESIAN_POINT('Ctrl Pts',(13.8445221343169,0.798076872025581,27.0254298794244));
#48526=CARTESIAN_POINT('Ctrl Pts',(13.8763497430117,0.448518637252629,27.3437027224627));
#48527=CARTESIAN_POINT('Ctrl Pts',(13.9081773517065,-0.0108297709036782,
27.4554506622093));
#48528=CARTESIAN_POINT('Ctrl Pts',(13.9400049604013,-0.467527224726181,
27.3333195941497));
#48529=CARTESIAN_POINT('Ctrl Pts',(13.9718325690962,-0.809781507628197,
27.0072052461849));
#48530=CARTESIAN_POINT('Ctrl Pts',(14.003660177791,-0.95381425692857,26.5569351836198));
#48531=CARTESIAN_POINT('Ctrl Pts',(14.0354877864858,-0.86436856420665,26.0927283006821));
#48532=CARTESIAN_POINT('Ctrl Pts',(14.0673153951806,-0.563339301373415,
25.7282150018417));
#48533=CARTESIAN_POINT('Ctrl Pts',(14.0991430038754,-0.12441360696645,25.5526223001065));
#48534=CARTESIAN_POINT('Ctrl Pts',(14.1309706125703,0.344966544280397,25.6089324743987));
#48535=CARTESIAN_POINT('Ctrl Pts',(14.1627982212651,0.729904414733746,25.8833616966112));
#48536=CARTESIAN_POINT('Ctrl Pts',(14.1946258299599,0.936173383627583,26.3087340917955));
#48537=CARTESIAN_POINT('Ctrl Pts',(14.2264534386547,0.913282113529031,26.7809253156302));
#48538=CARTESIAN_POINT('Ctrl Pts',(14.2582810473495,0.666834020448794,27.1843505249696));
#48539=CARTESIAN_POINT('Ctrl Pts',(14.2901086560443,0.257155647415318,27.4202576948097));
#48540=CARTESIAN_POINT('Ctrl Pts',(14.3219362647392,-0.21547030632334,27.4309005311777));
#48541=CARTESIAN_POINT('Ctrl Pts',(14.353763873434,-0.635352582708677,27.2136738383179));
#48542=CARTESIAN_POINT('Ctrl Pts',(14.3855914821288,-0.899710730503885,
26.8217512288558));
#48543=CARTESIAN_POINT('Ctrl Pts',(14.4174190908236,-0.943834112355007,
26.3510690757127));
#48544=CARTESIAN_POINT('Ctrl Pts',(14.4492466995184,-0.756922031610138,
25.9168428257175));
#48545=CARTESIAN_POINT('Ctrl Pts',(14.4810743082132,-0.384727569742386,
25.6253641049361));
#48546=CARTESIAN_POINT('Ctrl Pts',(14.5129019169081,0.0816420346481125,
25.5479822322916));
#48547=CARTESIAN_POINT('Ctrl Pts',(14.5447295256029,0.528026977544294,25.7036390499029));
#48548=CARTESIAN_POINT('Ctrl Pts',(14.5765571342977,0.845159379741648,26.0542322637418));
#48549=CARTESIAN_POINT('Ctrl Pts',(14.6083847429925,0.955410312293092,26.513942274493));
#48550=CARTESIAN_POINT('Ctrl Pts',(14.6402123516873,0.831792114051153,26.9702394399201));
#48551=CARTESIAN_POINT('Ctrl Pts',(14.6720399603822,0.504564538549048,27.3114295276195));
#48552=CARTESIAN_POINT('Ctrl Pts',(14.703867569077,0.0538276513498363,27.4539946728385));
#48553=CARTESIAN_POINT('Ctrl Pts',(14.7356951777718,-0.410085382131093,
27.3630372131122));
#48554=CARTESIAN_POINT('Ctrl Pts',(14.7675227864666,-0.773616087060543,
27.0608220766831));
#48555=CARTESIAN_POINT('Ctrl Pts',(14.7993503951614,-0.947777973671093,
26.6213266849376));
#48556=CARTESIAN_POINT('Ctrl Pts',(14.8311780038562,-0.889939003649095,
26.1521324653865));
#48557=CARTESIAN_POINT('Ctrl Pts',(14.8630056125511,-0.614257229792361,
25.7680906425644));
#48558=CARTESIAN_POINT('Ctrl Pts',(14.8948332212458,-0.188215131615601,
25.5632084991393));
#48559=CARTESIAN_POINT('Ctrl Pts',(14.9266608299407,0.283899014001654,25.5876378998978));
#48560=CARTESIAN_POINT('Ctrl Pts',(14.9584884386355,0.686519231425576,25.8353989190974));
#48561=CARTESIAN_POINT('Ctrl Pts',(14.9903160473303,0.921090544770697,26.2458436304397));
#48562=CARTESIAN_POINT('Ctrl Pts',(15.0221436560251,0.930193656322486,26.7185017473418));
#48563=CARTESIAN_POINT('Ctrl Pts',(15.05397126472,0.711600270280961,27.1376741387183));
#48564=CARTESIAN_POINT('Ctrl Pts',(15.0857988734148,0.318818543856639,27.4007541218042));
#48565=CARTESIAN_POINT('Ctrl Pts',(15.1176264821096,-0.15200485196688,27.4433439334795));
#48566=CARTESIAN_POINT('Ctrl Pts',(15.1494540908044,-0.585619896416687,
27.2550182704908));
#48567=CARTESIAN_POINT('Ctrl Pts',(15.1812816994992,-0.875884576747471,
26.8818762365871));
#48568=CARTESIAN_POINT('Ctrl Pts',(15.213109308194,-0.951746751679696,26.4152570208149));
#48569=CARTESIAN_POINT('Ctrl Pts',(15.2449369168889,-0.794636576735844,
25.9693815280566));
#48570=CARTESIAN_POINT('Ctrl Pts',(15.2767645255837,-0.443012104524464,
25.6533929322887));
#48571=CARTESIAN_POINT('Ctrl Pts',(15.3085921342785,0.0170546301190841,
25.5446401769775));
#48572=CARTESIAN_POINT('Ctrl Pts',(15.3404197429733,0.472946664667159,25.6697441934957));
#48573=CARTESIAN_POINT('Ctrl Pts',(15.3722473516681,0.813068936261896,25.9980815238109));
#48574=CARTESIAN_POINT('Ctrl Pts',(15.404074960363,0.95416496441753,26.4492804521697));
#48575=CARTESIAN_POINT('Ctrl Pts',(15.4359025690577,0.861696702978835,26.9128947128862));
#48576=CARTESIAN_POINT('Ctrl Pts',(15.4677301777526,0.558298900231862,27.2754389659116));
#48577=CARTESIAN_POINT('Ctrl Pts',(15.4995577864474,0.118238475321277,27.4481681890929));
#48578=CARTESIAN_POINT('Ctrl Pts',(15.5313853951422,-0.35076483317966,27.388801037161));
#48579=CARTESIAN_POINT('Ctrl Pts',(15.563213003837,-0.733906532701598,27.1118696373509));
#48580=CARTESIAN_POINT('Ctrl Pts',(15.5950406125319,-0.937399676332867,
26.6851623575813));
#48581=CARTESIAN_POINT('Ctrl Pts',(15.6268682212267,-0.911432404172941,
26.2131303005238));
#48582=CARTESIAN_POINT('Ctrl Pts',(15.6586958299215,-0.662361088233901,
25.8113193478487));
#48583=CARTESIAN_POINT('Ctrl Pts',(15.6905234386163,-0.251154394454069,
25.5780863804019));
#48584=CARTESIAN_POINT('Ctrl Pts',(15.7223510473111,0.22153086949624,25.5705230902737));
#48585=CARTESIAN_POINT('Ctrl Pts',(15.7541786560059,0.639988927369355,25.7904808496604));
#48586=CARTESIAN_POINT('Ctrl Pts',(15.7860062647008,0.901787953792385,26.1841175246251));
#48587=CARTESIAN_POINT('Ctrl Pts',(15.8178338733956,0.94284374330479,26.6550771664851));
#48588=CARTESIAN_POINT('Ctrl Pts',(15.8496614820904,0.753106496690714,27.0880764036214));
#48589=CARTESIAN_POINT('Ctrl Pts',(15.8814890907852,0.379020850745279,27.3771239630487));
#48590=CARTESIAN_POINT('Ctrl Pts',(15.91331669948,-0.0878430243817305,27.4514656351763));
#48591=CARTESIAN_POINT('Ctrl Pts',(15.9451443081748,-0.5332043351193,27.292903770242));
#48592=CARTESIAN_POINT('Ctrl Pts',(15.9769719168697,-0.848045771008207,
26.9402517712959));
#48593=CARTESIAN_POINT('Ctrl Pts',(16.0087995255645,-0.955299194933258,
26.4798331952482));
#48594=CARTESIAN_POINT('Ctrl Pts',(16.0406271342593,-0.828710687813575,
26.0243511297632));
#48595=CARTESIAN_POINT('Ctrl Pts',(16.0724547429541,-0.499267087186487,
25.685300283843));
#48596=CARTESIAN_POINT('Ctrl Pts',(16.1042823516489,-0.0476109060464227,
25.5456748701415));
#48597=CARTESIAN_POINT('Ctrl Pts',(16.1361099603437,0.415699661769282,25.6396529519671));
#48598=CARTESIAN_POINT('Ctrl Pts',(16.1679375690386,0.777253615365754,25.944230201203));
#48599=CARTESIAN_POINT('Ctrl Pts',(16.1997651777333,0.948548342017812,26.3848509891085));
#48600=CARTESIAN_POINT('Ctrl Pts',(16.2315927864282,0.887653638213781,26.8536584092311));
#48601=CARTESIAN_POINT('Ctrl Pts',(16.263420395123,0.609475551402932,27.2358959193365));
#48602=CARTESIAN_POINT('Ctrl Pts',(16.2952480038179,0.182107618499345,27.4379979035896));
#48603=CARTESIAN_POINT('Ctrl Pts',(16.3270756125126,-0.289837340527268,
27.4104930356077));
#48604=CARTESIAN_POINT('Ctrl Pts',(16.3589032212075,-0.690834764208691,
27.1601140662149));
#48605=CARTESIAN_POINT('Ctrl Pts',(16.3907308299023,-0.922726910556888,
26.7481497539554));
#48606=CARTESIAN_POINT('Ctrl Pts',(16.4225584385971,-0.928750298995543,
26.2754423593602));
#48607=CARTESIAN_POINT('Ctrl Pts',(16.4543860472919,-0.707430500579885,
25.8577030759039));
#48608=CARTESIAN_POINT('Ctrl Pts',(16.4862136559868,-0.312943054569711,
25.597187784503));
#48609=CARTESIAN_POINT('Ctrl Pts',(16.5180412646815,0.158147835236672,25.5576664528608));
#48610=CARTESIAN_POINT('Ctrl Pts',(16.5498688733764,0.59052666982678,25.7488132695013));
#48611=CARTESIAN_POINT('Ctrl Pts',(16.5816964820712,0.87835404081465,26.1238385574802));
#48612=CARTESIAN_POINT('Ctrl Pts',(16.613524090766,0.951174421181637,26.5909421373384));
#48613=CARTESIAN_POINT('Ctrl Pts',(16.6453516994608,0.79116254900519,27.0357845396294));
#48614=CARTESIAN_POINT('Ctrl Pts',(16.6771793081556,0.437486765866275,27.3494754743637));
#48615=CARTESIAN_POINT('Ctrl Pts',(16.7090069168505,-0.0232787653625354,
27.4552284286692));
#48616=CARTESIAN_POINT('Ctrl Pts',(16.7408345255453,-0.478346027952504,
27.3271567743758));
#48617=CARTESIAN_POINT('Ctrl Pts',(16.7726621342401,-0.816321849996796,
26.9966103996805));
#48618=CARTESIAN_POINT('Ctrl Pts',(16.8044897429349,-0.954475167464214,
26.5445017589863));
#48619=CARTESIAN_POINT('Ctrl Pts',(16.8363173516297,-0.858988262592818,
26.081499800992));
#48620=CARTESIAN_POINT('Ctrl Pts',(16.8681449603245,-0.553234799228007,
25.7209399838263));
#48621=CARTESIAN_POINT('Ctrl Pts',(16.8999725690194,-0.112058324417954,
25.5510815716047));
#48622=CARTESIAN_POINT('Ctrl Pts',(16.9318001777142,0.356548232026913,25.6135031809852));
#48623=CARTESIAN_POINT('Ctrl Pts',(16.963627786409,0.737877496289409,25.8929250027018));
#48624=CARTESIAN_POINT('Ctrl Pts',(16.9954553951038,0.938586176166046,26.3209490531028));
#48625=CARTESIAN_POINT('Ctrl Pts',(17.0272830037986,0.909544004595047,26.7928019058661));
#48626=CARTESIAN_POINT('Ctrl Pts',(17.0591106124935,0.657860038277722,27.1929815443489));
#48627=CARTESIAN_POINT('Ctrl Pts',(17.0909382211882,0.245142480733944,27.4235304097486));
#48628=CARTESIAN_POINT('Ctrl Pts',(17.1227658298831,-0.227582030128332,
27.4280138304583));
#48629=CARTESIAN_POINT('Ctrl Pts',(17.1545934385779,-0.644598101614693,
27.2053343457797));
#48630=CARTESIAN_POINT('Ctrl Pts',(17.1864210472727,-0.903826901316126,
26.810000307704));
#48631=CARTESIAN_POINT('Ctrl Pts',(17.2182486559675,-0.941813340449867,
26.3387831836783));
#48632=CARTESIAN_POINT('Ctrl Pts',(17.2500762646624,-0.749259011071048,
25.9070293133871));
#48633=CARTESIAN_POINT('Ctrl Pts',(17.2819038733572,-0.37329800679106,25.6204252362105));
#48634=CARTESIAN_POINT('Ctrl Pts',(17.313731482052,0.0940402181997153,25.5491268245229));
#48635=CARTESIAN_POINT('Ctrl Pts',(17.3455590907468,0.538359184536647,25.710587186869));
#48636=CARTESIAN_POINT('Ctrl Pts',(17.3773866994416,0.8508959238502,26.0652826589078));
#48637=CARTESIAN_POINT('Ctrl Pts',(17.4092143081364,0.955147975798902,26.5263909009626));
#48638=CARTESIAN_POINT('Ctrl Pts',(17.4410419168313,0.82559323144673,26.9810373122984));
#48639=CARTESIAN_POINT('Ctrl Pts',(17.4728695255261,0.493950049170587,27.3179368252602));
#48640=CARTESIAN_POINT('Ctrl Pts',(17.5046971342209,0.0413891047270388,
27.454612234474));
#48641=CARTESIAN_POINT('Ctrl Pts',(17.5365247429157,-0.421290564338076,
27.357625725782));
#48642=CARTESIAN_POINT('Ctrl Pts',(17.5683523516105,-0.780868969591605,
27.0506837987796));
#48643=CARTESIAN_POINT('Ctrl Pts',(17.6001799603053,-0.949258013167391,
26.6089855755142));
#48644=CARTESIAN_POINT('Ctrl Pts',(17.6320075690002,-0.885369169676656,
26.1405296139703));
#48645=CARTESIAN_POINT('Ctrl Pts',(17.663835177695,-0.604595160111121,25.7602169486908));
#48646=CARTESIAN_POINT('Ctrl Pts',(17.6956627863898,-0.176129893099558,
25.5607067654733));
#48647=CARTESIAN_POINT('Ctrl Pts',(17.7274903950846,0.296022865466284,25.5916576791216));
#48648=CARTESIAN_POINT('Ctrl Pts',(17.7593180037794,0.69463228888109,25.8439429522386));
#48649=CARTESIAN_POINT('Ctrl Pts',(17.7911456124743,0.925236125635749,26.2587255694389));
#48650=CARTESIAN_POINT('Ctrl Pts',(17.822973221169,0.925632690772768,26.7290377631501));
#48651=CARTESIAN_POINT('Ctrl Pts',(17.8654100327622,0.632304841034162,27.2895650238507));
#48652=CARTESIAN_POINT('Ctrl Pts',(17.9184560472535,-0.186353989231682,
27.5677348942982));
#48653=CARTESIAN_POINT('Ctrl Pts',(17.9715020617449,-0.862383325817902,
27.0286939930005));
#48654=CARTESIAN_POINT('Ctrl Pts',(18.013938873338,-0.948492985808557,26.4019427154772));
#48655=CARTESIAN_POINT('Ctrl Pts',(18.0457664820328,-0.788803737631534,
25.9595706313286));
#48656=CARTESIAN_POINT('Ctrl Pts',(18.0775940907276,-0.431327914010642,
25.6474267789399));
#48657=CARTESIAN_POINT('Ctrl Pts',(18.1094216994224,0.0291754375966058,
25.5450842431823));
#48658=CARTESIAN_POINT('Ctrl Pts',(18.1412493081172,0.483898085490023,25.6759028197294));
#48659=CARTESIAN_POINT('Ctrl Pts',(18.1730769168121,0.819448477247464,26.0087582430504));
#48660=CARTESIAN_POINT('Ctrl Pts',(18.2049045255069,0.954793383821898,26.461697007216));
#48661=CARTESIAN_POINT('Ctrl Pts',(18.2367321342017,0.856217655685264,26.9240989947235));
#48662=CARTESIAN_POINT('Ctrl Pts',(18.2685597428965,0.548160825395486,27.2826421298468));
#48663=CARTESIAN_POINT('Ctrl Pts',(18.3003873515913,0.105866207637405,27.449631492319));
#48664=CARTESIAN_POINT('Ctrl Pts',(18.3322149602861,-0.362312677488355,
27.3841533237673));
#48665=CARTESIAN_POINT('Ctrl Pts',(18.364042568981,-0.741819158733036,27.1022554581978));
#48666=CARTESIAN_POINT('Ctrl Pts',(18.3958701776758,-0.939731762255589,
26.6729314738328));
#48667=CARTESIAN_POINT('Ctrl Pts',(18.4276977863706,-0.907617561427819,
26.2012785620111));
#48668=CARTESIAN_POINT('Ctrl Pts',(18.4595253950654,-0.653330762540545,
25.8027468504271));
#48669=CARTESIAN_POINT('Ctrl Pts',(18.4913530037602,-0.239120318182226,
25.5748920741108));
#48670=CARTESIAN_POINT('Ctrl Pts',(18.5231806124551,0.233623611157383,25.5734886040687));
#48671=CARTESIAN_POINT('Ctrl Pts',(18.5550082211498,0.64917987353908,25.7988804247766));
#48672=CARTESIAN_POINT('Ctrl Pts',(18.5868358298447,0.905827494345743,26.1958949994812));
#48673=CARTESIAN_POINT('Ctrl Pts',(18.6186634385395,0.940742964858958,26.6673496464969));
#48674=CARTESIAN_POINT('Ctrl Pts',(18.6504910472343,0.745379688357512,27.0978397598884));
#48675=CARTESIAN_POINT('Ctrl Pts',(18.6823186559291,0.367559383700563,27.3819882943641));
#48676=CARTESIAN_POINT('Ctrl Pts',(18.7141462646239,-0.100233552067108,
27.4502402248901));
#48677=CARTESIAN_POINT('Ctrl Pts',(18.7459738733188,-0.543490928624728,
27.2858885824934));
#48678=CARTESIAN_POINT('Ctrl Pts',(18.7778014820136,-0.853710433012601,
26.9291640098336));
#48679=CARTESIAN_POINT('Ctrl Pts',(18.8096290907084,-0.95495530914884,26.4673869672972));
#48680=CARTESIAN_POINT('Ctrl Pts',(18.8414566994032,-0.822442430816195,
26.0135930719367));
#48681=CARTESIAN_POINT('Ctrl Pts',(18.873284308098,-0.488608828429489,25.678863796526));
#48682=CARTESIAN_POINT('Ctrl Pts',(18.9051119167929,-0.0351716161159826,
25.5451355021236));
#48683=CARTESIAN_POINT('Ctrl Pts',(18.9369395254877,0.426875043908396,25.6451427319677));
#48684=CARTESIAN_POINT('Ctrl Pts',(18.9687671341825,0.784429535379528,25.954405319031));
#48685=CARTESIAN_POINT('Ctrl Pts',(19.0005947428773,0.949968249657067,26.3972207390307));
#48686=CARTESIAN_POINT('Ctrl Pts',(19.0324223515721,0.88296996287263,26.8651948747223));
#48687=CARTESIAN_POINT('Ctrl Pts',(19.0642499602669,0.599834781719817,27.2437751585608));
#48688=CARTESIAN_POINT('Ctrl Pts',(19.0960775689618,0.169869660374138,27.4402912050732));
#48689=CARTESIAN_POINT('Ctrl Pts',(19.1279051776566,-0.301676831103628,
27.4066390359068));
#48690=CARTESIAN_POINT('Ctrl Pts',(19.1597327863514,-0.699377669708671,
27.1510561626821));
#48691=CARTESIAN_POINT('Ctrl Pts',(19.1915603950462,-0.925882064643884,
26.7361051761929));
#48692=CARTESIAN_POINT('Ctrl Pts',(19.223388003741,-0.925745370520436,26.263359426949));
#48693=CARTESIAN_POINT('Ctrl Pts',(19.2552156124358,-0.699001047869608,
25.848539497029));
#48694=CARTESIAN_POINT('Ctrl Pts',(19.2870432211307,-0.301152472537305,
25.5931866563957));
#48695=CARTESIAN_POINT('Ctrl Pts',(19.3188708298255,0.170413401093204,25.5598071875504));
#48696=CARTESIAN_POINT('Ctrl Pts',(19.3506984385203,0.600264805582684,25.7565718494482));
#48697=CARTESIAN_POINT('Ctrl Pts',(19.3825260472151,0.883181006923094,26.1353158066706));
#48698=CARTESIAN_POINT('Ctrl Pts',(19.4143536559099,0.949908653707736,26.6033286091321));
#48699=CARTESIAN_POINT('Ctrl Pts',(19.4461812646048,0.784113887538146,27.0460482242658));
#48700=CARTESIAN_POINT('Ctrl Pts',(19.4780088732995,0.426380609755225,27.3551039863542));
#48701=CARTESIAN_POINT('Ctrl Pts',(19.5098364819944,-0.0357238071158677,
27.4548439984936));
#48702=CARTESIAN_POINT('Ctrl Pts',(19.5416640906892,-0.489083608598873,
27.3208535043806));
#48703=CARTESIAN_POINT('Ctrl Pts',(19.573491699384,-0.822723581902726,26.9859312293269));
#48704=CARTESIAN_POINT('Ctrl Pts',(19.6053193080788,-0.954974009262693,
26.5320607780124));
#48705=CARTESIAN_POINT('Ctrl Pts',(19.6371469167737,-0.853462105817896,
26.070342362122));
#48706=CARTESIAN_POINT('Ctrl Pts',(19.6689745254685,-0.543036358462768,
25.7137972492788));
#48707=CARTESIAN_POINT('Ctrl Pts',(19.7008021341633,-0.0996840145356615,
25.5497019682752));
#48708=CARTESIAN_POINT('Ctrl Pts',(19.7326297428581,0.368069378378971,25.6182244137232));
#48709=CARTESIAN_POINT('Ctrl Pts',(19.7644573515529,0.745725287013211,25.9025913892794));
#48710=CARTESIAN_POINT('Ctrl Pts',(19.7962849602477,0.940839598136492,26.3331944172625));
#48711=CARTESIAN_POINT('Ctrl Pts',(19.8281125689426,0.905651455747343,26.8046287782806));
#48712=CARTESIAN_POINT('Ctrl Pts',(19.8599401776374,0.648774353094571,27.2014948970739));
#48713=CARTESIAN_POINT('Ctrl Pts',(19.8917677863322,0.233087687590096,27.426646308873));
#48714=CARTESIAN_POINT('Ctrl Pts',(19.923595395027,-0.239655107824156,27.4249695568762));
#48715=CARTESIAN_POINT('Ctrl Pts',(19.9554230037218,-0.653734174120269,
27.1968750830969));
#48716=CARTESIAN_POINT('Ctrl Pts',(19.9872506124167,-0.907789592875371,
26.7981967587369));
#48717=CARTESIAN_POINT('Ctrl Pts',(20.0190782211114,-0.939632669668737,
26.3265246474417));
#48718=CARTESIAN_POINT('Ctrl Pts',(20.0509058298063,-0.741468729693499,
25.8973165219282));
#48719=CARTESIAN_POINT('Ctrl Pts',(20.0827334385011,-0.361805129213555,
25.6156356518217));
#48720=CARTESIAN_POINT('Ctrl Pts',(20.1145610471959,0.106422567756699,25.5504329992433));
#48721=CARTESIAN_POINT('Ctrl Pts',(20.1463886558907,0.548599725918852,25.7176691284529));
#48722=CARTESIAN_POINT('Ctrl Pts',(20.1782162645855,0.856488464327402,26.0764073155399));
#48723=CARTESIAN_POINT('Ctrl Pts',(20.2100438732804,0.954722554770033,26.5388342022888));
#48724=CARTESIAN_POINT('Ctrl Pts',(20.2418714819751,0.8192558664373,26.9917550987657));
#48725=CARTESIAN_POINT('Ctrl Pts',(20.27369909067,0.483248473324846,27.3243022290903));
#48726=CARTESIAN_POINT('Ctrl Pts',(20.3055266993648,0.0289495996207101,
27.4550733859426));
#48727=CARTESIAN_POINT('Ctrl Pts',(20.3373543080596,-0.432435672056107,
27.3520578861717));
#48728=CARTESIAN_POINT('Ctrl Pts',(20.3691819167544,-0.787967622446194,
27.0404722729526));
#48729=CARTESIAN_POINT('Ctrl Pts',(20.4010095254493,-0.950617728686493,
26.5965877101963));
#48730=CARTESIAN_POINT('Ctrl Pts',(20.4328371341441,-0.880571851783068,
26.1290600241261));
#48731=CARTESIAN_POINT('Ctrl Pts',(20.4646647428389,-0.594976099681679,
25.7523324985921));
#48732=CARTESIAN_POINT('Ctrl Pts',(20.4964923515337,-0.163739734866541,
25.5586219935223));
#48733=CARTESIAN_POINT('Ctrl Pts',(20.5283199602285,0.307577492565278,25.5953457356972));
#48734=CARTESIAN_POINT('Ctrl Pts',(20.5601475689234,0.703604679778453,25.8535143416533));
#48735=CARTESIAN_POINT('Ctrl Pts',(20.5919751776182,0.927400719007669,26.269932274671));
#48736=CARTESIAN_POINT('Ctrl Pts',(20.623802786313,0.924183926932062,26.7426670992418));
#48737=CARTESIAN_POINT('Ctrl Pts',(20.6556303950078,0.694741722691852,27.1560009074729));
#48738=CARTESIAN_POINT('Ctrl Pts',(20.6874580037026,0.295237880303865,27.4087562081701));
#48739=CARTESIAN_POINT('Ctrl Pts',(20.7192856123974,-0.176535463004856,
27.4390625549747));
#48740=CARTESIAN_POINT('Ctrl Pts',(20.7511132210923,-0.605095754543117,
27.2395014399499));
#48741=CARTESIAN_POINT('Ctrl Pts',(20.782940829787,-0.885538304058988,26.8589222254171));
#48742=CARTESIAN_POINT('Ctrl Pts',(20.8147684384819,-0.949215270463799,
26.3904846030352));
#48743=CARTESIAN_POINT('Ctrl Pts',(20.8465960471767,-0.780539553018697,
25.9488545944785));
#48744=CARTESIAN_POINT('Ctrl Pts',(20.8784236558715,-0.420800263759921,
25.6421361472392));
#48745=CARTESIAN_POINT('Ctrl Pts',(20.9102512645663,0.041944185331135,25.545409021009));
#48746=CARTESIAN_POINT('Ctrl Pts',(20.9420788732612,0.494421370149437,25.6823504659124));
#48747=CARTESIAN_POINT('Ctrl Pts',(20.9739064819559,0.825872128316555,26.0194394111832));
#48748=CARTESIAN_POINT('Ctrl Pts',(21.0057340906508,0.955162626843708,26.4741618860005));
#48749=CARTESIAN_POINT('Ctrl Pts',(21.0375616993456,0.850644624005495,26.9352091169824));
#48750=CARTESIAN_POINT('Ctrl Pts',(21.0693893080404,0.537902451645026,27.2897241318133));
#48751=CARTESIAN_POINT('Ctrl Pts',(21.1012169167353,0.0934903808134796,
27.4509273371553));
#48752=CARTESIAN_POINT('Ctrl Pts',(21.1330445254301,-0.373806636744173,
27.379358772163));
#48753=CARTESIAN_POINT('Ctrl Pts',(21.1648721341249,-0.749601781132445,
27.09253727442));
#48754=CARTESIAN_POINT('Ctrl Pts',(21.1966997428197,-0.941906424383186,
26.660672149297));
#48755=CARTESIAN_POINT('Ctrl Pts',(21.2285273515145,-0.90364747215577,26.1894770573363));
#48756=CARTESIAN_POINT('Ctrl Pts',(21.2603549602093,-0.644190102727395,
25.7942930045677));
#48757=CARTESIAN_POINT('Ctrl Pts',(21.2921825689042,-0.227045321459216,
25.5718547129584));
#48758=CARTESIAN_POINT('Ctrl Pts',(21.324010177599,0.245676515339092,25.5766115109745));
#48759=CARTESIAN_POINT('Ctrl Pts',(21.3558377862938,0.658260678972873,25.8073990107051));
#48760=CARTESIAN_POINT('Ctrl Pts',(21.3876653949886,0.909713179230154,26.2077241313605));
#48761=CARTESIAN_POINT('Ctrl Pts',(21.4194930036834,0.938482474417972,26.6795936999572));
#48762=CARTESIAN_POINT('Ctrl Pts',(21.4513206123782,0.737526302198827,27.1075016093962));
#48763=CARTESIAN_POINT('Ctrl Pts',(21.4831482210731,0.356035512535034,27.3867028621065));
#48764=CARTESIAN_POINT('Ctrl Pts',(21.5149758297678,-0.112607063933625,
27.4488534665618));
#48765=CARTESIAN_POINT('Ctrl Pts',(21.5468034384627,-0.553685236057366,
27.2787399509632));
#48766=CARTESIAN_POINT('Ctrl Pts',(21.5786310471575,-0.859230137057964,
26.9180033772894));
#48767=CARTESIAN_POINT('Ctrl Pts',(21.6104586558523,-0.954449272552715,
26.4549462767619));
#48768=CARTESIAN_POINT('Ctrl Pts',(21.6422862645472,-0.816034524378642,
26.002917605546));
#48769=CARTESIAN_POINT('Ctrl Pts',(21.6741138732419,-0.477867604327989,
25.6725667370791));
#48770=CARTESIAN_POINT('Ctrl Pts',(21.7059414819368,-0.0227263541696066,
25.544758268981));
#48771=CARTESIAN_POINT('Ctrl Pts',(21.7377690906316,0.437977943223417,25.6507776656824));
#48772=CARTESIAN_POINT('Ctrl Pts',(21.7695966993264,0.791472260181452,25.9646730781875));
#48773=CARTESIAN_POINT('Ctrl Pts',(21.8014243080212,0.951226853845677,26.4096079407421));
#48774=CARTESIAN_POINT('Ctrl Pts',(21.833251916716,0.878136360290474,26.8766693305671));
#48775=CARTESIAN_POINT('Ctrl Pts',(21.8650795254109,0.590092160817773,27.251528105659));
#48776=CARTESIAN_POINT('Ctrl Pts',(21.8969071341057,0.157602858583708,27.4424248462452));
#48777=CARTESIAN_POINT('Ctrl Pts',(21.9287347428005,-0.313465097317032,
27.4026310899908));
#48778=CARTESIAN_POINT('Ctrl Pts',(21.9605623514953,-0.707801821724523,
27.1418877105986));
#48779=CARTESIAN_POINT('Ctrl Pts',(21.9923899601901,-0.928880005072949,
26.7240205080561));
#48780=CARTESIAN_POINT('Ctrl Pts',(22.0242175688849,-0.922583251598293,
26.2513166758218));
#48781=CARTESIAN_POINT('Ctrl Pts',(22.0560451775798,-0.690452905624547,
25.8394865353616));
#48782=CARTESIAN_POINT('Ctrl Pts',(22.0878727862746,-0.289310755178418,
25.5893395041004));
#48783=CARTESIAN_POINT('Ctrl Pts',(22.1197003949694,0.182650030959813,25.5621075658454));
#48784=CARTESIAN_POINT('Ctrl Pts',(22.1515280036642,0.609901017098679,25.7644566625983));
#48785=CARTESIAN_POINT('Ctrl Pts',(22.183355612359,0.887858009961992,26.1468549787971));
#48786=CARTESIAN_POINT('Ctrl Pts',(22.2151832210538,0.94848159289027,26.6156975358526));
#48787=CARTESIAN_POINT('Ctrl Pts',(22.2470108297487,0.776932084478994,27.0562191905725));
#48788=CARTESIAN_POINT('Ctrl Pts',(22.2788384384435,0.415202054730778,27.3605873027191));
#48789=CARTESIAN_POINT('Ctrl Pts',(22.3106660471383,-0.0481627830094708,
27.4542974369591));
#48790=CARTESIAN_POINT('Ctrl Pts',(22.3424936558331,-0.4997381434392,27.31441085445));
#48791=CARTESIAN_POINT('Ctrl Pts',(22.3743212645279,-0.828985616335545,
26.975169548438));
#48792=CARTESIAN_POINT('Ctrl Pts',(22.4061488732227,-0.955310697628965,
26.5196143531548));
#48793=CARTESIAN_POINT('Ctrl Pts',(22.4379764819176,-0.847791032202123,
26.0592578786051));
#48794=CARTESIAN_POINT('Ctrl Pts',(22.4698040906124,-0.532745710788099,
25.7067880110015));
#48795=CARTESIAN_POINT('Ctrl Pts',(22.5016316993072,-0.0872927784106915,
25.5484837244212));
#48796=CARTESIAN_POINT('Ctrl Pts',(22.533459308002,0.379528026961983,25.6230953708616));
#48797=CARTESIAN_POINT('Ctrl Pts',(22.5652869166968,0.753446454544427,25.9123592151761));
#48798=CARTESIAN_POINT('Ctrl Pts',(22.5971145253917,0.942933266561886,26.3454681047002));
#48799=CARTESIAN_POINT('Ctrl Pts',(22.6289421340865,0.90160512859444,26.8164039253015));
#48800=CARTESIAN_POINT('Ctrl Pts',(22.6607697427813,0.639578506394438,27.2098891364236));
#48801=CARTESIAN_POINT('Ctrl Pts',(22.6925973514761,0.220993317220635,27.4296048653045));
#48802=CARTESIAN_POINT('Ctrl Pts',(22.7244249601709,-0.251687493849366,
27.421768223196));
#48803=CARTESIAN_POINT('Ctrl Pts',(22.7562525688658,-0.662759240561632,
27.1882974944776));
#48804=CARTESIAN_POINT('Ctrl Pts',(22.7880801775606,-0.911598148125007,
26.786342571388));
#48805=CARTESIAN_POINT('Ctrl Pts',(22.8199077862554,-0.937292440446401,
26.314295576423));
#48806=CARTESIAN_POINT('Ctrl Pts',(22.8517353949502,-0.733552566602793,
25.8877060478133));
#48807=CARTESIAN_POINT('Ctrl Pts',(22.883563003645,-0.350250782096009,25.6109962646337));
#48808=CARTESIAN_POINT('Ctrl Pts',(22.9153906123398,0.118786779923891,25.5519003466042));
#48809=CARTESIAN_POINT('Ctrl Pts',(22.9472182210346,0.558747242175138,25.7248840272477));
#48810=CARTESIAN_POINT('Ctrl Pts',(22.9790458297295,0.861935335341246,26.0876036741868));
#48811=CARTESIAN_POINT('Ctrl Pts',(23.0108734384243,0.954135473821638,26.5512713316502));
#48812=CARTESIAN_POINT('Ctrl Pts',(23.0427010471191,0.812778541532895,27.0023885889206));
#48813=CARTESIAN_POINT('Ctrl Pts',(23.0745286558139,0.472466449780163,27.3305291720862));
#48814=CARTESIAN_POINT('Ctrl Pts',(23.1063562645087,0.0165021439813753,
27.4553695259417));
#48815=CARTESIAN_POINT('Ctrl Pts',(23.1381838732036,-0.443501622161829,
27.3463507328489));
#48816=CARTESIAN_POINT('Ctrl Pts',(23.1700114818984,-0.794943299801397,
27.0301588459649));
#48817=CARTESIAN_POINT('Ctrl Pts',(23.2018390905932,-0.951795599283248,
26.5841925711631));
#48818=CARTESIAN_POINT('Ctrl Pts',(23.233666699288,-0.875663591778624,26.1176173044091));
#48819=CARTESIAN_POINT('Ctrl Pts',(23.2654943079828,-0.585183172453782,
25.7446431925699));
#48820=CARTESIAN_POINT('Ctrl Pts',(23.2973219166776,-0.151459292036076,
25.5565683200624));
#48821=CARTESIAN_POINT('Ctrl Pts',(23.3291495253724,0.319339395428713,25.5994304011453));
#48822=CARTESIAN_POINT('Ctrl Pts',(23.3609771340673,0.711968917377853,25.8627374853784));
#48823=CARTESIAN_POINT('Ctrl Pts',(23.3928047427621,0.930319860043684,26.2820362189208));
#48824=CARTESIAN_POINT('Ctrl Pts',(23.4246323514569,0.920943412468097,26.7546889924705));
#48825=CARTESIAN_POINT('Ctrl Pts',(23.4564599601517,0.686134778728554,27.1649979829091));
#48826=CARTESIAN_POINT('Ctrl Pts',(23.4882875688465,0.283371348768303,27.4125261259554));
#48827=CARTESIAN_POINT('Ctrl Pts',(23.5201151775414,-0.188756845393764,
27.4366824996609));
#48828=CARTESIAN_POINT('Ctrl Pts',(23.5519427862362,-0.614680389265223,
27.2315540109293));
#48829=CARTESIAN_POINT('Ctrl Pts',(23.583770394931,-0.890140026160248,26.8473528259298));
#48830=CARTESIAN_POINT('Ctrl Pts',(23.6155980036258,-0.947707652131871,
26.3781252366373));
#48831=CARTESIAN_POINT('Ctrl Pts',(23.6474256123206,-0.773291635056603,
25.9387306359639));
#48832=CARTESIAN_POINT('Ctrl Pts',(23.6792532210155,-0.409586220312577,
25.6367257793817));
#48833=CARTESIAN_POINT('Ctrl Pts',(23.7110808297102,0.0543793361704953,
25.546036615141));
#48834=CARTESIAN_POINT('Ctrl Pts',(23.7429084384051,0.505033702770359,25.6888623970496));
#48835=CARTESIAN_POINT('Ctrl Pts',(23.7747360470999,0.832063913791676,26.0302416629588));
#48836=CARTESIAN_POINT('Ctrl Pts',(23.8065636557947,0.95541821533284,26.4866102403221));
#48837=CARTESIAN_POINT('Ctrl Pts',(23.8383912644896,0.844901451543165,26.9462564162388));
#48838=CARTESIAN_POINT('Ctrl Pts',(23.8702188731843,0.527566354796399,27.2966661742165));
#48839=CARTESIAN_POINT('Ctrl Pts',(23.9020464818792,0.0810914704164689,
27.4520648219947));
#48840=CARTESIAN_POINT('Ctrl Pts',(23.933874090574,-0.385233306158512,27.3744132613817));
#48841=CARTESIAN_POINT('Ctrl Pts',(23.9657016992688,-0.757259144042203,
27.082719349789));
#48842=CARTESIAN_POINT('Ctrl Pts',(23.9975293079636,-0.943920081082997,
26.6483850814007));
#48843=CARTESIAN_POINT('Ctrl Pts',(24.0293569166584,-0.899524511761129,
26.1777285234543));
#48844=CARTESIAN_POINT('Ctrl Pts',(24.0611845253532,-0.634939759858623,
25.7859588574846));
#48845=CARTESIAN_POINT('Ctrl Pts',(24.0930121340481,-0.214931931782802,
25.5689750182975));
#48846=CARTESIAN_POINT('Ctrl Pts',(24.1248397427429,0.257687788188069,25.579891171832));
#48847=CARTESIAN_POINT('Ctrl Pts',(24.1566673514377,0.667229667921932,25.8160352186707));
#48848=CARTESIAN_POINT('Ctrl Pts',(24.1884949601325,0.913444419542706,26.2196028811483));
#48849=CARTESIAN_POINT('Ctrl Pts',(24.2203225688273,0.936062618271151,26.6918072640162));
#48850=CARTESIAN_POINT('Ctrl Pts',(24.2521501775222,0.729547691591071,27.1170603030079));
#48851=CARTESIAN_POINT('Ctrl Pts',(24.283977786217,0.344451183459123,27.391266870285));
#48852=CARTESIAN_POINT('Ctrl Pts',(24.3158053949118,-0.124961453397658,
27.4473055932585));
#48853=CARTESIAN_POINT('Ctrl Pts',(24.3476330036066,-0.563785529389269,
27.2714590907529));
#48854=CARTESIAN_POINT('Ctrl Pts',(24.3794606123014,-0.864603944341185,
26.9067717680514));
#48855=CARTESIAN_POINT('Ctrl Pts',(24.4112882209962,-0.953781171897604,
26.4425132364135));
#48856=CARTESIAN_POINT('Ctrl Pts',(24.4431158296911,-0.809488056117004,
25.9923265430831));
#48857=CARTESIAN_POINT('Ctrl Pts',(24.4749434383859,-0.467045238961159,
25.6664101748356));
#48858=CARTESIAN_POINT('Ctrl Pts',(24.5067710470807,-0.0102772332746646,
25.5445432347142));
#48859=CARTESIAN_POINT('Ctrl Pts',(24.5385986557755,0.449006474390322,25.6565567963345));
#48860=CARTESIAN_POINT('Ctrl Pts',(24.5704262644703,0.79838059395987,25.9750317352046));
#48861=CARTESIAN_POINT('Ctrl Pts',(24.6022538731651,0.952323940855888,26.4220104909188));
#48862=CARTESIAN_POINT('Ctrl Pts',(24.63408148186,0.873153651216892,26.8880798284125));
#48863=CARTESIAN_POINT('Ctrl Pts',(24.6659090905548,0.580249342976974,27.2591534441921));
#48864=CARTESIAN_POINT('Ctrl Pts',(24.6977366992496,0.145309296018941,27.4443984648148));
#48865=CARTESIAN_POINT('Ctrl Pts',(24.7295643079444,-0.325200137535511,
27.3984698784049));
#48866=CARTESIAN_POINT('Ctrl Pts',(24.7613919166392,-0.716105789844623,
27.1326102667559));
#48867=CARTESIAN_POINT('Ctrl Pts',(24.7932195253341,-0.931720222797812,
26.7118978015073));
#48868=CARTESIAN_POINT('Ctrl Pts',(24.8250471340289,-0.919264479152886,
26.2393161508229));
#48869=CARTESIAN_POINT('Ctrl Pts',(24.8568747427237,-0.681787525309043,
25.8305457280837));
#48870=CARTESIAN_POINT('Ctrl Pts',(24.8887023514185,-0.277419913202257,
25.5856469808586));
#48871=CARTESIAN_POINT('Ctrl Pts',(24.9205299601133,0.194855647071497,25.5645671971444));
#48872=CARTESIAN_POINT('Ctrl Pts',(24.9523575688081,0.6194336681577,25.7724663701197));
#48873=CARTESIAN_POINT('Ctrl Pts',(24.984185177503,0.892384255781827,26.1584541145223));
#48874=CARTESIAN_POINT('Ctrl Pts',(25.0160127861977,0.946893481042504,26.628046817271));
#48875=CARTESIAN_POINT('Ctrl Pts',(25.0478403948926,0.769618359289142,27.0662957115316));
#48876=CARTESIAN_POINT('Ctrl Pts',(25.0796680035874,0.403952998898319,27.3659244923982));
#48877=CARTESIAN_POINT('Ctrl Pts',(25.1114956122822,-0.0605935809206184,
27.4535888368711));
#48878=CARTESIAN_POINT('Ctrl Pts',(25.1433232209771,-0.510307823345631,
27.3078299185387));
#48879=CARTESIAN_POINT('Ctrl Pts',(25.1751508296718,-0.835106890010742,
26.964327184333));
#48880=CARTESIAN_POINT('Ctrl Pts',(25.2069784383667,-0.955485175391192,
26.5071645978036));
#48881=CARTESIAN_POINT('Ctrl Pts',(25.2388060470615,-0.841976004691772,
26.0482482325687));
#48882=CARTESIAN_POINT('Ctrl Pts',(25.2706336557563,-0.522364603534392,
25.699913459163));
#48883=CARTESIAN_POINT('Ctrl Pts',(25.3024612644511,-0.0748867200772622,
25.547427046883));
#48884=CARTESIAN_POINT('Ctrl Pts',(25.3342888731459,0.390922232143804,25.6281152253481));
#48885=CARTESIAN_POINT('Ctrl Pts',(25.3661164818408,0.761039687776565,25.9222268217692));
#48886=CARTESIAN_POINT('Ctrl Pts',(25.3979440905356,0.944866826056054,26.3577680314671));
#48887=CARTESIAN_POINT('Ctrl Pts',(25.4297716992304,0.897405709978404,26.8281253473178));
#48888=CARTESIAN_POINT('Ctrl Pts',(25.4615993079252,0.630274060035337,27.218162837454));
#48889=CARTESIAN_POINT('Ctrl Pts',(25.49342691662,0.208861422452774,27.4324055759519));
#48890=CARTESIAN_POINT('Ctrl Pts',(25.5252545253149,-0.263677143642244,
27.4184103743823));
#48891=CARTESIAN_POINT('Ctrl Pts',(25.5570821340096,-0.671671771282482,
27.1796030337761));
#48892=CARTESIAN_POINT('Ctrl Pts',(25.5889097427045,-0.915251915110534,
26.7744397634122));
#48893=CARTESIAN_POINT('Ctrl Pts',(25.6207373513993,-0.934793060094999,
26.3020980377986));
#48894=CARTESIAN_POINT('Ctrl Pts',(25.6525649600941,-0.725511847177558,
25.8781995404594));
#48895=CARTESIAN_POINT('Ctrl Pts',(25.6843925687889,-0.338636962806214,
25.6065078292329));
#48896=CARTESIAN_POINT('Ctrl Pts',(25.7162201774838,0.131130822216466,25.5535286800947));
#48897=CARTESIAN_POINT('Ctrl Pts',(25.7480477861786,0.568799883866499,25.7322305398899));
#48898=CARTESIAN_POINT('Ctrl Pts',(25.7798753948734,0.867235850694155,26.0988700570622));
#48899=CARTESIAN_POINT('Ctrl Pts',(25.8117030035682,0.953386381973287,26.5636997555226));
#48900=CARTESIAN_POINT('Ctrl Pts',(25.843530612263,0.80616320752463,27.0129367734926));
#48901=CARTESIAN_POINT('Ctrl Pts',(25.8753582209578,0.461604202545949,27.3366150933761));
#48902=CARTESIAN_POINT('Ctrl Pts',(25.9071858296527,0.00405188527124226,
27.4555034431848));
#48903=CARTESIAN_POINT('Ctrl Pts',(25.9390134383475,-0.454492264288568,
27.3404998742768));
#48904=CARTESIAN_POINT('Ctrl Pts',(25.9708410470423,-0.801784000403587,
27.019755390933));
#48905=CARTESIAN_POINT('Ctrl Pts',(26.0026686557371,-0.952811849223926,
26.5717831508947));
#48906=CARTESIAN_POINT('Ctrl Pts',(26.034496264432,-0.870606658202922,26.1062394853173));
#48907=CARTESIAN_POINT('Ctrl Pts',(26.0663238731267,-0.575290857187556,
25.7370821971392));
#48908=CARTESIAN_POINT('Ctrl Pts',(26.0981514818216,-0.139153178128873,
25.5546747421343));
#48909=CARTESIAN_POINT('Ctrl Pts',(26.1299790905164,0.331047162702991,25.6036681673243));
#48910=CARTESIAN_POINT('Ctrl Pts',(26.1618066992112,0.720212097625758,25.8720684860043));
#48911=CARTESIAN_POINT('Ctrl Pts',(26.193634307906,0.933081347121382,26.2941778330969));
#48912=CARTESIAN_POINT('Ctrl Pts',(26.2254619166008,0.917545931470056,26.7666663937008));
#48913=CARTESIAN_POINT('Ctrl Pts',(26.2572895252956,0.677412446761784,27.1738844955338));
#48914=CARTESIAN_POINT('Ctrl Pts',(26.2891171339905,0.271454591702591,27.416136653851));
#48915=CARTESIAN_POINT('Ctrl Pts',(26.3209447426853,-0.200942189437803,
27.434151796482));
#48916=CARTESIAN_POINT('Ctrl Pts',(26.3527723513801,-0.624168219542933,
27.223466435793));
#48917=CARTESIAN_POINT('Ctrl Pts',(26.3845999600749,-0.894576003957899,
26.8357550859606));
#48918=CARTESIAN_POINT('Ctrl Pts',(26.4164275687697,-0.946069180424221,
26.365724145282));
#48919=CARTESIAN_POINT('Ctrl Pts',(26.4376459745663,-0.82591582866072,26.0744774398212));
#48920=CARTESIAN_POINT('Ctrl Pts',(26.4482551774646,-0.734601664004067,
25.9520568295746));
#48921=CARTESIAN_POINT('Ctrl Pts',(9.60000015794368,-0.899145364714185,
26.9202321182148));
#48922=CARTESIAN_POINT('Ctrl Pts',(9.61060936084195,-0.969176614135344,
26.770390469819));
#48923=CARTESIAN_POINT('Ctrl Pts',(9.63182776663849,-1.03281304011026,26.4351748220049));
#48924=CARTESIAN_POINT('Ctrl Pts',(9.66365537533331,-0.87523841633845,25.9479403018373));
#48925=CARTESIAN_POINT('Ctrl Pts',(9.69548298402813,-0.503515492261773,
25.5959674242812));
#48926=CARTESIAN_POINT('Ctrl Pts',(9.72731059272294,-0.00849156889496621,
25.4652231538941));
#48927=CARTESIAN_POINT('Ctrl Pts',(9.75913820141777,0.488585575395564,25.58780926119));
#48928=CARTESIAN_POINT('Ctrl Pts',(9.79096581011257,0.866078206808652,25.933667292316));
#48929=CARTESIAN_POINT('Ctrl Pts',(9.82279341880741,1.03156168020563,26.4181638872238));
#48930=CARTESIAN_POINT('Ctrl Pts',(9.85462102750221,0.944539145419091,26.9226876762002));
#48931=CARTESIAN_POINT('Ctrl Pts',(9.88644863619703,0.62630657764322,27.3237469315434));
#48932=CARTESIAN_POINT('Ctrl Pts',(9.91827624489185,0.154765252016519,27.5231647461145));
#48933=CARTESIAN_POINT('Ctrl Pts',(9.95010385358666,-0.354660684709781,
27.4721289694078));
#48934=CARTESIAN_POINT('Ctrl Pts',(9.9819314622815,-0.777271074907365,27.1831312112822));
#48935=CARTESIAN_POINT('Ctrl Pts',(10.0137590709763,-1.00961812086333,26.7269140893577));
#48936=CARTESIAN_POINT('Ctrl Pts',(10.0455866796711,-0.994826750456996,
26.2151519256561));
#48937=CARTESIAN_POINT('Ctrl Pts',(10.0774142883659,-0.736517780875856,
25.7731160630381));
#48938=CARTESIAN_POINT('Ctrl Pts',(10.1092418970608,-0.297921040455159,
25.5090097066483));
#48939=CARTESIAN_POINT('Ctrl Pts',(10.1410695057556,0.21360198317146,25.4874819064308));
#48940=CARTESIAN_POINT('Ctrl Pts',(10.1728971144504,0.672838671527312,25.7138022978844));
#48941=CARTESIAN_POINT('Ctrl Pts',(10.2047247231452,0.967375234136969,26.1325712899329));
#48942=CARTESIAN_POINT('Ctrl Pts',(10.23655233184,1.02511384669292,26.641280938506));
#48943=CARTESIAN_POINT('Ctrl Pts',(10.2683799405348,0.831921019498759,27.1154072791165));
#48944=CARTESIAN_POINT('Ctrl Pts',(10.3002075492297,0.435087261570011,27.4388917810866));
#48945=CARTESIAN_POINT('Ctrl Pts',(10.3320351579245,-0.0682488845295447,
27.5325506242975));
#48946=CARTESIAN_POINT('Ctrl Pts',(10.3638627666193,-0.554878797469749,
27.3734576245781));
#48947=CARTESIAN_POINT('Ctrl Pts',(10.3956903753141,-0.90568327466009,27.0005561985521));
#48948=CARTESIAN_POINT('Ctrl Pts',(10.4275179840089,-1.03479100278662,26.5051266381597));
#48949=CARTESIAN_POINT('Ctrl Pts',(10.4593455927037,-0.910598479450232,
26.0084421589457));
#48950=CARTESIAN_POINT('Ctrl Pts',(10.4911732013986,-0.563506043729093,
25.6320831603431));
#48951=CARTESIAN_POINT('Ctrl Pts',(10.5230008100934,-0.0784763605841615,
25.4681762928169));
#48952=CARTESIAN_POINT('Ctrl Pts',(10.5548284187882,0.425763077787955,25.5568433303679));
#48953=CARTESIAN_POINT('Ctrl Pts',(10.586656027483,0.825782538997791,25.8763800033968));
#48954=CARTESIAN_POINT('Ctrl Pts',(10.6184836361778,1.02366367059781,26.3485688559903));
#48955=CARTESIAN_POINT('Ctrl Pts',(10.6503112448726,0.970968343280062,26.8578256254456));
#48956=CARTESIAN_POINT('Ctrl Pts',(10.6821388535675,0.680595528553212,27.2794924171479));
#48957=CARTESIAN_POINT('Ctrl Pts',(10.7139664622623,0.223623837263367,27.5103519591139));
#48958=CARTESIAN_POINT('Ctrl Pts',(10.7457940709571,-0.28808738506616,27.493893535769));
#48959=CARTESIAN_POINT('Ctrl Pts',(10.7776216796519,-0.729279433098497,
27.2341459053465));
#48960=CARTESIAN_POINT('Ctrl Pts',(10.8094492883467,-0.991955565058188,
26.7946911244468));
#48961=CARTESIAN_POINT('Ctrl Pts',(10.8412768970415,-1.0118168741079,26.2831006796964));
#48962=CARTESIAN_POINT('Ctrl Pts',(10.8731045057364,-0.784001630136379,
25.8246037120171));
#48963=CARTESIAN_POINT('Ctrl Pts',(10.9049321144312,-0.36427535336417,25.5314329301442));
#48964=CARTESIAN_POINT('Ctrl Pts',(10.936759723126,0.144619691176789,25.4753518424349));
#48965=CARTESIAN_POINT('Ctrl Pts',(10.9685873318208,0.618114153333466,25.6700882002728));
#48966=CARTESIAN_POINT('Ctrl Pts',(11.0004149405156,0.94030417810739,26.0679736645627));
#48967=CARTESIAN_POINT('Ctrl Pts',(11.0322425492105,1.0323228116101,26.571612251096));
#48968=CARTESIAN_POINT('Ctrl Pts',(11.0640701579053,0.871645367267493,27.0577213063876));
#48969=CARTESIAN_POINT('Ctrl Pts',(11.0958977666001,0.497603108059459,27.4073091252309));
#48970=CARTESIAN_POINT('Ctrl Pts',(11.1277253752949,0.00175558375789874,
27.5348022128906));
#48971=CARTESIAN_POINT('Ctrl Pts',(11.1595529839897,-0.494521679308475,
27.4089923050123));
#48972=CARTESIAN_POINT('Ctrl Pts',(11.1913805926845,-0.869747961649325,
27.0606756505186));
#48973=CARTESIAN_POINT('Ctrl Pts',(11.2232082013794,-1.03207388360779,26.5751145834865));
#48974=CARTESIAN_POINT('Ctrl Pts',(11.2550358100742,-0.941764661305992,
26.0711666703802));
#48975=CARTESIAN_POINT('Ctrl Pts',(11.286863418769,-0.62092654485511,25.6721902828718));
#48976=CARTESIAN_POINT('Ctrl Pts',(11.3186910274638,-0.148095562654985,
25.4758484456881));
#48977=CARTESIAN_POINT('Ctrl Pts',(11.3505186361586,0.360986839554778,25.5302024935349));
#48978=CARTESIAN_POINT('Ctrl Pts',(11.3823462448535,0.781705449466869,25.8219474267054));
#48979=CARTESIAN_POINT('Ctrl Pts',(11.4141738535483,1.01107509480216,26.2796687617508));
#48980=CARTESIAN_POINT('Ctrl Pts',(11.4460014622431,0.992949762800771,26.7913236523723));
#48981=CARTESIAN_POINT('Ctrl Pts',(11.4778290709379,0.73176624421736,27.2316671823319));
#48982=CARTESIAN_POINT('Ctrl Pts',(11.5096566796327,0.291458078058921,27.4929103134785));
#48983=CARTESIAN_POINT('Ctrl Pts',(11.5414842883276,-0.22019435401471,27.5111049146046));
#48984=CARTESIAN_POINT('Ctrl Pts',(11.5733118970223,-0.677946737578888,
27.2817972389845));
#48985=CARTESIAN_POINT('Ctrl Pts',(11.6051395057172,-0.96974862615495,26.8611181301848));
#48986=CARTESIAN_POINT('Ctrl Pts',(11.636967114412,-1.02417159452383,26.3520430912457));
#48987=CARTESIAN_POINT('Ctrl Pts',(11.6687947231068,-0.82789377233951,25.8791855320637));
#48988=CARTESIAN_POINT('Ctrl Pts',(11.7006223318016,-0.428960824462024,
25.5582934039976));
#48989=CARTESIAN_POINT('Ctrl Pts',(11.7324499404964,0.0749748577072528,
25.467915956625));
#48990=CARTESIAN_POINT('Ctrl Pts',(11.7642775491913,0.560557896433451,25.6301761404608));
#48991=CARTESIAN_POINT('Ctrl Pts',(11.7961051578861,0.908925346933881,26.0053552632659));
#48992=CARTESIAN_POINT('Ctrl Pts',(11.8279327665809,1.03480244108332,26.5016154892819));
#48993=CARTESIAN_POINT('Ctrl Pts',(11.8597603752757,0.907376483836781,26.9974802694154));
#48994=CARTESIAN_POINT('Ctrl Pts',(11.8915879839705,0.557839307099688,27.3715698533865));
#48995=CARTESIAN_POINT('Ctrl Pts',(11.9234155926653,0.0717520092312157,
27.5323131070799));
#48996=CARTESIAN_POINT('Ctrl Pts',(11.9552432013602,-0.431899030430357,
27.4403626584414));
#48997=CARTESIAN_POINT('Ctrl Pts',(11.987070810055,-0.829828110073699,27.1182265034833));
#48998=CARTESIAN_POINT('Ctrl Pts',(12.0188984187498,-1.02462856915081,26.6447584096265));
#48999=CARTESIAN_POINT('Ctrl Pts',(12.0507260274446,-0.968616377610574,
26.1358557773324));
#49000=CARTESIAN_POINT('Ctrl Pts',(12.0825536361394,-0.675502422158747,
25.7160898141143));
#49001=CARTESIAN_POINT('Ctrl Pts',(12.1143812448342,-0.217036300955299,
25.4882124996101));
#49002=CARTESIAN_POINT('Ctrl Pts',(12.1462088535291,0.294556827987056,25.5080045479117));
#49003=CARTESIAN_POINT('Ctrl Pts',(12.1780364622239,0.73404716669968,25.770621182829));
#49004=CARTESIAN_POINT('Ctrl Pts',(12.2098640709187,0.993854524573037,26.2117780614468));
#49005=CARTESIAN_POINT('Ctrl Pts',(12.2416916796135,1.01038222468437,26.7234870508989));
#49006=CARTESIAN_POINT('Ctrl Pts',(12.2735192883083,0.779584550958275,27.1804899924208));
#49007=CARTESIAN_POINT('Ctrl Pts',(12.3053468970032,0.357957074615781,27.4709198909334));
#49008=CARTESIAN_POINT('Ctrl Pts',(12.337174505698,-0.151292556129472,27.5236841623946));
#49009=CARTESIAN_POINT('Ctrl Pts',(12.3690021143928,-0.623508194105078,
27.325866958875));
#49010=CARTESIAN_POINT('Ctrl Pts',(12.4008297230876,-0.943099019974642,
26.9258907611119));
#49011=CARTESIAN_POINT('Ctrl Pts',(12.4326573317824,-1.03183432208061,26.4216633313571));
#49012=CARTESIAN_POINT('Ctrl Pts',(12.4644849404772,-0.867993120748392,
25.9366114624781));
#49013=CARTESIAN_POINT('Ctrl Pts',(12.496312549172,-0.491681115959126,25.5894680773928));
#49014=CARTESIAN_POINT('Ctrl Pts',(12.5281401578669,0.00498654517730746,
25.4652083126325));
#49015=CARTESIAN_POINT('Ctrl Pts',(12.5599677665617,0.500433579980453,25.594248966931));
#49016=CARTESIAN_POINT('Ctrl Pts',(12.5917953752565,0.873382495531615,25.9450029564253));
#49017=CARTESIAN_POINT('Ctrl Pts',(12.6236229839513,1.03254137506161,26.431611326497));
#49018=CARTESIAN_POINT('Ctrl Pts',(12.6554505926462,0.938950675916567,26.9349601476841));
#49019=CARTESIAN_POINT('Ctrl Pts',(12.6872782013409,0.615519901142211,27.3318376964141));
#49020=CARTESIAN_POINT('Ctrl Pts',(12.7191058100358,0.141419720339925,27.525094710052));
#49021=CARTESIAN_POINT('Ctrl Pts',(12.7509334187306,-0.367297741276047,
27.4674249692514));
#49022=CARTESIAN_POINT('Ctrl Pts',(12.7827610274254,-0.786106603006349,
27.1729451022093));
#49023=CARTESIAN_POINT('Ctrl Pts',(12.8145886361202,-1.01248916831665,26.7137390603495));
#49024=CARTESIAN_POINT('Ctrl Pts',(12.846416244815,-0.991030613759187,26.2022131224017));
#49025=CARTESIAN_POINT('Ctrl Pts',(12.8782438535099,-0.726983649544281,
25.7635806390562));
#49026=CARTESIAN_POINT('Ctrl Pts',(12.9100714622047,-0.284982740273187,
25.5052118116785));
#49027=CARTESIAN_POINT('Ctrl Pts',(12.9418990708995,0.22677737601216,25.4903511879833));
#49028=CARTESIAN_POINT('Ctrl Pts',(12.9737266795943,0.683026025518092,25.7226364104599));
#49029=CARTESIAN_POINT('Ctrl Pts',(13.0055542882891,0.97208085176103,26.1452077797962));
#49030=CARTESIAN_POINT('Ctrl Pts',(13.037381896984,1.02318586635016,26.6546265979024));
#49031=CARTESIAN_POINT('Ctrl Pts',(13.0692095056788,0.823831380843395,27.1261953032524));
#49032=CARTESIAN_POINT('Ctrl Pts',(13.1010371143736,0.422816177968262,27.4444814352468));
#49033=CARTESIAN_POINT('Ctrl Pts',(13.1328647230684,-0.0816976482255668,
27.531573650377));
#49034=CARTESIAN_POINT('Ctrl Pts',(13.1646923317632,-0.566213199612709,
27.3661531703238));
#49035=CARTESIAN_POINT('Ctrl Pts',(13.196519940458,-0.91212883520101,26.9887122771861));
#49036=CARTESIAN_POINT('Ctrl Pts',(13.2283475491529,-1.03476995185717,26.4916424518474));
#49037=CARTESIAN_POINT('Ctrl Pts',(13.2601751578477,-0.904115969959171,
25.9966184203386));
#49038=CARTESIAN_POINT('Ctrl Pts',(13.2920027665425,-0.552148890107181,
25.6248141311521));
#49039=CARTESIAN_POINT('Ctrl Pts',(13.3238303752373,-0.0650246119955593,
25.4672413148695));
#49040=CARTESIAN_POINT('Ctrl Pts',(13.3556579839321,0.438016648894992,25.5624712712837));
#49041=CARTESIAN_POINT('Ctrl Pts',(13.3874855926269,0.833838454822538,25.887193233444));
#49042=CARTESIAN_POINT('Ctrl Pts',(13.4193132013218,1.02554997206856,26.3619204697727));
#49043=CARTESIAN_POINT('Ctrl Pts',(13.4511408100166,0.966223294031546,26.8704473619132));
#49044=CARTESIAN_POINT('Ctrl Pts',(13.4829684187114,0.670380640585883,27.2882946775193));
#49045=CARTESIAN_POINT('Ctrl Pts',(13.5147960274062,0.210439551423907,27.5131800911359));
#49046=CARTESIAN_POINT('Ctrl Pts',(13.546623636101,-0.301013766926736,27.4900552580529));
#49047=CARTESIAN_POINT('Ctrl Pts',(13.5784512447958,-0.738783739889328,
27.224580766756));
#49048=CARTESIAN_POINT('Ctrl Pts',(13.6102788534907,-0.995711294815304,
26.7817405175953));
#49049=CARTESIAN_POINT('Ctrl Pts',(13.6421064621855,-1.00890468438493,26.2699347055643));
#49050=CARTESIAN_POINT('Ctrl Pts',(13.6739340708803,-0.77513437829989,25.8144451900429));
#49051=CARTESIAN_POINT('Ctrl Pts',(13.7057616795751,-0.351623600536278,
25.526768503683));
#49052=CARTESIAN_POINT('Ctrl Pts',(13.7375892882699,0.157958998690607,25.4773232883211));
#49053=CARTESIAN_POINT('Ctrl Pts',(13.7694168969648,0.628875766860997,25.6782129401527));
#49054=CARTESIAN_POINT('Ctrl Pts',(13.8012445056596,0.94585382714805,26.0802628923397));
#49055=CARTESIAN_POINT('Ctrl Pts',(13.8330721143544,1.03130203103048,26.5850577607866));
#49056=CARTESIAN_POINT('Ctrl Pts',(13.8648997230492,0.864304027792048,27.0690318527289));
#49057=CARTESIAN_POINT('Ctrl Pts',(13.896727331744,0.485738251922189,27.4137160677679));
#49058=CARTESIAN_POINT('Ctrl Pts',(13.9285549404388,-0.0117284624329275,
27.5347372347831));
#49059=CARTESIAN_POINT('Ctrl Pts',(13.9603825491336,-0.506324237172425,
27.4024713118595));
#49060=CARTESIAN_POINT('Ctrl Pts',(13.9922101578285,-0.876979954196896,
27.0492948769235));
#49061=CARTESIAN_POINT('Ctrl Pts',(14.0240377665233,-1.03296503498029,26.5616598604102));
#49062=CARTESIAN_POINT('Ctrl Pts',(14.0558653752181,-0.936096831931118,
26.0589314983745));
#49063=CARTESIAN_POINT('Ctrl Pts',(14.0876929839129,-0.610087128517846,
25.6641696359342));
#49064=CARTESIAN_POINT('Ctrl Pts',(14.1195205926077,-0.13473787473667,25.474005649631));
#49065=CARTESIAN_POINT('Ctrl Pts',(14.1513482013026,0.373593051153504,25.5349886352962));
#49066=CARTESIAN_POINT('Ctrl Pts',(14.1831758099974,0.790474386203466,25.8321909354959));
#49067=CARTESIAN_POINT('Ctrl Pts',(14.2150034186922,1.01386026151516,26.2928621908052));
#49068=CARTESIAN_POINT('Ctrl Pts',(14.246831027387,0.989069395320457,26.8042374617269));
#49069=CARTESIAN_POINT('Ctrl Pts',(14.2786586360818,0.72217019430702,27.2411402784441));
#49070=CARTESIAN_POINT('Ctrl Pts',(14.3104862447766,0.278495304927702,27.4966238342578));
#49071=CARTESIAN_POINT('Ctrl Pts',(14.3423138534715,-0.233350771276214,
27.5081498496863));
#49072=CARTESIAN_POINT('Ctrl Pts',(14.3741414621663,-0.688076318900794,
27.2728969408954));
#49073=CARTESIAN_POINT('Ctrl Pts',(14.4059690708611,-0.97437181239019,26.8484512492403));
#49074=CARTESIAN_POINT('Ctrl Pts',(14.4377966795559,-1.02215670378408,26.3387102768714));
#49075=CARTESIAN_POINT('Ctrl Pts',(14.4696242882507,-0.819734017582471,
25.8684504435156));
#49076=CARTESIAN_POINT('Ctrl Pts',(14.5014518969455,-0.416653582864778,
25.5527838188863));
#49077=CARTESIAN_POINT('Ctrl Pts',(14.5332795056404,0.0884169706665388,
25.4689805330763));
#49078=CARTESIAN_POINT('Ctrl Pts',(14.5651071143352,0.57184446695731,25.6375542872227));
#49079=CARTESIAN_POINT('Ctrl Pts',(14.59693472303,0.915293603463237,26.0172409282707));
#49080=CARTESIAN_POINT('Ctrl Pts',(14.6287623317248,1.03469353649247,26.5150992522442));
#49081=CARTESIAN_POINT('Ctrl Pts',(14.6605899404196,0.900817076223997,27.0092615212843));
#49082=CARTESIAN_POINT('Ctrl Pts',(14.6924175491145,0.546435034312068,27.3787647325388));
#49083=CARTESIAN_POINT('Ctrl Pts',(14.7242451578093,0.0582944544554268,
27.5331604224211));
#49084=CARTESIAN_POINT('Ctrl Pts',(14.7560727665041,-0.444115673487672,
27.4346550007571));
#49085=CARTESIAN_POINT('Ctrl Pts',(14.7879003751989,-0.837813403004803,
27.1073610158902));
#49086=CARTESIAN_POINT('Ctrl Pts',(14.8197279838937,-1.02642784023727,26.6313947893315));
#49087=CARTESIAN_POINT('Ctrl Pts',(14.8515555925885,-0.963789194129796,
26.1232652243869));
#49088=CARTESIAN_POINT('Ctrl Pts',(14.8833832012833,-0.665230401255004,
25.7073542940735));
#49089=CARTESIAN_POINT('Ctrl Pts',(14.9152108099782,-0.203833868702235,
25.4854703277639));
#49090=CARTESIAN_POINT('Ctrl Pts',(14.947038418673,0.307457927787168,25.5119269639756));
#49091=CARTESIAN_POINT('Ctrl Pts',(14.9788660273678,0.743488951599186,25.7802480422204));
#49092=CARTESIAN_POINT('Ctrl Pts',(15.0106936360626,0.997525796964821,26.2247528632895));
#49093=CARTESIAN_POINT('Ctrl Pts',(15.0425212447574,1.00738431593138,26.7366337716664));
#49094=CARTESIAN_POINT('Ctrl Pts',(15.0743488534523,0.770651301071694,27.1905905255896));
#49095=CARTESIAN_POINT('Ctrl Pts',(15.1061764621471,0.345275199982537,27.4755017878787));
#49096=CARTESIAN_POINT('Ctrl Pts',(15.1380040708419,-0.164618735868749,
27.5216258481844));
#49097=CARTESIAN_POINT('Ctrl Pts',(15.1698316795367,-0.634216643746959,
27.3176722758367));
#49098=CARTESIAN_POINT('Ctrl Pts',(15.2016592882315,-0.94856848268563,26.9135656363059));
#49099=CARTESIAN_POINT('Ctrl Pts',(15.2334868969263,-1.03072596105555,26.4082247577844));
#49100=CARTESIAN_POINT('Ctrl Pts',(15.2653145056211,-0.860578245001017,
25.9253489875511));
#49101=CARTESIAN_POINT('Ctrl Pts',(15.297142114316,-0.47977476822413,25.5831385744546));
#49102=CARTESIAN_POINT('Ctrl Pts',(15.3289697230108,0.0184698818135679,
25.465361142551));
#49103=CARTESIAN_POINT('Ctrl Pts',(15.3607973317056,0.512193400825138,25.6008467193916));
#49104=CARTESIAN_POINT('Ctrl Pts',(15.3926249404004,0.880540184932533,25.9564306073769));
#49105=CARTESIAN_POINT('Ctrl Pts',(15.4244525490953,1.03334484537939,26.445071570153));
#49106=CARTESIAN_POINT('Ctrl Pts',(15.4562801577901,0.933203250495736,26.9471581321432));
#49107=CARTESIAN_POINT('Ctrl Pts',(15.4881077664849,0.604628457604007,27.3397875505942));
#49108=CARTESIAN_POINT('Ctrl Pts',(15.5199353751797,0.128050309490577,27.526850437073));
#49109=CARTESIAN_POINT('Ctrl Pts',(15.5517629838745,-0.379872501950287,
27.4625567952799));
#49110=CARTESIAN_POINT('Ctrl Pts',(15.5835905925693,-0.79480861364516,27.1626446782048));
#49111=CARTESIAN_POINT('Ctrl Pts',(15.6154182012641,-1.01518831619457,26.7005277650094));
#49112=CARTESIAN_POINT('Ctrl Pts',(15.647245809959,-0.987066190738606,26.18932486907));
#49113=CARTESIAN_POINT('Ctrl Pts',(15.6790734186538,-0.717326082837455,
25.7541702655708));
#49114=CARTESIAN_POINT('Ctrl Pts',(15.7109010273486,-0.271996047415024,
25.501582826636));
#49115=CARTESIAN_POINT('Ctrl Pts',(15.7427286360434,0.239914260765304,25.4933919087554));
#49116=CARTESIAN_POINT('Ctrl Pts',(15.7745562447382,0.693097403341301,25.7316025173394));
#49117=CARTESIAN_POINT('Ctrl Pts',(15.8063838534331,0.976621410790803,26.1579045135308));
#49118=CARTESIAN_POINT('Ctrl Pts',(15.8382114621279,1.0210841505137,26.6679460015818));
#49119=CARTESIAN_POINT('Ctrl Pts',(15.8700390708227,0.815601856490434,27.1368770003439));
#49120=CARTESIAN_POINT('Ctrl Pts',(15.9018666795175,0.410473300754662,27.4499107175125));
#49121=CARTESIAN_POINT('Ctrl Pts',(15.9336942882123,-0.0951325397939341,
27.5304215165407));
#49122=CARTESIAN_POINT('Ctrl Pts',(15.9655218969071,-0.577451459419126,
27.3587016442818));
#49123=CARTESIAN_POINT('Ctrl Pts',(15.997349505602,-0.918419517375691,26.9767853730779));
#49124=CARTESIAN_POINT('Ctrl Pts',(16.0291771142968,-1.03457319823305,26.4781596846298));
#49125=CARTESIAN_POINT('Ctrl Pts',(16.0610047229916,-0.89747994266978,25.9848801553201));
#49126=CARTESIAN_POINT('Ctrl Pts',(16.0928323316864,-0.540697982268354,
25.617693707464));
#49127=CARTESIAN_POINT('Ctrl Pts',(16.1246599403813,-0.0515618223070227,
25.4664816981021));
#49128=CARTESIAN_POINT('Ctrl Pts',(16.156487549076,0.450195845303856,25.5682584034461));
#49129=CARTESIAN_POINT('Ctrl Pts',(16.1883151577709,0.841752785883323,25.8981105173412));
#49130=CARTESIAN_POINT('Ctrl Pts',(16.2201427664656,1.0272621363913,26.3752955292926));
#49131=CARTESIAN_POINT('Ctrl Pts',(16.2519703751605,0.961314181233222,26.8830061968657));
#49132=CARTESIAN_POINT('Ctrl Pts',(16.2837979838553,0.660051922794526,27.2969630864054));
#49133=CARTESIAN_POINT('Ctrl Pts',(16.3156255925501,0.197219533202479,27.5158361864007));
#49134=CARTESIAN_POINT('Ctrl Pts',(16.3474532012449,-0.313889037012783,
27.4860488701483));
#49135=CARTESIAN_POINT('Ctrl Pts',(16.3792808099398,-0.748162602092337,
27.2148925952254));
#49136=CARTESIAN_POINT('Ctrl Pts',(16.4111084186346,-0.999297953995706,
26.7687420715437));
#49137=CARTESIAN_POINT('Ctrl Pts',(16.4429360273294,-1.0058211838636,26.2568077962417));
#49138=CARTESIAN_POINT('Ctrl Pts',(16.4747636360242,-0.766135509581008,
25.8044030744485));
#49139=CARTESIAN_POINT('Ctrl Pts',(16.506591244719,-0.33891214244517,25.5222693307557));
#49140=CARTESIAN_POINT('Ctrl Pts',(16.5384188534138,0.171271484957023,25.4794683834794));
#49141=CARTESIAN_POINT('Ctrl Pts',(16.5702464621087,0.639530598041916,25.6864772184838));
#49142=CARTESIAN_POINT('Ctrl Pts',(16.6020740708035,0.951242871349886,26.0926233909713));
#49143=CARTESIAN_POINT('Ctrl Pts',(16.6339016794983,1.03010613661001,26.5984888277719));
#49144=CARTESIAN_POINT('Ctrl Pts',(16.6657292881931,0.856815930535437,27.080245778148));
#49145=CARTESIAN_POINT('Ctrl Pts',(16.6975568968879,0.473790918015481,27.4199678624187));
#49146=CARTESIAN_POINT('Ctrl Pts',(16.7293845055828,-0.0252105171445776,
27.5344965595417));
#49147=CARTESIAN_POINT('Ctrl Pts',(16.7612121142776,-0.518040821792485,
27.3957970801659));
#49148=CARTESIAN_POINT('Ctrl Pts',(16.7930397229724,-0.884063036604701,
27.0378208337223));
#49149=CARTESIAN_POINT('Ctrl Pts',(16.8248673316672,-1.0336807901387,26.5481946675613));
#49150=CARTESIAN_POINT('Ctrl Pts',(16.856694940362,-0.930270054438158,26.0467712192733));
#49151=CARTESIAN_POINT('Ctrl Pts',(16.8885225490569,-0.599144120132018,
25.6562909119748));
#49152=CARTESIAN_POINT('Ctrl Pts',(16.9203501577516,-0.121357308471081,
25.4723370661945));
#49153=CARTESIAN_POINT('Ctrl Pts',(16.9521777664465,0.386135827067481,25.5399386347901));
#49154=CARTESIAN_POINT('Ctrl Pts',(16.9840053751413,0.799109101409514,25.8425478375223));
#49155=CARTESIAN_POINT('Ctrl Pts',(17.0158329838361,1.0164732758529,26.3060907914917));
#49156=CARTESIAN_POINT('Ctrl Pts',(17.0476605925309,0.985021085287657,26.8170996121502));
#49157=CARTESIAN_POINT('Ctrl Pts',(17.0794882012258,0.712451520320007,27.2504875294108));
#49158=CARTESIAN_POINT('Ctrl Pts',(17.1113158099206,0.265485244477138,27.5001681303059));
#49159=CARTESIAN_POINT('Ctrl Pts',(17.1431434186154,-0.246467567458505,
27.5050236006414));
#49160=CARTESIAN_POINT('Ctrl Pts',(17.1749710273102,-0.698089062672224,
27.2638654086669));
#49161=CARTESIAN_POINT('Ctrl Pts',(17.206798636005,-0.97882955717243,26.8357251963527));
#49162=CARTESIAN_POINT('Ctrl Pts',(17.2386262446998,-1.01996824129622,26.3254048593828));
#49163=CARTESIAN_POINT('Ctrl Pts',(17.2704538533946,-0.811435093319473,
25.8578225722776));
#49164=CARTESIAN_POINT('Ctrl Pts',(17.3022814620895,-0.404275555583194,
25.5474351058964));
#49165=CARTESIAN_POINT('Ctrl Pts',(17.3341090707843,0.101843998007599,25.4702201074962));
#49166=CARTESIAN_POINT('Ctrl Pts',(17.3659366794791,0.583034075919173,25.6450790044221));
#49167=CARTESIAN_POINT('Ctrl Pts',(17.3977642881739,0.921506185674827,26.0292083231239));
#49168=CARTESIAN_POINT('Ctrl Pts',(17.4295918968687,1.03440943041633,26.5285809084295));
#49169=CARTESIAN_POINT('Ctrl Pts',(17.4614195055636,0.894103789082602,27.0209554381429));
#49170=CARTESIAN_POINT('Ctrl Pts',(17.4932471142584,0.534939718203638,27.3858120280539));
#49171=CARTESIAN_POINT('Ctrl Pts',(17.5250747229532,0.0448237145771032,
27.5338292314391));
#49172=CARTESIAN_POINT('Ctrl Pts',(17.556902331648,-0.456250700141257,27.4287944496501));
#49173=CARTESIAN_POINT('Ctrl Pts',(17.5887299403428,-0.845668154601334,
27.096381428918));
#49174=CARTESIAN_POINT('Ctrl Pts',(17.6205575490376,-1.02803069848662,26.6180295723256));
#49175=CARTESIAN_POINT('Ctrl Pts',(17.6523851577325,-0.958840139662527,
26.1106995285693));
#49176=CARTESIAN_POINT('Ctrl Pts',(17.6842127664273,-0.654766539896501,
25.6988272140803));
#49177=CARTESIAN_POINT('Ctrl Pts',(17.7160403751221,-0.190745755648998,
25.4827609916589));
#49178=CARTESIAN_POINT('Ctrl Pts',(17.7478679838169,0.320587858023884,25.5162803182649));
#49179=CARTESIAN_POINT('Ctrl Pts',(17.7796955925117,0.752275258385287,25.7895010885325));
#49180=CARTESIAN_POINT('Ctrl Pts',(17.8115232012066,1.00201539234692,26.2387037897642));
#49181=CARTESIAN_POINT('Ctrl Pts',(17.8433508099014,1.00244486581897,26.7480441021986));
#49182=CARTESIAN_POINT('Ctrl Pts',(17.8857876214945,0.684775665170146,27.3550858372652));
#49183=CARTESIAN_POINT('Ctrl Pts',(17.9388336359858,-0.201818282340762,
27.6563391975183));
#49184=CARTESIAN_POINT('Ctrl Pts',(17.9918796504772,-0.933946851652724,
27.0725668336436));
#49185=CARTESIAN_POINT('Ctrl Pts',(18.0343164620703,-1.02720218653396,26.3938055857297));
#49186=CARTESIAN_POINT('Ctrl Pts',(18.0661440707651,-0.854261376904684,
25.9147239489671));
#49187=CARTESIAN_POINT('Ctrl Pts',(18.0979716794599,-0.467120983511694,
25.5766773292406));
#49188=CARTESIAN_POINT('Ctrl Pts',(18.1297992881547,0.0315965154626858,
25.4658420588924));
#49189=CARTESIAN_POINT('Ctrl Pts',(18.1616268968495,0.524053608104702,25.6075164095507));
#49190=CARTESIAN_POINT('Ctrl Pts',(18.1934545055444,0.887449122107085,25.9679933173937));
#49191=CARTESIAN_POINT('Ctrl Pts',(18.2252821142392,1.03402541318104,26.4585184935185));
#49192=CARTESIAN_POINT('Ctrl Pts',(18.257109722934,0.927269533067888,26.9592921837113));
#49193=CARTESIAN_POINT('Ctrl Pts',(18.2889373316288,0.593649090550186,27.3475884577754));
#49194=CARTESIAN_POINT('Ctrl Pts',(18.3207649403236,0.114651348604825,27.528435170219));
#49195=CARTESIAN_POINT('Ctrl Pts',(18.3525925490184,-0.392378625981908,
27.45752339869));
#49196=CARTESIAN_POINT('Ctrl Pts',(18.3844201577133,-0.803377856520256,
27.1522326814947));
#49197=CARTESIAN_POINT('Ctrl Pts',(18.416247766408,-1.01771392660482,26.6872819205827));
#49198=CARTESIAN_POINT('Ctrl Pts',(18.4480753751029,-0.982934779259867,
26.1764896326511));
#49199=CARTESIAN_POINT('Ctrl Pts',(18.4799029837977,-0.707546389749453,
25.7448863929147));
#49200=CARTESIAN_POINT('Ctrl Pts',(18.5117305924926,-0.258963342224468,
25.4981234458543));
#49201=CARTESIAN_POINT('Ctrl Pts',(18.5435582011873,0.253010499600352,25.496603511055));
#49202=CARTESIAN_POINT('Ctrl Pts',(18.5753858098822,0.703051045743631,25.7406991180043));
#49203=CARTESIAN_POINT('Ctrl Pts',(18.607213418577,0.980996166272481,26.1706593236401));
#49204=CARTESIAN_POINT('Ctrl Pts',(18.6390410272718,1.01880904226803,26.6812368940723));
#49205=CARTESIAN_POINT('Ctrl Pts',(18.6708686359666,0.807233851103414,27.1474505533964));
#49206=CARTESIAN_POINT('Ctrl Pts',(18.7026962446614,0.398060721868608,27.4551787077222));
#49207=CARTESIAN_POINT('Ctrl Pts',(18.7345238533562,-0.108551275958736,
27.5290944175065));
#49208=CARTESIAN_POINT('Ctrl Pts',(18.7663514620511,-0.58859166973049,27.351104312196));
#49209=CARTESIAN_POINT('Ctrl Pts',(18.7981790707459,-0.924554252459608,
26.9647775111451));
#49210=CARTESIAN_POINT('Ctrl Pts',(18.8300066794407,-1.03420077562692,26.4646806260004));
#49211=CARTESIAN_POINT('Ctrl Pts',(18.8618342881355,-0.890691524210388,
25.9732293569615));
#49212=CARTESIAN_POINT('Ctrl Pts',(18.8936618968303,-0.529155264648254,
25.6107230983562));
#49213=CARTESIAN_POINT('Ctrl Pts',(18.9254895055251,-0.038090277438839,
25.4658975714764));
#49214=CARTESIAN_POINT('Ctrl Pts',(18.95731711422,0.462298598977743,25.5742037442178));
#49215=CARTESIAN_POINT('Ctrl Pts',(18.9891447229147,0.849524188348949,25.9091300013411));
#49216=CARTESIAN_POINT('Ctrl Pts',(19.0209723316096,1.02879987283589,26.3886917634842));
#49217=CARTESIAN_POINT('Ctrl Pts',(19.0527999403044,0.956241838450062,26.8954999978265));
#49218=CARTESIAN_POINT('Ctrl Pts',(19.0846275489993,0.649611128981037,27.3054961719217));
#49219=CARTESIAN_POINT('Ctrl Pts',(19.116455157694,0.183966027343174,27.518319793906));
#49220=CARTESIAN_POINT('Ctrl Pts',(19.1482827663889,-0.326711009119531,
27.4818750523353));
#49221=CARTESIAN_POINT('Ctrl Pts',(19.1801103750837,-0.757414427187756,
27.2050830357943));
#49222=CARTESIAN_POINT('Ctrl Pts',(19.2119379837785,-1.00271493358913,26.7556979934127));
#49223=CARTESIAN_POINT('Ctrl Pts',(19.2437655924733,-1.00256689611852,26.2437221806618));
#49224=CARTESIAN_POINT('Ctrl Pts',(19.2755932011681,-0.757006551976856,
25.7944790703729));
#49225=CARTESIAN_POINT('Ctrl Pts',(19.307420809863,-0.326143137481079,25.5179361753167));
#49226=CARTESIAN_POINT('Ctrl Pts',(19.3392484185578,0.184554889531876,25.481786763675));
#49227=CARTESIAN_POINT('Ctrl Pts',(19.3710760272526,0.650076837698819,25.694879632002));
#49228=CARTESIAN_POINT('Ctrl Pts',(19.4029036359474,0.956470395659613,26.1050530616598));
#49229=CARTESIAN_POINT('Ctrl Pts',(19.4347312446422,1.0287353314103,26.6119031714732));
#49230=CARTESIAN_POINT('Ctrl Pts',(19.466558853337,0.849182346967171,27.0913611785339));
#49231=CARTESIAN_POINT('Ctrl Pts',(19.4983864620319,0.46176313498287,27.4260634476365));
#49232=CARTESIAN_POINT('Ctrl Pts',(19.5302140707267,-0.038688291141642,
27.5340802280318));
#49233=CARTESIAN_POINT('Ctrl Pts',(19.5620416794215,-0.529669443704362,
27.3889707432101));
#49234=CARTESIAN_POINT('Ctrl Pts',(19.5938692881163,-0.890996006178292,
27.0262554691896));
#49235=CARTESIAN_POINT('Ctrl Pts',(19.6256968968112,-1.03422102754035,26.5347212913211));
#49236=CARTESIAN_POINT('Ctrl Pts',(19.6575245055059,-0.924285318222643,
26.0346878978624));
#49237=CARTESIAN_POINT('Ctrl Pts',(19.6893521142008,-0.588099377777535,
25.6485554488193));
#49238=CARTESIAN_POINT('Ctrl Pts',(19.7211797228956,-0.10795613591828,25.4708429786494));
#49239=CARTESIAN_POINT('Ctrl Pts',(19.7530073315904,0.398613037654465,25.5450516516117));
#49240=CARTESIAN_POINT('Ctrl Pts',(19.7848349402852,0.8076081287208,25.853016374008));
#49241=CARTESIAN_POINT('Ctrl Pts',(19.8166625489801,1.01891369450633,26.3193523179637));
#49242=CARTESIAN_POINT('Ctrl Pts',(19.8484901576748,0.980805519387458,26.8299079189967));
#49243=CARTESIAN_POINT('Ctrl Pts',(19.8803177663697,0.702611873821896,27.2597073493406));
#49244=CARTESIAN_POINT('Ctrl Pts',(19.9121453750645,0.252430103257493,27.5035425974252));
#49245=CARTESIAN_POINT('Ctrl Pts',(19.9439729837593,-0.259542510544956,
27.5017267027975));
#49246=CARTESIAN_POINT('Ctrl Pts',(19.9758005924541,-0.70798327780557,27.2547041673565));
#49247=CARTESIAN_POINT('Ctrl Pts',(20.0076282011489,-0.983121086466923,
26.8229421484132));
#49248=CARTESIAN_POINT('Ctrl Pts',(20.0394558098438,-1.01760661097527,26.3121290677698));
#49249=CARTESIAN_POINT('Ctrl Pts',(20.0712834185386,-0.802998347677216,
25.8473037800743));
#49250=CARTESIAN_POINT('Ctrl Pts',(20.1031110272334,-0.391828959610619,
25.5422480653697));
#49251=CARTESIAN_POINT('Ctrl Pts',(20.1349386359282,0.115253877394866,25.4716346730743));
#49252=CARTESIAN_POINT('Ctrl Pts',(20.1667662446231,0.594124412544197,25.6527486298054));
#49253=CARTESIAN_POINT('Ctrl Pts',(20.1985938533178,0.927562814339893,26.0412561419142));
#49254=CARTESIAN_POINT('Ctrl Pts',(20.2304214620127,1.03394870649155,26.5420567975728));
#49255=CARTESIAN_POINT('Ctrl Pts',(20.2622490707075,0.887240527791323,27.0325626232869));
#49256=CARTESIAN_POINT('Ctrl Pts',(20.2940766794023,0.523350088894221,27.3927056549233));
#49257=CARTESIAN_POINT('Ctrl Pts',(20.3259042880971,0.0313519366769965,
27.534328650838));
#49258=CARTESIAN_POINT('Ctrl Pts',(20.3577318967919,-0.468320667118775,
27.4227645716146));
#49259=CARTESIAN_POINT('Ctrl Pts',(20.3895595054867,-0.853355878013929,
27.0853225156584));
#49260=CARTESIAN_POINT('Ctrl Pts',(20.4213871141815,-1.0295032478625,26.6046028896263));
#49261=CARTESIAN_POINT('Ctrl Pts',(20.4532147228764,-0.953644723878202,
26.098278152826));
#49262=CARTESIAN_POINT('Ctrl Pts',(20.4850423315712,-0.644349256845004,
25.6902884852733));
#49263=CARTESIAN_POINT('Ctrl Pts',(20.516869940266,-0.177327419594983,25.4805032181819));
#49264=CARTESIAN_POINT('Ctrl Pts',(20.5486975489608,0.333101327705005,25.5202744224229));
#49265=CARTESIAN_POINT('Ctrl Pts',(20.5805251576557,0.761992209049242,25.7998667446651));
#49266=CARTESIAN_POINT('Ctrl Pts',(20.6123527663505,1.0043596111001,26.2508404658286));
#49267=CARTESIAN_POINT('Ctrl Pts',(20.6441803750453,1.00087587858637,26.7628044473398));
#49268=CARTESIAN_POINT('Ctrl Pts',(20.6760079837401,0.752393773388913,27.2104381124652));
#49269=CARTESIAN_POINT('Ctrl Pts',(20.7078355924349,0.319737732100598,27.4841679148137));
#49270=CARTESIAN_POINT('Ctrl Pts',(20.7396632011297,-0.191184981135965,
27.5169891862088));
#49271=CARTESIAN_POINT('Ctrl Pts',(20.7714908098246,-0.655308675371252,
27.300867805484));
#49272=CARTESIAN_POINT('Ctrl Pts',(20.8033184185194,-0.959023309395961,
26.8887068225705));
#49273=CARTESIAN_POINT('Ctrl Pts',(20.8351460272142,-1.02798440884689,26.3813966398228));
#49274=CARTESIAN_POINT('Ctrl Pts',(20.866973635909,-0.84531140191147,25.9031186586296));
#49275=CARTESIAN_POINT('Ctrl Pts',(20.8988012446038,-0.45571971273963,25.5709476627777));
#49276=CARTESIAN_POINT('Ctrl Pts',(20.9306288532986,0.0454248576733852,
25.4661937878969));
#49277=CARTESIAN_POINT('Ctrl Pts',(20.9624564619935,0.535450151013717,25.6144991035256));
#49278=CARTESIAN_POINT('Ctrl Pts',(20.9942840706883,0.894405829771168,25.9795608454882));
#49279=CARTESIAN_POINT('Ctrl Pts',(21.0261116793831,1.03442529725508,26.4720177506916));
#49280=CARTESIAN_POINT('Ctrl Pts',(21.0579392880779,0.921234032107172,26.9713242620163));
#49281=CARTESIAN_POINT('Ctrl Pts',(21.0897668967727,0.582539441765831,27.3552581485521));
#49282=CARTESIAN_POINT('Ctrl Pts',(21.1215945054676,0.101248533229376,27.5298385487039));
#49283=CARTESIAN_POINT('Ctrl Pts',(21.1534221141624,-0.404826393394172,
27.4523309787512));
#49284=CARTESIAN_POINT('Ctrl Pts',(21.1852497228572,-0.811806307616102,
27.1417080494994));
#49285=CARTESIAN_POINT('Ctrl Pts',(21.217077331552,-1.02006904965355,26.6740052752549));
#49286=CARTESIAN_POINT('Ctrl Pts',(21.2489049402468,-0.978635238364995,
26.1637087986463));
#49287=CARTESIAN_POINT('Ctrl Pts',(21.2807325489416,-0.697647206638017,
25.7357310179343));
#49288=CARTESIAN_POINT('Ctrl Pts',(21.3125601576365,-0.245886320863374,
25.4948340340571));
#49289=CARTESIAN_POINT('Ctrl Pts',(21.3443877663313,0.266063595105304,25.4999855674855));
#49290=CARTESIAN_POINT('Ctrl Pts',(21.3762153750261,0.712885407554046,25.7499246054068));
#49291=CARTESIAN_POINT('Ctrl Pts',(21.4080429837209,0.985204298614172,26.1834700774496));
#49292=CARTESIAN_POINT('Ctrl Pts',(21.4398705924157,1.01636096857812,26.6944970010786));
#49293=CARTESIAN_POINT('Ctrl Pts',(21.4716982011106,0.79872876402887,27.1579141763107));
#49294=CARTESIAN_POINT('Ctrl Pts',(21.5035258098053,0.385580560353784,27.460284506464));
#49295=CARTESIAN_POINT('Ctrl Pts',(21.5353534185002,-0.121951584273673,
27.5275925812163));
#49296=CARTESIAN_POINT('Ctrl Pts',(21.567181027195,-0.599631935754259,27.3433624627058));
#49297=CARTESIAN_POINT('Ctrl Pts',(21.5990086358898,-0.930532000475933,
26.9526907310382));
#49298=CARTESIAN_POINT('Ctrl Pts',(21.6308362445846,-1.03365274637864,26.4512075643002));
#49299=CARTESIAN_POINT('Ctrl Pts',(21.6626638532794,-0.883751867721363,
25.9616680037592));
#49300=CARTESIAN_POINT('Ctrl Pts',(21.6944914619742,-0.517522696934846,
25.6039034873213));
#49301=CARTESIAN_POINT('Ctrl Pts',(21.7263190706691,-0.024612264976355,
25.4654890342339));
#49302=CARTESIAN_POINT('Ctrl Pts',(21.7581466793639,0.47432285495422,25.5803062840566));
#49303=CARTESIAN_POINT('Ctrl Pts',(21.7899742880587,0.857151342607267,25.9202498143647));
#49304=CARTESIAN_POINT('Ctrl Pts',(21.8218018967535,1.03016292031633,26.4021068976742));
#49305=CARTESIAN_POINT('Ctrl Pts',(21.8536295054483,0.951007126949275,26.9079266433678));
#49306=CARTESIAN_POINT('Ctrl Pts',(21.8854571141432,0.639060031985187,27.313892485158));
#49307=CARTESIAN_POINT('Ctrl Pts',(21.917284722838,0.170681284272388,27.5206304919396));
#49308=CARTESIAN_POINT('Ctrl Pts',(21.9491123315328,-0.339477506090018,
27.4775345133224));
#49309=CARTESIAN_POINT('Ctrl Pts',(21.9809399402276,-0.766537644227681,
27.1951537541145));
#49310=CARTESIAN_POINT('Ctrl Pts',(22.0127675489225,-1.00596165339614,26.7426104980707));
#49311=CARTESIAN_POINT('Ctrl Pts',(22.0445951576172,-0.999142373724045,
26.2306800807465));
#49312=CARTESIAN_POINT('Ctrl Pts',(22.0764227663121,-0.74774905557329,25.7846748629002));
#49313=CARTESIAN_POINT('Ctrl Pts',(22.1082503750069,-0.313318753805751,
25.5137697731304));
#49314=CARTESIAN_POINT('Ctrl Pts',(22.1400779837017,0.19780695690913,25.4842780352498));
#49315=CARTESIAN_POINT('Ctrl Pts',(22.1719055923965,0.660512695092847,25.7034187539875));
#49316=CARTESIAN_POINT('Ctrl Pts',(22.2037332010913,0.961535512449999,26.1175497938618));
#49317=CARTESIAN_POINT('Ctrl Pts',(22.2355608097862,1.02718984819223,26.625298514151));
#49318=CARTESIAN_POINT('Ctrl Pts',(22.267388418481,0.841404573260887,27.102376166505));
#49319=CARTESIAN_POINT('Ctrl Pts',(22.2992160271758,0.449656945126742,27.4320017883979));
#49320=CARTESIAN_POINT('Ctrl Pts',(22.3310436358706,-0.0521594959131353,
27.5334883109468));
#49321=CARTESIAN_POINT('Ctrl Pts',(22.3628712445654,-0.541208128384414,
27.3819934600938));
#49322=CARTESIAN_POINT('Ctrl Pts',(22.3946988532602,-0.897777685703373,
27.0146007471144));
#49323=CARTESIAN_POINT('Ctrl Pts',(22.426526461955,-1.03458565546189,26.521242019445));
#49324=CARTESIAN_POINT('Ctrl Pts',(22.4583540706499,-0.918143639469846,
26.0226835858901));
#49325=CARTESIAN_POINT('Ctrl Pts',(22.4901816793447,-0.576954776868062,
25.6409645599122));
#49326=CARTESIAN_POINT('Ctrl Pts',(22.5220092880395,-0.0945366325251403,
25.4695236407426));
#49327=CARTESIAN_POINT('Ctrl Pts',(22.5538368967343,0.4110225641932,25.5503268174779));
#49328=CARTESIAN_POINT('Ctrl Pts',(22.5856645054292,0.815970025212737,25.8635947675954));
#49329=CARTESIAN_POINT('Ctrl Pts',(22.6174921141239,1.0211811027177,26.3326445180763));
#49330=CARTESIAN_POINT('Ctrl Pts',(22.6493197228188,0.976423414130928,26.8426602080991));
#49331=CARTESIAN_POINT('Ctrl Pts',(22.6811473315136,0.692652924226338,27.2687981714588));
#49332=CARTESIAN_POINT('Ctrl Pts',(22.7129749402084,0.239332100558325,27.5067466650155));
#49333=CARTESIAN_POINT('Ctrl Pts',(22.7448025489032,-0.272573385226417,
27.4982597114699));
#49334=CARTESIAN_POINT('Ctrl Pts',(22.7766301575981,-0.717757275210811,
27.2454147810176));
#49335=CARTESIAN_POINT('Ctrl Pts',(22.8084577662928,-0.987245688692236,
26.8101042599453));
#49336=CARTESIAN_POINT('Ctrl Pts',(22.8402853749877,-1.01507218150648,26.2988851864996));
#49337=CARTESIAN_POINT('Ctrl Pts',(22.8721129836825,-0.794425274225543,
25.8368957958591));
#49338=CARTESIAN_POINT('Ctrl Pts',(22.9039405923773,-0.379315793144767,
25.5372236859226));
#49339=CARTESIAN_POINT('Ctrl Pts',(22.9357682010721,0.128644114289536,25.4732237859512));
#49340=CARTESIAN_POINT('Ctrl Pts',(22.967595809767,0.605114004499334,25.6605622456451));
#49341=CARTESIAN_POINT('Ctrl Pts',(22.9994234184617,0.933461685389972,26.0533816127984));
#49342=CARTESIAN_POINT('Ctrl Pts',(23.0312510271566,1.03331290755272,26.5555260025805));
#49343=CARTESIAN_POINT('Ctrl Pts',(23.0630786358514,0.880225692253004,27.0440785169214));
#49344=CARTESIAN_POINT('Ctrl Pts',(23.0949062445462,0.511673336059915,27.3994493310037));
#49345=CARTESIAN_POINT('Ctrl Pts',(23.126733853241,0.0178715484813904,27.5346493655498));
#49346=CARTESIAN_POINT('Ctrl Pts',(23.1585614619359,-0.480304907713853,
27.4165838191369));
#49347=CARTESIAN_POINT('Ctrl Pts',(23.1903890706307,-0.860910420998461,
27.0741532451305));
#49348=CARTESIAN_POINT('Ctrl Pts',(23.2222166793255,-1.03077886220077,26.5911791594484));
#49349=CARTESIAN_POINT('Ctrl Pts',(23.2540442880203,-0.948329159626196,
26.0858858769852));
#49350=CARTESIAN_POINT('Ctrl Pts',(23.2858718967151,-0.63374367893186,25.6819610942678));
#49351=CARTESIAN_POINT('Ctrl Pts',(23.31769950541,-0.16402790350388,25.4782791238554));
#49352=CARTESIAN_POINT('Ctrl Pts',(23.3495271141047,0.345839273604333,25.5246980474179));
#49353=CARTESIAN_POINT('Ctrl Pts',(23.3813547227996,0.771050539768965,25.8098552564863));
#49354=CARTESIAN_POINT('Ctrl Pts',(23.4131823314944,1.00752099247019,26.2639488368816));
#49355=CARTESIAN_POINT('Ctrl Pts',(23.4450099401892,0.997366455119157,26.7758239584965));
#49356=CARTESIAN_POINT('Ctrl Pts',(23.476837548884,0.743072595698879,27.2201817960758));
#49357=CARTESIAN_POINT('Ctrl Pts',(23.5086651575788,0.306886475083116,27.4882506733054));
#49358=CARTESIAN_POINT('Ctrl Pts',(23.5404927662737,-0.204420535747526,
27.5144116257429));
#49359=CARTESIAN_POINT('Ctrl Pts',(23.5723203749685,-0.665688675952158,
27.2922608715484));
#49360=CARTESIAN_POINT('Ctrl Pts',(23.6041479836633,-0.964006898178333,
26.8761773546377));
#49361=CARTESIAN_POINT('Ctrl Pts',(23.6359755923581,-1.02635168317555,26.3680116508159));
#49362=CARTESIAN_POINT('Ctrl Pts',(23.6678032010529,-0.837462026860863,
25.8921545793183));
#49363=CARTESIAN_POINT('Ctrl Pts',(23.6996308097477,-0.44357508950957,25.5650883240412));
#49364=CARTESIAN_POINT('Ctrl Pts',(23.7314584184426,0.0588919199745167,
25.4668734619421));
#49365=CARTESIAN_POINT('Ctrl Pts',(23.7632860271374,0.54694313138947,25.6215514170406));
#49366=CARTESIAN_POINT('Ctrl Pts',(23.7951136358322,0.90111143083913,25.9912595051613));
#49367=CARTESIAN_POINT('Ctrl Pts',(23.826941244527,1.03470209535356,26.4854991121453));
#49368=CARTESIAN_POINT('Ctrl Pts',(23.8587688532218,0.915014271498275,26.9832883040506));
#49369=CARTESIAN_POINT('Ctrl Pts',(23.8905964619167,0.571345620154082,27.362776265441));
#49370=CARTESIAN_POINT('Ctrl Pts',(23.9224240706114,0.0878207187267834,
27.531070425936));
#49371=CARTESIAN_POINT('Ctrl Pts',(23.9542516793063,-0.417201287023148,
27.4469750725251));
#49372=CARTESIAN_POINT('Ctrl Pts',(23.9860792880011,-0.820099104760281,
27.1310753998129));
#49373=CARTESIAN_POINT('Ctrl Pts',(24.0179068966959,-1.02224980649195,26.6606985843273));
#49374=CARTESIAN_POINT('Ctrl Pts',(24.0497345053907,-0.974170140577519,
26.1509853311323));
#49375=CARTESIAN_POINT('Ctrl Pts',(24.0815621140856,-0.687629238594858,
25.7267052747451));
#49376=CARTESIAN_POINT('Ctrl Pts',(24.1133897227804,-0.232767720569937,
25.4917153724576));
#49377=CARTESIAN_POINT('Ctrl Pts',(24.1452173314752,0.279071604566762,25.5035373858483));
#49378=CARTESIAN_POINT('Ctrl Pts',(24.17704494017,0.722598673964357,25.7592774755263));
#49379=CARTESIAN_POINT('Ctrl Pts',(24.2088725488648,0.989245170043781,26.1963345666319));
#49380=CARTESIAN_POINT('Ctrl Pts',(24.2407001575596,1.01374030446957,26.7077240885684));
#49381=CARTESIAN_POINT('Ctrl Pts',(24.2725277662545,0.790088060951025,27.1682660830988));
#49382=CARTESIAN_POINT('Ctrl Pts',(24.3043553749492,0.373034923923842,27.465227251693));
#49383=CARTESIAN_POINT('Ctrl Pts',(24.3361829836441,-0.13533118334359,27.525916260078));
#49384=CARTESIAN_POINT('Ctrl Pts',(24.3680105923389,-0.610570386064801,
27.3354774117463));
#49385=CARTESIAN_POINT('Ctrl Pts',(24.3998382010337,-0.936351744716457,
26.9405270843479));
#49386=CARTESIAN_POINT('Ctrl Pts',(24.4316658097286,-1.03292920443998,26.4377427876258));
#49387=CARTESIAN_POINT('Ctrl Pts',(24.4634934184233,-0.876662151072909,
25.9501980586121));
#49388=CARTESIAN_POINT('Ctrl Pts',(24.4953210271182,-0.505802254575641,
25.5972360324294));
#49389=CARTESIAN_POINT('Ctrl Pts',(24.527148635813,-0.0111300733365206,
25.4652561556863));
#49390=CARTESIAN_POINT('Ctrl Pts',(24.5589762445079,0.486266571458613,25.5865649867891));
#49391=CARTESIAN_POINT('Ctrl Pts',(24.5908038532026,0.864632953614065,25.9314680682651));
#49392=CARTESIAN_POINT('Ctrl Pts',(24.6226314618975,1.031351047369,26.4155386539979));
#49393=CARTESIAN_POINT('Ctrl Pts',(24.6544590705922,0.945610935589058,26.9202840234556));
#49394=CARTESIAN_POINT('Ctrl Pts',(24.6862866792871,0.628400423364985,27.3221506004329));
#49395=CARTESIAN_POINT('Ctrl Pts',(24.7181142879819,0.157367559726439,27.5227678881464));
#49396=CARTESIAN_POINT('Ctrl Pts',(24.7499418966767,-0.352186360189988,
27.4730279901286));
#49397=CARTESIAN_POINT('Ctrl Pts',(24.7817695053715,-0.775530704100024,
27.1851064361658));
#49398=CARTESIAN_POINT('Ctrl Pts',(24.8135971140664,-1.00903756212806,26.7294818077589));
#49399=CARTESIAN_POINT('Ctrl Pts',(24.8454247227612,-0.995548198159715,
26.2176837110286));
#49400=CARTESIAN_POINT('Ctrl Pts',(24.877252331456,-0.73836459228214,25.7749921167727));
#49401=CARTESIAN_POINT('Ctrl Pts',(24.9090799401508,-0.300441168983939,
25.5097708316469));
#49402=CARTESIAN_POINT('Ctrl Pts',(24.9409075488456,0.211025436903717,25.486941775189));
#49403=CARTESIAN_POINT('Ctrl Pts',(24.9727351575404,0.670836398228031,25.7120931345076));
#49404=CARTESIAN_POINT('Ctrl Pts',(25.0045627662353,0.966437361670276,26.1301114656476));
#49405=CARTESIAN_POINT('Ctrl Pts',(25.0363903749301,1.02546994937707,26.6386725812921));
#49406=CARTESIAN_POINT('Ctrl Pts',(25.0682179836249,0.833483930073081,27.1132888717298));
#49407=CARTESIAN_POINT('Ctrl Pts',(25.1000455923197,0.437474404063782,27.4377818763799));
#49408=CARTESIAN_POINT('Ctrl Pts',(25.1318732010145,-0.0656218440651441,
27.5327209087934));
#49409=CARTESIAN_POINT('Ctrl Pts',(25.1637008097093,-0.552654916577154,
27.3748664155519));
#49410=CARTESIAN_POINT('Ctrl Pts',(25.1955284184042,-0.90440692366044,27.0028586464532));
#49411=CARTESIAN_POINT('Ctrl Pts',(25.227356027099,-1.03477461198718,26.5077591406996));
#49412=CARTESIAN_POINT('Ctrl Pts',(25.2591836357938,-0.911846061034622,
26.0107603216692));
#49413=CARTESIAN_POINT('Ctrl Pts',(25.2910112444886,-0.56571220973346,25.6335195341866));
#49414=CARTESIAN_POINT('Ctrl Pts',(25.3228388531834,-0.0811010769258508,
25.4683792764785));
#49415=CARTESIAN_POINT('Ctrl Pts',(25.3546664618783,0.423362299596309,25.5557632367048));
#49416=CARTESIAN_POINT('Ctrl Pts',(25.386494070573,0.824193370978722,25.8742812220235));
#49417=CARTESIAN_POINT('Ctrl Pts',(25.4183216792679,1.02327511560964,26.3459651349479));
#49418=CARTESIAN_POINT('Ctrl Pts',(25.4501492879627,0.971875513356643,26.8553543139117));
#49419=CARTESIAN_POINT('Ctrl Pts',(25.4819768966576,0.682576362999678,27.2777584525745));
#49420=CARTESIAN_POINT('Ctrl Pts',(25.5138045053523,0.226193459557492,27.5097797882372));
#49421=CARTESIAN_POINT('Ctrl Pts',(25.5456321140472,-0.285557977276429,
27.4946232168462));
#49422=CARTESIAN_POINT('Ctrl Pts',(25.5774597227419,-0.727409398295521,
27.2359988241503));
#49423=CARTESIAN_POINT('Ctrl Pts',(25.6092873314368,-0.991202657792454,
26.7972137161442));
#49424=CARTESIAN_POINT('Ctrl Pts',(25.6411149401316,-1.01236539400214,26.2856754542898));
#49425=CARTESIAN_POINT('Ctrl Pts',(25.6729425488264,-0.785717308327549,
25.8266004059235));
#49426=CARTESIAN_POINT('Ctrl Pts',(25.7047701575212,-0.366738219301859,
25.5323627847595));
#49427=CARTESIAN_POINT('Ctrl Pts',(25.7365977662161,0.142012507544223,25.4749872441391));
#49428=CARTESIAN_POINT('Ctrl Pts',(25.7684253749109,0.616000848872784,25.6685183971005));
#49429=CARTESIAN_POINT('Ctrl Pts',(25.8002529836057,0.93920205568446,26.0655829187618));
#49430=CARTESIAN_POINT('Ctrl Pts',(25.8320805923005,1.03250165349385,26.568985779688));
#49431=CARTESIAN_POINT('Ctrl Pts',(25.8639082009953,0.873061395142099,27.055502026023));
#49432=CARTESIAN_POINT('Ctrl Pts',(25.8957358096901,0.499909702299201,27.4060402829133));
#49433=CARTESIAN_POINT('Ctrl Pts',(25.927563418385,0.00438812460655832,
27.5347943957049));
#49434=CARTESIAN_POINT('Ctrl Pts',(25.9593910270797,-0.49220759101559,27.4102474362556));
#49435=CARTESIAN_POINT('Ctrl Pts',(25.9912186357746,-0.868318786396127,
27.0628864757224));
#49436=CARTESIAN_POINT('Ctrl Pts',(26.0230462444694,-1.03187944404665,26.5777399629291));
#49437=CARTESIAN_POINT('Ctrl Pts',(26.0548738531642,-0.942852584360126,
26.0735638874461));
#49438=CARTESIAN_POINT('Ctrl Pts',(26.086701461859,-0.623030465420126,25.6737726615066));
#49439=CARTESIAN_POINT('Ctrl Pts',(26.1185290705539,-0.150700586062053,
25.4762284103369));
#49440=CARTESIAN_POINT('Ctrl Pts',(26.1503566792486,0.35851859155766,25.5292874779674));
#49441=CARTESIAN_POINT('Ctrl Pts',(26.1821842879435,0.779977767383015,25.8199605755439));
#49442=CARTESIAN_POINT('Ctrl Pts',(26.2140118966383,1.01051163721584,26.2770980038405));
#49443=CARTESIAN_POINT('Ctrl Pts',(26.2458395053331,0.993687039496576,26.7887952855562));
#49444=CARTESIAN_POINT('Ctrl Pts',(26.2776671140279,0.733626454713128,27.2298057419935));
#49445=CARTESIAN_POINT('Ctrl Pts',(26.3094947227228,0.29398082464875,27.4921608151878));
#49446=CARTESIAN_POINT('Ctrl Pts',(26.3413223314176,-0.217617061428775,
27.5116709161353));
#49447=CARTESIAN_POINT('Ctrl Pts',(26.3731499401124,-0.675963838923886,
27.2835021616918));
#49448=CARTESIAN_POINT('Ctrl Pts',(26.4049775488072,-0.968810988626381,
26.8636171944324));
#49449=CARTESIAN_POINT('Ctrl Pts',(26.436805157502,-1.02457724546662,26.3545814743717));
#49450=CARTESIAN_POINT('Ctrl Pts',(26.4580235632986,-0.894453156519727,
26.0391661184899));
#49451=CARTESIAN_POINT('Ctrl Pts',(26.4686327661969,-0.795561429326952,
25.9065866261757));
#49452=CARTESIAN_POINT('Ctrl Pts',(26.0278332223638,-0.992541444115404,
26.5000219547962));
#49453=CARTESIAN_POINT('Ctrl Pts',(26.036846713316,-0.9924061168657,26.3595200944171));
#49454=CARTESIAN_POINT('Ctrl Pts',(26.0458602042683,-0.962278587565093,
26.2189620518872));
#49455=CARTESIAN_POINT('Ctrl Pts',(26.0548736952205,-0.904386170695536,
26.0909616053013));
#49456=CARTESIAN_POINT('Ctrl Pts',(26.0654828981188,-0.836244714727549,
25.9403004778764));
#49457=CARTESIAN_POINT('Ctrl Pts',(26.0760921010171,-0.729637405062499,
25.8070368150429));
#49458=CARTESIAN_POINT('Ctrl Pts',(26.0867013039153,-0.597612150423695,
25.7074809613184));
#49459=CARTESIAN_POINT('Ctrl Pts',(26.0973105068136,-0.465586895784892,
25.6079251075939));
#49460=CARTESIAN_POINT('Ctrl Pts',(26.1079197097119,-0.308143696172334,
25.5420770629784));
#49461=CARTESIAN_POINT('Ctrl Pts',(26.1185289126102,-0.144552283834306,
25.5179962133571));
#49462=CARTESIAN_POINT('Ctrl Pts',(26.1291381155085,0.0190391285036842,
25.4939153637357));
#49463=CARTESIAN_POINT('Ctrl Pts',(26.1397473184067,0.188778753567142,25.5116017091084));
#49464=CARTESIAN_POINT('Ctrl Pts',(26.150356521305,0.343891720351772,25.5688903692854));
#49465=CARTESIAN_POINT('Ctrl Pts',(26.1609657242032,0.499004687136437,25.6261790294623));
#49466=CARTESIAN_POINT('Ctrl Pts',(26.1715749271015,0.639490995642267,25.7230700044435));
#49467=CARTESIAN_POINT('Ctrl Pts',(26.1821841299998,0.748156438714674,25.8477050180672));
#49468=CARTESIAN_POINT('Ctrl Pts',(26.1927933328981,0.856821881787082,25.972340031691));
#49469=CARTESIAN_POINT('Ctrl Pts',(26.2034025357963,0.933666459426068,26.1247190839574));
#49470=CARTESIAN_POINT('Ctrl Pts',(26.2140117386946,0.969284650291061,26.2861914397263));
#49471=CARTESIAN_POINT('Ctrl Pts',(26.2246209415929,1.00490284115605,26.4476637954953));
#49472=CARTESIAN_POINT('Ctrl Pts',(26.2352301444912,0.999294645247054,26.6182294547669));
#49473=CARTESIAN_POINT('Ctrl Pts',(26.2458393473894,0.953147142237316,26.777013983489));
#49474=CARTESIAN_POINT('Ctrl Pts',(26.2564485502877,0.906999639227578,26.935798512211));
#49475=CARTESIAN_POINT('Ctrl Pts',(26.267057753186,0.820312829117102,27.0828019103836));
#49476=CARTESIAN_POINT('Ctrl Pts',(26.2776669560843,0.703695195902629,27.2000294290331));
#49477=CARTESIAN_POINT('Ctrl Pts',(26.2882761589825,0.587077562688156,27.3172569476826));
#49478=CARTESIAN_POINT('Ctrl Pts',(26.2988853618808,0.440529106369687,27.4047085868092));
#49479=CARTESIAN_POINT('Ctrl Pts',(26.3094945647791,0.281988614504523,27.4516860879325));
#49480=CARTESIAN_POINT('Ctrl Pts',(26.3201037676774,0.123448122639396,27.4986635890558));
#49481=CARTESIAN_POINT('Ctrl Pts',(26.3307129705756,-0.0470844047724203,
27.5051669521759));
#49482=CARTESIAN_POINT('Ctrl Pts',(26.3413221734739,-0.208741752691548,
27.4703905305806));
#49483=CARTESIAN_POINT('Ctrl Pts',(26.3467147823159,-0.290911436137823,
27.4527138360742));
#49484=CARTESIAN_POINT('Ctrl Pts',(26.352107391158,-0.370788090973951,27.4243719231966));
#49485=CARTESIAN_POINT('Ctrl Pts',(26.3575,-0.445914873067339,27.3865896766146));
#49486=CARTESIAN_POINT('',(9.6,-0.662189971174158,26.1181378955904));
#49487=CARTESIAN_POINT('Ctrl Pts',(9.6,-0.662189971174161,26.1181378955904));
#49488=CARTESIAN_POINT('Ctrl Pts',(9.6,-0.686801732918713,26.1409234509207));
#49489=CARTESIAN_POINT('Ctrl Pts',(9.6,-0.709791921105586,26.1653652554484));
#49490=CARTESIAN_POINT('Ctrl Pts',(9.6,-0.731095598422574,26.1911933292668));
#49491=CARTESIAN_POINT('Ctrl Pts',(9.6,-0.746587075514762,26.2099748291899));
#49492=CARTESIAN_POINT('Ctrl Pts',(9.6,-0.76118721574113,26.2294905658139));
#49493=CARTESIAN_POINT('Ctrl Pts',(9.6,-0.774872528490492,26.2496541439083));
#49494=CARTESIAN_POINT('Ctrl Pts',(9.6,-0.787306841273407,26.2679745317168));
#49495=CARTESIAN_POINT('Ctrl Pts',(9.6,-0.798986056598059,26.2868299650152));
#49496=CARTESIAN_POINT('Ctrl Pts',(9.6,-0.809890960914313,26.3061651627819));
#49497=CARTESIAN_POINT('Ctrl Pts',(9.6,-0.81424407823496,26.3138835601062));
#49498=CARTESIAN_POINT('Ctrl Pts',(9.6,-0.81847261504564,26.321676705201));
#49499=CARTESIAN_POINT('Ctrl Pts',(9.6,-0.822570170079064,26.3295304891797));
#49500=CARTESIAN_POINT('Ctrl Pts',(9.6,-0.839363102383987,26.3617175035373));
#49501=CARTESIAN_POINT('Ctrl Pts',(9.6,-0.853982926877251,26.3949649073311));
#49502=CARTESIAN_POINT('Ctrl Pts',(9.6,-0.866370885724305,26.4290078753479));
#49503=CARTESIAN_POINT('Ctrl Pts',(9.6,-0.868330245916886,26.4343923327224));
#49504=CARTESIAN_POINT('Ctrl Pts',(9.6,-0.8702337540175,26.4397967967659));
#49505=CARTESIAN_POINT('Ctrl Pts',(9.6,-0.872081151097179,26.4452203335801));
#49506=CARTESIAN_POINT('Ctrl Pts',(9.6,-0.88031761925099,26.4694007270337));
#49507=CARTESIAN_POINT('Ctrl Pts',(9.6,-0.887439277333979,26.4939594120755));
#49508=CARTESIAN_POINT('Ctrl Pts',(9.6,-0.893464100126309,26.5188184610355));
#49509=CARTESIAN_POINT('Ctrl Pts',(9.6,-0.896486584530233,26.531289547799));
#49510=CARTESIAN_POINT('Ctrl Pts',(9.6,-0.899232918726265,26.5438363937201));
#49511=CARTESIAN_POINT('Ctrl Pts',(9.6,-0.901704670785838,26.5564500650579));
#49512=CARTESIAN_POINT('Ctrl Pts',(9.6,-0.903275800885989,26.5644677457292));
#49513=CARTESIAN_POINT('Ctrl Pts',(9.6,-0.904735366145582,26.5725097265233));
#49514=CARTESIAN_POINT('Ctrl Pts',(9.6,-0.90608264699377,26.580564871723));
#49515=CARTESIAN_POINT('Ctrl Pts',(9.6,-0.912493287483545,26.6188929159742));
#49516=CARTESIAN_POINT('Ctrl Pts',(9.6,-0.916374828360992,26.6575700845772));
#49517=CARTESIAN_POINT('Ctrl Pts',(9.6,-0.917813576717061,26.6963221410477));
#49518=CARTESIAN_POINT('Ctrl Pts',(9.6,-0.919296030516451,26.7362513844811));
#49519=CARTESIAN_POINT('Ctrl Pts',(9.6,-0.918185813702954,26.776260957008));
#49520=CARTESIAN_POINT('Ctrl Pts',(9.6,-0.914542375176316,26.816094610719));
#49521=CARTESIAN_POINT('Ctrl Pts',(9.6,-0.911350401534987,26.8509924062365));
#49522=CARTESIAN_POINT('Ctrl Pts',(9.6,-0.90621378911242,26.8857563520486));
#49523=CARTESIAN_POINT('Ctrl Pts',(9.6,-0.899144830704795,26.9202318686355));
#49524=CARTESIAN_POINT('Ctrl Pts',(9.59999999999996,-0.662189971174005,
26.1181378955905));
#49525=CARTESIAN_POINT('Ctrl Pts',(9.60084086971211,-0.657153163178387,
26.1093900202931));
#49526=CARTESIAN_POINT('Ctrl Pts',(9.61229094232253,-0.586182178363583,
25.9916516862185));
#49527=CARTESIAN_POINT('Ctrl Pts',(9.63435021783122,-0.387770113791111,
25.8037814721796));
#49528=CARTESIAN_POINT('Ctrl Pts',(9.66617782652605,-0.00653957363242062,
25.7030919772491));
#49529=CARTESIAN_POINT('Ctrl Pts',(9.69800543522088,0.376272204290504,25.7974986628543));
#49530=CARTESIAN_POINT('Ctrl Pts',(9.72983304391567,0.66698890097209,26.0638527475773));
#49531=CARTESIAN_POINT('Ctrl Pts',(9.76166065261051,0.794431941545588,26.4369759237776));
#49532=CARTESIAN_POINT('Ctrl Pts',(9.79348826130532,0.727413669545738,26.8255225525671));
#49533=CARTESIAN_POINT('Ctrl Pts',(9.82531587000014,0.482334658244354,27.1343885069846));
#49534=CARTESIAN_POINT('Ctrl Pts',(9.85714347869494,0.119188665110999,27.2879652485877));
#49535=CARTESIAN_POINT('Ctrl Pts',(9.88897108738978,-0.273133232602854,
27.2486612961868));
#49536=CARTESIAN_POINT('Ctrl Pts',(9.92079869608458,-0.598596265249733,
27.0260967569105));
#49537=CARTESIAN_POINT('Ctrl Pts',(9.94670853832486,-0.744262673060946,
26.740078447277));
#49538=CARTESIAN_POINT('Ctrl Pts',(9.96200917766685,-0.764304859829967,
26.5563460400826));
#49539=CARTESIAN_POINT('Ctrl Pts',(9.96670061411058,-0.764287395473808,
26.5000068045578));
#49540=CARTESIAN_POINT('Origin',(8.83329938588935,0.,26.5));
#49541=CARTESIAN_POINT('Origin',(9.6,0.,26.5));
#49542=CARTESIAN_POINT('Origin',(18.,0.,26.5));
#49543=CARTESIAN_POINT('Origin',(3.12167427535308,0.,26.5));
#49544=CARTESIAN_POINT('',(3.24334855070616,0.,26.5));
#49545=CARTESIAN_POINT('',(3.12167427535308,-2.4799097682734E-17,26.2975));
#49546=CARTESIAN_POINT('Origin',(2.25,-0.25,27.2));
#49547=CARTESIAN_POINT('',(3.75,-0.25,27.4682458365519));
#49548=CARTESIAN_POINT('',(2.25,-0.25,27.4682458365519));
#49549=CARTESIAN_POINT('',(5.1,-0.25,27.4682458365519));
#49550=CARTESIAN_POINT('',(3.75,-0.25,27.2));
#49551=CARTESIAN_POINT('',(3.75,-0.25,27.2));
#49552=CARTESIAN_POINT('',(2.25,-0.25,27.2));
#49553=CARTESIAN_POINT('',(2.25,-0.25,27.2));
#49554=CARTESIAN_POINT('',(2.25,-0.25,27.2));
#49555=CARTESIAN_POINT('Origin',(2.25,0.,27.2));
#49556=CARTESIAN_POINT('',(2.25,0.25,27.4682458365519));
#49557=CARTESIAN_POINT('Ctrl Pts',(2.25,-0.25,27.4682458365519));
#49558=CARTESIAN_POINT('Ctrl Pts',(2.2184626473304,-0.25,27.4682458365519));
#49559=CARTESIAN_POINT('Ctrl Pts',(2.18491957299737,-0.243669763522489,
27.4699471586642));
#49560=CARTESIAN_POINT('Ctrl Pts',(2.12336732874239,-0.218115996279034,
27.4760111944473));
#49561=CARTESIAN_POINT('Ctrl Pts',(2.09534588636318,-0.198899276956455,
27.4802776512909));
#49562=CARTESIAN_POINT('Ctrl Pts',(2.05110381617461,-0.154657206767882,
27.4882237616694));
#49563=CARTESIAN_POINT('Ctrl Pts',(2.03188468517318,-0.126634476150511,
27.4924312594508));
#49564=CARTESIAN_POINT('Ctrl Pts',(2.00632915724249,-0.0650776639541235,
27.4983591502449));
#49565=CARTESIAN_POINT('Ctrl Pts',(2.,-0.0315329431858092,27.5));
#49566=CARTESIAN_POINT('Ctrl Pts',(2.,0.0315329431858092,27.5));
#49567=CARTESIAN_POINT('Ctrl Pts',(2.00632915724249,0.065077663954124,27.4983591502449));
#49568=CARTESIAN_POINT('Ctrl Pts',(2.03188468517318,0.126634476150511,27.4924312594508));
#49569=CARTESIAN_POINT('Ctrl Pts',(2.05110381617461,0.154657206767882,27.4882237616694));
#49570=CARTESIAN_POINT('Ctrl Pts',(2.09534588636318,0.198899276956455,27.4802776512909));
#49571=CARTESIAN_POINT('Ctrl Pts',(2.12336732874239,0.218115996279034,27.4760111944473));
#49572=CARTESIAN_POINT('Ctrl Pts',(2.18491957299737,0.243669763522489,27.4699471586642));
#49573=CARTESIAN_POINT('Ctrl Pts',(2.2184626473304,0.25,27.4682458365519));
#49574=CARTESIAN_POINT('Ctrl Pts',(2.25,0.25,27.4682458365519));
#49575=CARTESIAN_POINT('',(2.25,0.25,27.2));
#49576=CARTESIAN_POINT('Origin',(2.25,0.,27.2));
#49577=CARTESIAN_POINT('',(2.25,0.25,27.2));
#49578=CARTESIAN_POINT('Origin',(3.75,0.25,27.2));
#49579=CARTESIAN_POINT('',(3.75,0.25,27.4682458365519));
#49580=CARTESIAN_POINT('',(5.1,0.25,27.4682458365519));
#49581=CARTESIAN_POINT('',(3.75,0.25,27.2));
#49582=CARTESIAN_POINT('',(3.75,0.25,27.2));
#49583=CARTESIAN_POINT('',(3.75,0.25,27.2));
#49584=CARTESIAN_POINT('Origin',(3.75,0.,27.2));
#49585=CARTESIAN_POINT('Ctrl Pts',(3.75,0.25,27.4682458365519));
#49586=CARTESIAN_POINT('Ctrl Pts',(3.7815373526696,0.25,27.4682458365519));
#49587=CARTESIAN_POINT('Ctrl Pts',(3.81508042700262,0.243669763522489,27.4699471586642));
#49588=CARTESIAN_POINT('Ctrl Pts',(3.87663267125761,0.218115996279034,27.4760111944473));
#49589=CARTESIAN_POINT('Ctrl Pts',(3.90465411363682,0.198899276956455,27.4802776512909));
#49590=CARTESIAN_POINT('Ctrl Pts',(3.94889618382539,0.154657206767882,27.4882237616694));
#49591=CARTESIAN_POINT('Ctrl Pts',(3.96811531482682,0.126634476150511,27.4924312594508));
#49592=CARTESIAN_POINT('Ctrl Pts',(3.99367084275751,0.065077663954124,27.4983591502449));
#49593=CARTESIAN_POINT('Ctrl Pts',(4.,0.0315329431858092,27.5));
#49594=CARTESIAN_POINT('Ctrl Pts',(4.,-0.0315329431858091,27.5));
#49595=CARTESIAN_POINT('Ctrl Pts',(3.99367084275751,-0.0650776639541237,
27.4983591502449));
#49596=CARTESIAN_POINT('Ctrl Pts',(3.96811531482682,-0.126634476150511,
27.4924312594508));
#49597=CARTESIAN_POINT('Ctrl Pts',(3.94889618382539,-0.154657206767882,
27.4882237616694));
#49598=CARTESIAN_POINT('Ctrl Pts',(3.90465411363682,-0.198899276956454,
27.4802776512909));
#49599=CARTESIAN_POINT('Ctrl Pts',(3.87663267125761,-0.218115996279034,
27.4760111944473));
#49600=CARTESIAN_POINT('Ctrl Pts',(3.81508042700263,-0.243669763522489,
27.4699471586642));
#49601=CARTESIAN_POINT('Ctrl Pts',(3.7815373526696,-0.25,27.4682458365519));
#49602=CARTESIAN_POINT('Ctrl Pts',(3.75,-0.25,27.4682458365519));
#49603=CARTESIAN_POINT('Origin',(3.75,0.,27.2));
#49604=CARTESIAN_POINT('Origin',(3.,0.,27.2));
#49605=CARTESIAN_POINT('Origin',(1.375,0.,26.5));
#49606=CARTESIAN_POINT('',(1.4,-0.999999999999999,26.5));
#49607=CARTESIAN_POINT('Origin',(1.4,0.,26.5));
#49608=CARTESIAN_POINT('',(1.375,-0.975,26.5));
#49609=CARTESIAN_POINT('Origin',(5.1,0.,26.5));
#49610=CARTESIAN_POINT('',(8.8,-1.,26.5));
#49611=CARTESIAN_POINT('Origin',(8.8,0.,26.5));
#49612=CARTESIAN_POINT('',(5.1,-1.,26.5));
#49613=CARTESIAN_POINT('Origin',(8.8,1.55,26.5));
#49614=CARTESIAN_POINT('',(8.8,-1.55,26.5));
#49615=CARTESIAN_POINT('Origin',(8.8,0.,26.5));
#49616=CARTESIAN_POINT('Origin',(8.825,0.,26.5));
#49617=CARTESIAN_POINT('',(8.85,-1.6,26.5));
#49618=CARTESIAN_POINT('Origin',(8.85,0.,26.5));
#49619=CARTESIAN_POINT('',(8.825,-1.575,26.5));
#49620=CARTESIAN_POINT('Origin',(9.2,0.,26.5));
#49621=CARTESIAN_POINT('',(9.55,-1.6,26.5));
#49622=CARTESIAN_POINT('Origin',(9.55,0.,26.5));
#49623=CARTESIAN_POINT('',(9.2,-1.6,26.5));
#49624=CARTESIAN_POINT('Origin',(9.575,0.,26.5));
#49625=CARTESIAN_POINT('',(9.6,-1.55,26.5));
#49626=CARTESIAN_POINT('Origin',(9.6,0.,26.5));
#49627=CARTESIAN_POINT('',(9.575,-1.575,26.5));
#49628=CARTESIAN_POINT('Origin',(9.6,1.,26.5));
#76622=UNCERTAINTY_MEASURE_WITH_UNIT(LENGTH_MEASURE(0.001),#76661,
'DISTANCE_ACCURACY_VALUE',
'Maximum model space distance between geometric entities at asserted c
onnectivities');
#76638=UNCERTAINTY_MEASURE_WITH_UNIT(LENGTH_MEASURE(0.001),#76661,
'DISTANCE_ACCURACY_VALUE',
'Maximum model space distance between geometric entities at asserted c
onnectivities');
#76644=(
GEOMETRIC_REPRESENTATION_CONTEXT(3)
GLOBAL_UNCERTAINTY_ASSIGNED_CONTEXT((#76622))
GLOBAL_UNIT_ASSIGNED_CONTEXT((#76661,#76663,#76664))
REPRESENTATION_CONTEXT('','3D')
);
#76660=(
GEOMETRIC_REPRESENTATION_CONTEXT(3)
GLOBAL_UNCERTAINTY_ASSIGNED_CONTEXT((#76638))
GLOBAL_UNIT_ASSIGNED_CONTEXT((#76661,#76663,#76664))
REPRESENTATION_CONTEXT('','3D')
);
#76661=(
LENGTH_UNIT()
NAMED_UNIT(*)
SI_UNIT(.CENTI.,.METRE.)
);
#76663=(
NAMED_UNIT(*)
PLANE_ANGLE_UNIT()
SI_UNIT($,.RADIAN.)
);
#76664=(
NAMED_UNIT(*)
SI_UNIT($,.STERADIAN.)
SOLID_ANGLE_UNIT()
);
#76670=SHAPE_DEFINITION_REPRESENTATION(#76691,#76740);
#76691=PRODUCT_DEFINITION_SHAPE('',$,#76762);
#76740=SHAPE_REPRESENTATION('',(#27589),#76644);
#76756=PRODUCT_DEFINITION_CONTEXT('part definition',#76821,'design');
#76762=PRODUCT_DEFINITION('2026-10-26-11-12-44-958',
'05_Quill_Feed_Lead_Screw_Tr20x4',#76783,#76756);
#76783=PRODUCT_DEFINITION_FORMATION('',$,#76828);
#76821=APPLICATION_CONTEXT(
'Core Data for Automotive Mechanical Design Process');
#76822=PRODUCT_CONTEXT('part definition',#76821,'mechanical');
#76828=PRODUCT('2026-10-26-11-12-44-958',
'05_Quill_Feed_Lead_Screw_Tr20x4',$,(#76822));
#76907=COLOUR_RGB('Black',0.12,0.14,0.17);
#76908=FILL_AREA_STYLE_COLOUR('',#76907);
#76909=FILL_AREA_STYLE('',(#76908));
#76910=SURFACE_STYLE_FILL_AREA(#76909);
#76911=SURFACE_SIDE_STYLE('',(#76910));
#76912=SURFACE_STYLE_USAGE(.BOTH.,#76911);
#76913=PRESENTATION_STYLE_ASSIGNMENT((#76912));
ENDSEC;
END-ISO-10303-21;
